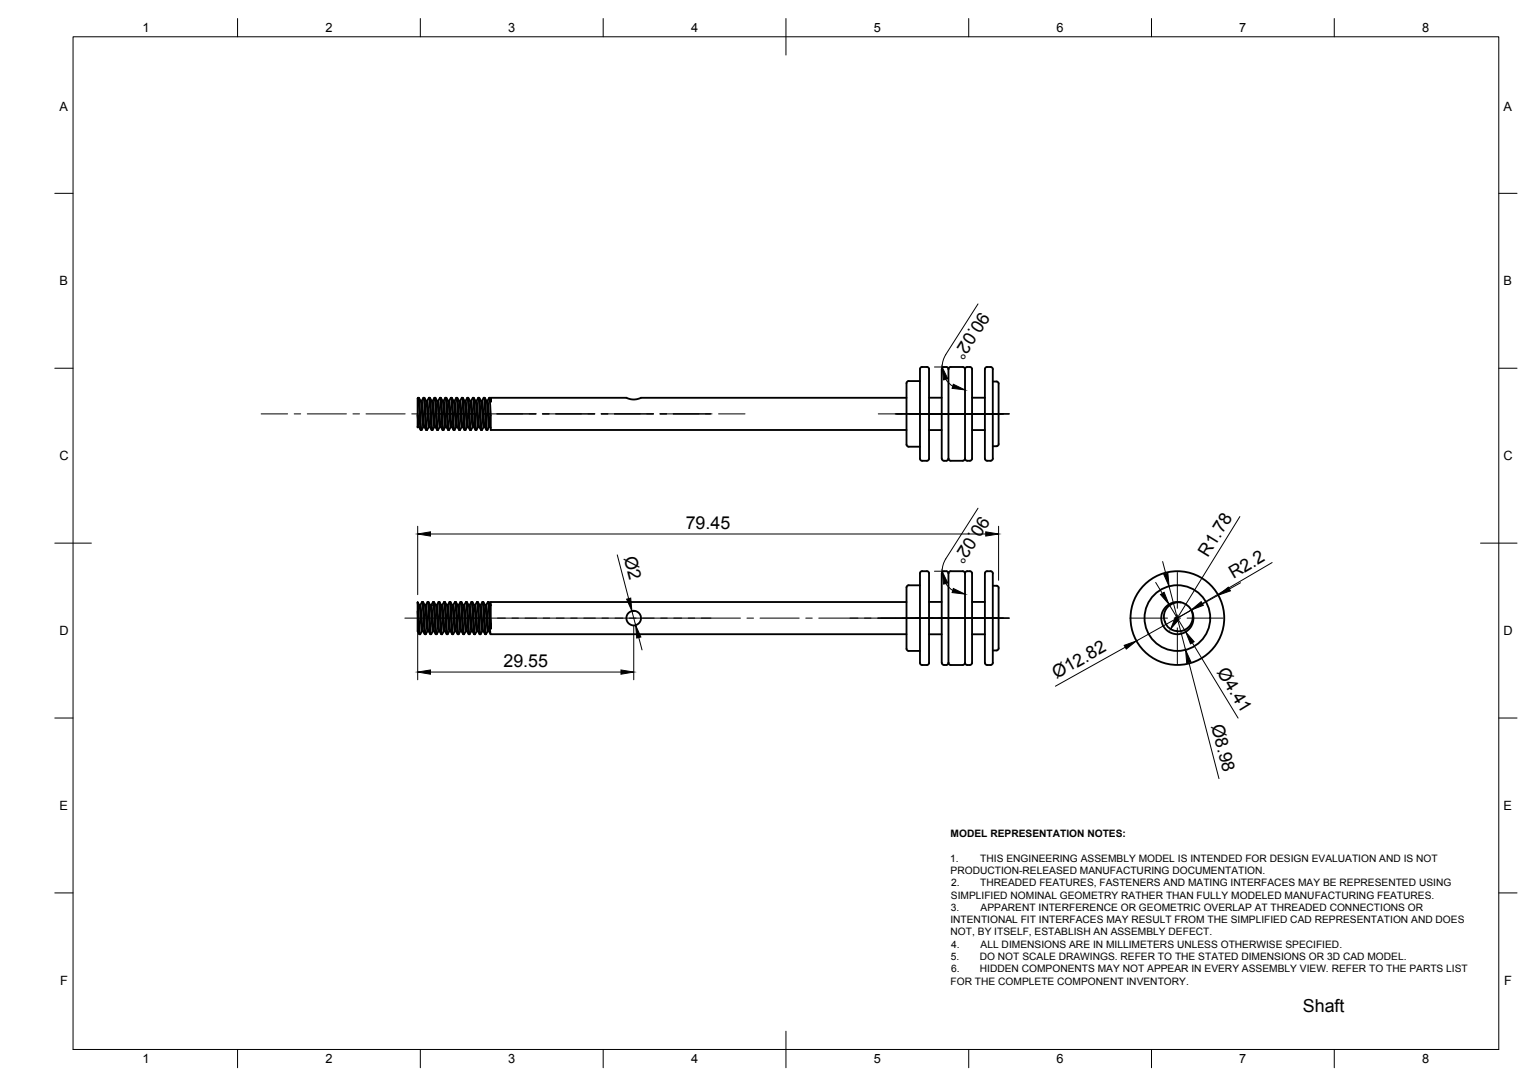
ISO-10303-21;
HEADER;
/* Generated by software containing ST-Developer
 * from STEP Tools, Inc. (www.steptools.com) 
 */

FILE_DESCRIPTION(
/* description */ (''),
/* implementation_level */ '2;1');

FILE_NAME(
/* name */ 'Shaft.step',
/* time_stamp */ '2026-10-06T13:15:55-07:00',
/* author */ (''),
/* organization */ (''),
/* preprocessor_version */ 'ST-DEVELOPER v20.2',
/* originating_system */ 'Autodesk Translation Framework v15.15.0.0',
/* authorisation */ '');

FILE_SCHEMA (('AUTOMOTIVE_DESIGN { 1 0 10303 214 3 1 1 }'));
ENDSEC;

DATA;
#10=MECHANICAL_DESIGN_GEOMETRIC_PRESENTATION_REPRESENTATION('',(#116),#27707);
#55=TOROIDAL_SURFACE('',#4197,6.10845002480549,0.3);
#56=TOROIDAL_SURFACE('',#4203,6.107959450045,0.3);
#57=TOROIDAL_SURFACE('',#4209,4.18902817623056,0.3);
#58=TOROIDAL_SURFACE('',#4216,6.1096023907077,0.3);
#59=TOROIDAL_SURFACE('',#4223,6.10941276264524,0.3);
#60=TOROIDAL_SURFACE('',#4228,6.1087216021292,0.3);
#61=TOROIDAL_SURFACE('',#4236,6.1086273903848,0.3);
#62=TOROIDAL_SURFACE('',#4238,6.10778208446569,0.3);
#63=TOROIDAL_SURFACE('',#4243,6.10767319978801,0.3);
#64=TOROIDAL_SURFACE('',#4248,6.1069775362949,0.3);
#65=TOROIDAL_SURFACE('',#4256,6.10683442041659,0.3);
#66=TOROIDAL_SURFACE('',#4261,4.12329516333974,0.3);
#83=CONICAL_SURFACE('',#4201,6.40820475053297,0.000295609290233083);
#84=CONICAL_SURFACE('',#4220,6.40950758978419,0.000295609290232241);
#85=CONICAL_SURFACE('',#4232,6.40867450936473,0.000295609290232273);
#86=CONICAL_SURFACE('',#4241,6.40772765523458,0.000295609290232245);
#87=CONICAL_SURFACE('',#4252,6.40690599146347,0.000295609290233429);
#96=SHAPE_REPRESENTATION_RELATIONSHIP('SRR','None',#27753,#106);
#106=ADVANCED_BREP_SHAPE_REPRESENTATION('',(#126),#27705);
#116=STYLED_ITEM('',(#27804),#126);
#126=MANIFOLD_SOLID_BREP('Body1',#3842);
#151=FACE_BOUND('',#835,.T.);
#152=FACE_BOUND('',#866,.T.);
#153=FACE_BOUND('',#871,.T.);
#154=FACE_BOUND('',#879,.T.);
#155=FACE_BOUND('',#883,.T.);
#156=FACE_BOUND('',#886,.T.);
#157=FACE_BOUND('',#890,.T.);
#158=FACE_BOUND('',#896,.T.);
#159=FACE_BOUND('',#900,.T.);
#160=FACE_BOUND('',#903,.T.);
#203=PLANE('',#4191);
#204=PLANE('',#4194);
#205=PLANE('',#4205);
#206=PLANE('',#4207);
#207=PLANE('',#4208);
#208=PLANE('',#4215);
#209=PLANE('',#4222);
#210=PLANE('',#4226);
#211=PLANE('',#4234);
#212=PLANE('',#4246);
#213=PLANE('',#4254);
#214=PLANE('',#4259);
#215=PLANE('',#4265);
#291=CIRCLE('',#4158,2.204);
#292=CIRCLE('',#4159,2.204);
#293=CIRCLE('',#4160,2.204);
#294=CIRCLE('',#4174,1.77625);
#295=CIRCLE('',#4188,1.77625);
#296=CIRCLE('',#4190,0.999999999999996);
#297=CIRCLE('',#4193,2.204);
#298=CIRCLE('',#4195,6.107959450045);
#299=CIRCLE('',#4196,6.10778208446569);
#300=CIRCLE('',#4198,6.10845002480549);
#301=CIRCLE('',#4199,0.3);
#302=CIRCLE('',#4200,6.40845001169777);
#303=CIRCLE('',#4202,6.40795943693727);
#304=CIRCLE('',#4204,0.3);
#305=CIRCLE('',#4206,6.1086273903848);
#306=CIRCLE('',#4210,4.18902817623056);
#307=CIRCLE('',#4211,0.3);
#308=CIRCLE('',#4212,4.48902817623056);
#309=CIRCLE('',#4214,4.48902817623056);
#310=CIRCLE('',#4217,6.1096023907077);
#311=CIRCLE('',#4218,0.3);
#312=CIRCLE('',#4219,6.40960237759997);
#313=CIRCLE('',#4221,6.40941274953751);
#314=CIRCLE('',#4224,0.3);
#315=CIRCLE('',#4225,6.10941276264524);
#316=CIRCLE('',#4227,2.21164758166987);
#317=CIRCLE('',#4229,6.1087216021292);
#318=CIRCLE('',#4230,0.3);
#319=CIRCLE('',#4231,6.40872158902147);
#320=CIRCLE('',#4233,6.40862737727707);
#321=CIRCLE('',#4235,2.21164758166987);
#322=CIRCLE('',#4237,0.3);
#323=CIRCLE('',#4239,0.3);
#324=CIRCLE('',#4240,6.40778207135796);
#325=CIRCLE('',#4242,6.40767318668028);
#326=CIRCLE('',#4244,0.3);
#327=CIRCLE('',#4245,6.10767319978801);
#328=CIRCLE('',#4247,2.21164758166987);
#329=CIRCLE('',#4249,6.1069775362949);
#330=CIRCLE('',#4250,0.3);
#331=CIRCLE('',#4251,6.40697752318717);
#332=CIRCLE('',#4253,6.40683440730886);
#333=CIRCLE('',#4255,2.21164758166987);
#334=CIRCLE('',#4257,0.3);
#335=CIRCLE('',#4258,6.10683442041659);
#336=CIRCLE('',#4260,4.42329516333974);
#337=CIRCLE('',#4262,4.42329516333974);
#338=CIRCLE('',#4263,0.3);
#339=CIRCLE('',#4264,4.12329516333974);
#403=CYLINDRICAL_SURFACE('',#4157,2.204);
#404=CYLINDRICAL_SURFACE('',#4161,2.204);
#405=CYLINDRICAL_SURFACE('',#4162,2.204);
#406=CYLINDRICAL_SURFACE('',#4163,2.204);
#407=CYLINDRICAL_SURFACE('',#4164,2.204);
#408=CYLINDRICAL_SURFACE('',#4165,2.204);
#409=CYLINDRICAL_SURFACE('',#4166,2.204);
#410=CYLINDRICAL_SURFACE('',#4167,2.204);
#411=CYLINDRICAL_SURFACE('',#4168,2.204);
#412=CYLINDRICAL_SURFACE('',#4169,2.204);
#413=CYLINDRICAL_SURFACE('',#4170,2.204);
#414=CYLINDRICAL_SURFACE('',#4171,2.204);
#415=CYLINDRICAL_SURFACE('',#4172,2.204);
#416=CYLINDRICAL_SURFACE('',#4173,1.77625);
#417=CYLINDRICAL_SURFACE('',#4175,1.77625);
#418=CYLINDRICAL_SURFACE('',#4176,1.77625);
#419=CYLINDRICAL_SURFACE('',#4177,1.77625);
#420=CYLINDRICAL_SURFACE('',#4178,1.77625);
#421=CYLINDRICAL_SURFACE('',#4179,1.77625);
#422=CYLINDRICAL_SURFACE('',#4180,1.77625);
#423=CYLINDRICAL_SURFACE('',#4181,1.77625);
#424=CYLINDRICAL_SURFACE('',#4182,1.77625);
#425=CYLINDRICAL_SURFACE('',#4183,1.77625);
#426=CYLINDRICAL_SURFACE('',#4184,1.77625);
#427=CYLINDRICAL_SURFACE('',#4185,1.77625);
#428=CYLINDRICAL_SURFACE('',#4186,1.77625);
#429=CYLINDRICAL_SURFACE('',#4187,1.77625);
#430=CYLINDRICAL_SURFACE('',#4189,0.999999999999996);
#431=CYLINDRICAL_SURFACE('',#4192,2.204);
#432=CYLINDRICAL_SURFACE('',#4213,4.48902817623056);
#433=CYLINDRICAL_SURFACE('',#4266,4.42329516333974);
#434=CYLINDRICAL_SURFACE('',#4267,2.21164758166987);
#435=CYLINDRICAL_SURFACE('',#4268,2.21164758166987);
#590=FACE_OUTER_BOUND('',#834,.T.);
#591=FACE_OUTER_BOUND('',#836,.T.);
#592=FACE_OUTER_BOUND('',#837,.T.);
#593=FACE_OUTER_BOUND('',#838,.T.);
#594=FACE_OUTER_BOUND('',#839,.T.);
#595=FACE_OUTER_BOUND('',#840,.T.);
#596=FACE_OUTER_BOUND('',#841,.T.);
#597=FACE_OUTER_BOUND('',#842,.T.);
#598=FACE_OUTER_BOUND('',#843,.T.);
#599=FACE_OUTER_BOUND('',#844,.T.);
#600=FACE_OUTER_BOUND('',#845,.T.);
#601=FACE_OUTER_BOUND('',#846,.T.);
#602=FACE_OUTER_BOUND('',#847,.T.);
#603=FACE_OUTER_BOUND('',#848,.T.);
#604=FACE_OUTER_BOUND('',#849,.T.);
#605=FACE_OUTER_BOUND('',#850,.T.);
#606=FACE_OUTER_BOUND('',#851,.T.);
#607=FACE_OUTER_BOUND('',#852,.T.);
#608=FACE_OUTER_BOUND('',#853,.T.);
#609=FACE_OUTER_BOUND('',#854,.T.);
#610=FACE_OUTER_BOUND('',#855,.T.);
#611=FACE_OUTER_BOUND('',#856,.T.);
#612=FACE_OUTER_BOUND('',#857,.T.);
#613=FACE_OUTER_BOUND('',#858,.T.);
#614=FACE_OUTER_BOUND('',#859,.T.);
#615=FACE_OUTER_BOUND('',#860,.T.);
#616=FACE_OUTER_BOUND('',#861,.T.);
#617=FACE_OUTER_BOUND('',#862,.T.);
#618=FACE_OUTER_BOUND('',#863,.T.);
#619=FACE_OUTER_BOUND('',#864,.T.);
#620=FACE_OUTER_BOUND('',#865,.T.);
#621=FACE_OUTER_BOUND('',#867,.T.);
#622=FACE_OUTER_BOUND('',#868,.T.);
#623=FACE_OUTER_BOUND('',#869,.T.);
#624=FACE_OUTER_BOUND('',#870,.T.);
#625=FACE_OUTER_BOUND('',#872,.T.);
#626=FACE_OUTER_BOUND('',#873,.T.);
#627=FACE_OUTER_BOUND('',#874,.T.);
#628=FACE_OUTER_BOUND('',#875,.T.);
#629=FACE_OUTER_BOUND('',#876,.T.);
#630=FACE_OUTER_BOUND('',#877,.T.);
#631=FACE_OUTER_BOUND('',#878,.T.);
#632=FACE_OUTER_BOUND('',#880,.T.);
#633=FACE_OUTER_BOUND('',#881,.T.);
#634=FACE_OUTER_BOUND('',#882,.T.);
#635=FACE_OUTER_BOUND('',#884,.T.);
#636=FACE_OUTER_BOUND('',#885,.T.);
#637=FACE_OUTER_BOUND('',#887,.T.);
#638=FACE_OUTER_BOUND('',#888,.T.);
#639=FACE_OUTER_BOUND('',#889,.T.);
#640=FACE_OUTER_BOUND('',#891,.T.);
#641=FACE_OUTER_BOUND('',#892,.T.);
#642=FACE_OUTER_BOUND('',#893,.T.);
#643=FACE_OUTER_BOUND('',#894,.T.);
#644=FACE_OUTER_BOUND('',#895,.T.);
#645=FACE_OUTER_BOUND('',#897,.T.);
#646=FACE_OUTER_BOUND('',#898,.T.);
#647=FACE_OUTER_BOUND('',#899,.T.);
#648=FACE_OUTER_BOUND('',#901,.T.);
#649=FACE_OUTER_BOUND('',#902,.T.);
#650=FACE_OUTER_BOUND('',#904,.T.);
#651=FACE_OUTER_BOUND('',#905,.T.);
#652=FACE_OUTER_BOUND('',#906,.T.);
#653=FACE_OUTER_BOUND('',#907,.T.);
#654=FACE_OUTER_BOUND('',#908,.T.);
#834=EDGE_LOOP('',(#3233,#3234,#3235,#3236,#3237,#3238,#3239,#3240,#3241,
#3242));
#835=EDGE_LOOP('',(#3243,#3244));
#836=EDGE_LOOP('',(#3245,#3246,#3247,#3248));
#837=EDGE_LOOP('',(#3249,#3250,#3251,#3252));
#838=EDGE_LOOP('',(#3253,#3254,#3255,#3256,#3257,#3258));
#839=EDGE_LOOP('',(#3259,#3260,#3261,#3262,#3263,#3264));
#840=EDGE_LOOP('',(#3265,#3266,#3267,#3268));
#841=EDGE_LOOP('',(#3269,#3270,#3271,#3272,#3273,#3274));
#842=EDGE_LOOP('',(#3275,#3276,#3277,#3278));
#843=EDGE_LOOP('',(#3279,#3280,#3281,#3282));
#844=EDGE_LOOP('',(#3283,#3284,#3285,#3286,#3287,#3288));
#845=EDGE_LOOP('',(#3289,#3290,#3291,#3292,#3293,#3294));
#846=EDGE_LOOP('',(#3295,#3296,#3297,#3298));
#847=EDGE_LOOP('',(#3299,#3300,#3301,#3302));
#848=EDGE_LOOP('',(#3303,#3304,#3305,#3306));
#849=EDGE_LOOP('',(#3307,#3308,#3309,#3310));
#850=EDGE_LOOP('',(#3311,#3312,#3313,#3314,#3315));
#851=EDGE_LOOP('',(#3316,#3317,#3318,#3319));
#852=EDGE_LOOP('',(#3320,#3321,#3322,#3323));
#853=EDGE_LOOP('',(#3324,#3325,#3326,#3327));
#854=EDGE_LOOP('',(#3328,#3329,#3330,#3331));
#855=EDGE_LOOP('',(#3332,#3333,#3334,#3335));
#856=EDGE_LOOP('',(#3336,#3337,#3338,#3339));
#857=EDGE_LOOP('',(#3340,#3341,#3342,#3343));
#858=EDGE_LOOP('',(#3344,#3345,#3346,#3347));
#859=EDGE_LOOP('',(#3348,#3349,#3350,#3351,#3352));
#860=EDGE_LOOP('',(#3353,#3354,#3355,#3356));
#861=EDGE_LOOP('',(#3357,#3358,#3359,#3360,#3361));
#862=EDGE_LOOP('',(#3362,#3363,#3364,#3365,#3366));
#863=EDGE_LOOP('',(#3367));
#864=EDGE_LOOP('',(#3368,#3369,#3370,#3371));
#865=EDGE_LOOP('',(#3372));
#866=EDGE_LOOP('',(#3373));
#867=EDGE_LOOP('',(#3374,#3375,#3376,#3377));
#868=EDGE_LOOP('',(#3378,#3379,#3380,#3381));
#869=EDGE_LOOP('',(#3382,#3383,#3384,#3385));
#870=EDGE_LOOP('',(#3386));
#871=EDGE_LOOP('',(#3387));
#872=EDGE_LOOP('',(#3388,#3389,#3390,#3391,#3392,#3393,#3394,#3395,#3396,
#3397,#3398,#3399,#3400,#3401,#3402,#3403,#3404,#3405,#3406,#3407,#3408,
#3409,#3410,#3411,#3412,#3413,#3414,#3415,#3416,#3417,#3418,#3419,#3420,
#3421,#3422,#3423,#3424,#3425));
#873=EDGE_LOOP('',(#3426,#3427,#3428,#3429,#3430,#3431));
#874=EDGE_LOOP('',(#3432,#3433,#3434,#3435,#3436,#3437,#3438,#3439,#3440,
#3441,#3442,#3443,#3444,#3445,#3446,#3447,#3448,#3449,#3450,#3451,#3452,
#3453,#3454,#3455,#3456,#3457,#3458,#3459,#3460,#3461,#3462,#3463,#3464,
#3465,#3466,#3467,#3468,#3469,#3470));
#875=EDGE_LOOP('',(#3471,#3472,#3473,#3474,#3475));
#876=EDGE_LOOP('',(#3476,#3477,#3478,#3479));
#877=EDGE_LOOP('',(#3480,#3481,#3482,#3483));
#878=EDGE_LOOP('',(#3484));
#879=EDGE_LOOP('',(#3485));
#880=EDGE_LOOP('',(#3486,#3487,#3488,#3489));
#881=EDGE_LOOP('',(#3490,#3491,#3492,#3493));
#882=EDGE_LOOP('',(#3494));
#883=EDGE_LOOP('',(#3495));
#884=EDGE_LOOP('',(#3496,#3497,#3498,#3499));
#885=EDGE_LOOP('',(#3500));
#886=EDGE_LOOP('',(#3501));
#887=EDGE_LOOP('',(#3502,#3503,#3504,#3505));
#888=EDGE_LOOP('',(#3506,#3507,#3508,#3509));
#889=EDGE_LOOP('',(#3510));
#890=EDGE_LOOP('',(#3511));
#891=EDGE_LOOP('',(#3512,#3513,#3514,#3515));
#892=EDGE_LOOP('',(#3516,#3517,#3518,#3519));
#893=EDGE_LOOP('',(#3520,#3521,#3522,#3523));
#894=EDGE_LOOP('',(#3524,#3525,#3526,#3527));
#895=EDGE_LOOP('',(#3528));
#896=EDGE_LOOP('',(#3529));
#897=EDGE_LOOP('',(#3530,#3531,#3532,#3533));
#898=EDGE_LOOP('',(#3534,#3535,#3536,#3537));
#899=EDGE_LOOP('',(#3538));
#900=EDGE_LOOP('',(#3539));
#901=EDGE_LOOP('',(#3540,#3541,#3542,#3543));
#902=EDGE_LOOP('',(#3544));
#903=EDGE_LOOP('',(#3545));
#904=EDGE_LOOP('',(#3546,#3547,#3548,#3549));
#905=EDGE_LOOP('',(#3550));
#906=EDGE_LOOP('',(#3551,#3552,#3553,#3554));
#907=EDGE_LOOP('',(#3555,#3556,#3557,#3558));
#908=EDGE_LOOP('',(#3559,#3560,#3561,#3562));
#1052=LINE('',#15722,#1228);
#1053=LINE('',#15863,#1229);
#1054=LINE('',#15978,#1230);
#1055=LINE('',#16402,#1231);
#1056=LINE('',#16802,#1232);
#1057=LINE('',#17236,#1233);
#1058=LINE('',#17648,#1234);
#1059=LINE('',#18052,#1235);
#1060=LINE('',#18470,#1236);
#1061=LINE('',#18872,#1237);
#1062=LINE('',#19296,#1238);
#1063=LINE('',#19720,#1239);
#1064=LINE('',#20146,#1240);
#1065=LINE('',#20554,#1241);
#1066=LINE('',#20960,#1242);
#1067=LINE('',#21259,#1243);
#1068=LINE('',#21635,#1244);
#1069=LINE('',#22036,#1245);
#1070=LINE('',#22418,#1246);
#1071=LINE('',#22804,#1247);
#1072=LINE('',#23196,#1248);
#1073=LINE('',#23578,#1249);
#1074=LINE('',#23968,#1250);
#1075=LINE('',#24346,#1251);
#1076=LINE('',#24732,#1252);
#1077=LINE('',#25116,#1253);
#1078=LINE('',#25507,#1254);
#1079=LINE('',#26142,#1255);
#1080=LINE('',#26496,#1256);
#1081=LINE('',#27575,#1257);
#1082=LINE('',#27586,#1258);
#1083=LINE('',#27604,#1259);
#1084=LINE('',#27617,#1260);
#1085=LINE('',#27634,#1261);
#1086=LINE('',#27654,#1262);
#1087=LINE('',#27656,#1263);
#1088=LINE('',#27658,#1264);
#1228=VECTOR('',#4831,2.204);
#1229=VECTOR('',#4834,2.204);
#1230=VECTOR('',#4841,2.204);
#1231=VECTOR('',#4844,2.204);
#1232=VECTOR('',#4847,2.204);
#1233=VECTOR('',#4850,2.204);
#1234=VECTOR('',#4853,2.204);
#1235=VECTOR('',#4856,2.204);
#1236=VECTOR('',#4859,2.204);
#1237=VECTOR('',#4862,2.204);
#1238=VECTOR('',#4865,2.204);
#1239=VECTOR('',#4868,2.204);
#1240=VECTOR('',#4871,2.204);
#1241=VECTOR('',#4874,2.204);
#1242=VECTOR('',#4877,1.77625);
#1243=VECTOR('',#4882,1.77625);
#1244=VECTOR('',#4885,1.77625);
#1245=VECTOR('',#4888,1.77625);
#1246=VECTOR('',#4891,1.77625);
#1247=VECTOR('',#4894,1.77625);
#1248=VECTOR('',#4897,1.77625);
#1249=VECTOR('',#4900,1.77625);
#1250=VECTOR('',#4903,1.77625);
#1251=VECTOR('',#4906,1.77625);
#1252=VECTOR('',#4909,1.77625);
#1253=VECTOR('',#4912,1.77625);
#1254=VECTOR('',#4915,1.77625);
#1255=VECTOR('',#4924,0.999999999999996);
#1256=VECTOR('',#4947,6.40820475053297);
#1257=VECTOR('',#4972,4.48902817623056);
#1258=VECTOR('',#4987,6.40950758978419);
#1259=VECTOR('',#5012,6.40867450936473);
#1260=VECTOR('',#5031,6.40772765523458);
#1261=VECTOR('',#5054,6.40690599146347);
#1262=VECTOR('',#5083,4.42329516333974);
#1263=VECTOR('',#5086,2.21164758166987);
#1264=VECTOR('',#5089,2.21164758166987);
#1442=B_SPLINE_CURVE_WITH_KNOTS('',3,(#15724,#15725,#15726,#15727),
 .UNSPECIFIED.,.F.,.F.,(4,4),(2.77524983164141,2.7754356884636),
 .UNSPECIFIED.);
#1443=B_SPLINE_CURVE_WITH_KNOTS('',3,(#15729,#15730,#15731,#15732,#15733,
#15734,#15735,#15736,#15737,#15738,#15739,#15740,#15741,#15742,#15743,#15744,
#15745,#15746,#15747,#15748,#15749,#15750,#15751,#15752,#15753,#15754,#15755,
#15756,#15757,#15758,#15759,#15760,#15761,#15762,#15763,#15764,#15765,#15766,
#15767,#15768,#15769,#15770,#15771,#15772,#15773,#15774,#15775,#15776,#15777,
#15778,#15779,#15780,#15781,#15782,#15783,#15784,#15785,#15786,#15787,#15788,
#15789,#15790,#15791,#15792,#15793,#15794,#15795,#15796,#15797,#15798,#15799,
#15800,#15801,#15802,#15803,#15804,#15805,#15806,#15807,#15808,#15809,#15810,
#15811,#15812,#15813,#15814,#15815,#15816,#15817,#15818,#15819,#15820,#15821,
#15822,#15823,#15824,#15825,#15826,#15827,#15828,#15829,#15830,#15831,#15832,
#15833,#15834,#15835,#15836,#15837,#15838,#15839,#15840,#15841,#15842,#15843,
#15844,#15845,#15846,#15847,#15848,#15849,#15850,#15851,#15852),
 .UNSPECIFIED.,.F.,.F.,(4,3,3,3,3,3,3,3,3,3,3,3,3,3,3,3,3,3,3,3,3,3,3,3,
3,3,3,3,3,3,3,3,3,3,3,3,3,3,3,3,3,4),(-5.2891562906822,-5.18360776201043,
-5.16592202403009,-5.06502794865638,-5.0409071101405,-4.991013367524,-4.99097352154249,
-4.89791297254004,-4.8887207823386,-4.78661873310371,-4.68463617498642,
-4.58271830049947,-4.48083193862712,-4.37894396049634,-4.27695022114797,
-4.17490252616154,-4.07267004030852,-3.9928178800891,-3.99277881723399,
-3.89952340746646,-3.89022667007414,-3.78782539108402,-3.68554527959923,
-3.58333102513057,-3.48114986928111,-3.37896909715953,-3.27668767666928,
-3.17435468887112,-3.0718440432757,-2.9946218545813,-2.99458411292549,-2.90179614365268,
-2.89325038855348,-2.79021171641803,-2.68914057287426,-2.58812832611143,
-2.48714069765389,-2.38259077610789,-2.28148996903811,-2.175215490254,-2.07915882623621,
-2.06894888197497),.UNSPECIFIED.);
#1444=B_SPLINE_CURVE_WITH_KNOTS('',3,(#15854,#15855,#15856,#15857,#15858,
#15859),.UNSPECIFIED.,.F.,.F.,(4,2,4),(0.000102523276221914,0.00211374109474727,
0.00412550342438516),.UNSPECIFIED.);
#1445=B_SPLINE_CURVE_WITH_KNOTS('',3,(#15867,#15868,#15869,#15870,#15871,
#15872,#15873,#15874,#15875,#15876,#15877,#15878,#15879,#15880,#15881,#15882,
#15883,#15884,#15885,#15886,#15887,#15888,#15889,#15890,#15891,#15892,#15893,
#15894,#15895,#15896,#15897,#15898,#15899,#15900,#15901,#15902,#15903,#15904,
#15905,#15906,#15907,#15908,#15909,#15910,#15911,#15912,#15913,#15914,#15915,
#15916,#15917,#15918,#15919,#15920,#15921,#15922,#15923,#15924,#15925,#15926,
#15927,#15928,#15929,#15930,#15931,#15932,#15933,#15934,#15935,#15936),
 .UNSPECIFIED.,.F.,.F.,(4,3,3,3,3,3,3,3,3,3,3,3,3,3,3,3,3,3,3,3,3,3,3,4),
(0.,0.104661171317195,0.209255039882458,0.313836025669164,0.418414672909222,
0.523017976486558,0.627672951902333,0.732486530385716,0.837386576506837,
0.942488701205836,0.998194704308485,1.09966450843524,1.20096987785232,1.30213869551464,
1.40323263958923,1.50428592829615,1.60533272568538,1.70647828415392,1.80767242300264,
1.9090522202859,1.99638940861699,2.12019797963207,2.24242280953419,2.31370279205594),
 .UNSPECIFIED.);
#1446=B_SPLINE_CURVE_WITH_KNOTS('',3,(#15939,#15940,#15941,#15942,#15943,
#15944,#15945,#15946,#15947,#15948),.UNSPECIFIED.,.F.,.F.,(4,2,2,2,4),(0.,
0.038320218022911,0.076640436045822,0.114893233564743,0.153146031083664),
 .UNSPECIFIED.);
#1447=B_SPLINE_CURVE_WITH_KNOTS('',3,(#15949,#15950,#15951,#15952,#15953,
#15954,#15955,#15956,#15957,#15958,#15959,#15960,#15961,#15962,#15963,#15964,
#15965,#15966,#15967,#15968,#15969,#15970,#15971,#15972,#15973,#15974),
 .UNSPECIFIED.,.F.,.F.,(4,2,2,2,2,2,2,2,2,2,2,2,4),(0.153146031083664,0.191398828602585,
0.229651626121507,0.267971844144418,0.306292062167329,0.344612280190239,
0.382932498213151,0.421185295732072,0.459438093250993,0.497690890769914,
0.535943688288835,0.574263906311746,0.612584124334657),.UNSPECIFIED.);
#1448=B_SPLINE_CURVE_WITH_KNOTS('',3,(#15979,#15980,#15981,#15982,#15983,
#15984,#15985,#15986,#15987,#15988,#15989,#15990,#15991,#15992,#15993,#15994,
#15995,#15996,#15997,#15998,#15999,#16000,#16001,#16002,#16003,#16004,#16005,
#16006,#16007,#16008,#16009,#16010,#16011,#16012,#16013,#16014,#16015,#16016,
#16017,#16018,#16019,#16020,#16021,#16022,#16023,#16024,#16025,#16026,#16027,
#16028,#16029,#16030,#16031,#16032,#16033,#16034,#16035,#16036,#16037,#16038,
#16039,#16040,#16041,#16042,#16043,#16044,#16045,#16046,#16047,#16048,#16049,
#16050,#16051,#16052,#16053,#16054,#16055,#16056,#16057,#16058,#16059,#16060,
#16061,#16062,#16063,#16064,#16065,#16066,#16067,#16068,#16069,#16070,#16071,
#16072,#16073,#16074,#16075,#16076,#16077,#16078,#16079,#16080,#16081,#16082,
#16083,#16084,#16085,#16086,#16087,#16088,#16089,#16090,#16091,#16092,#16093,
#16094,#16095,#16096,#16097,#16098,#16099,#16100,#16101,#16102,#16103,#16104,
#16105,#16106,#16107,#16108,#16109,#16110,#16111,#16112,#16113,#16114,#16115,
#16116,#16117,#16118,#16119,#16120,#16121,#16122,#16123,#16124,#16125,#16126,
#16127,#16128,#16129,#16130,#16131,#16132,#16133,#16134,#16135,#16136,#16137,
#16138,#16139,#16140,#16141,#16142,#16143,#16144,#16145,#16146,#16147,#16148,
#16149,#16150,#16151,#16152,#16153,#16154,#16155,#16156,#16157,#16158,#16159,
#16160,#16161,#16162,#16163,#16164,#16165,#16166,#16167,#16168,#16169,#16170,
#16171,#16172,#16173,#16174,#16175,#16176,#16177,#16178,#16179,#16180,#16181,
#16182,#16183,#16184,#16185,#16186,#16187,#16188),.UNSPECIFIED.,.F.,.F.,
(4,2,2,2,2,2,2,2,2,2,2,2,2,2,2,2,2,2,2,2,2,2,2,2,2,2,2,2,2,2,2,2,2,2,2,
2,2,2,2,2,2,2,2,2,2,2,2,2,2,2,2,2,2,2,2,2,2,2,2,2,2,2,2,2,2,2,2,2,2,2,2,
2,2,2,2,2,2,2,2,2,2,2,2,2,2,2,2,2,2,2,2,2,2,2,2,2,2,2,2,2,2,2,2,2,4),(1.38781753873472,
1.39967307302691,1.40445914459052,1.40800356043637,1.41188756410644,1.41730276084749,
1.43084058397849,1.45101472565709,1.49357630988404,1.51136965632633,1.51559250277158,
1.51800787610396,1.52016188469643,1.52312080974288,1.5301823492393,1.54050794057009,
1.57534931570515,1.61237651259864,1.62165050138927,1.62639272592381,1.63018049920159,
1.63449363382543,1.64197198759118,1.68827555501049,1.72888793290298,1.73432736841164,
1.73703730628583,1.73921644847553,1.74151957718618,1.74523007548616,1.75831706971953,
1.78424581384169,1.83324275090273,1.84148685272035,1.84640241907379,1.85021948989542,
1.85438844787025,1.86119275138631,1.88833036670492,1.91645593292796,1.92484579996025,
1.95163644192558,1.95615739428983,1.95866430015579,1.96080002902903,1.96360332353323,
1.96976113670856,1.9974795461816,2.04742308357646,2.06052975701291,2.06602236058527,
2.06988229338644,2.07387199386493,2.07982730521795,2.09743024198081,2.12751039769845,
2.16992979139149,2.17582030821991,2.17857371361266,2.18070399666525,2.18324296864977,
2.18805348663228,2.19427456685343,2.20908608355818,2.2374776975812,2.27704904795642,
2.2843724340021,2.28869178348119,2.29243957129668,2.29714655932481,2.30656346429877,
2.31888721665889,2.35133919106459,2.39005584916645,2.39615404619614,2.39891498336828,
2.40104980462189,2.40355070418799,2.40817287159305,2.44279419766279,2.49508899561064,
2.5030484745972,2.50793628306202,2.51174021856224,2.51596804476606,2.52304226080094,
2.55492153642243,2.59780879562011,2.6137871040324,2.61788971530304,2.62028035171697,
2.62244948790057,2.62547794183238,2.63293492193362,2.64405309222125,2.66962673554813,
2.70117621828321,2.71983292544932,2.72609634153291,2.73015451659309,2.73402583299897,
2.73784961158552,2.74298847368029,2.75426624309546,2.77524983164141),
 .UNSPECIFIED.);
#1449=B_SPLINE_CURVE_WITH_KNOTS('',3,(#16189,#16190,#16191,#16192,#16193,
#16194,#16195,#16196,#16197,#16198,#16199,#16200,#16201,#16202,#16203,#16204,
#16205,#16206,#16207,#16208,#16209,#16210,#16211,#16212,#16213,#16214,#16215,
#16216,#16217,#16218,#16219,#16220,#16221,#16222,#16223,#16224,#16225,#16226,
#16227,#16228,#16229,#16230,#16231,#16232,#16233,#16234,#16235,#16236,#16237,
#16238,#16239,#16240,#16241,#16242,#16243,#16244,#16245,#16246,#16247,#16248,
#16249,#16250,#16251,#16252,#16253,#16254,#16255,#16256,#16257,#16258,#16259,
#16260,#16261,#16262,#16263,#16264,#16265,#16266,#16267,#16268,#16269,#16270,
#16271,#16272,#16273,#16274,#16275,#16276,#16277,#16278,#16279,#16280,#16281,
#16282,#16283,#16284,#16285,#16286,#16287,#16288,#16289,#16290,#16291,#16292,
#16293,#16294,#16295,#16296,#16297,#16298,#16299,#16300,#16301,#16302,#16303,
#16304,#16305,#16306,#16307,#16308,#16309,#16310,#16311,#16312,#16313,#16314,
#16315,#16316,#16317,#16318,#16319,#16320,#16321,#16322,#16323,#16324,#16325,
#16326,#16327,#16328,#16329,#16330,#16331,#16332,#16333,#16334,#16335,#16336,
#16337,#16338,#16339,#16340,#16341,#16342,#16343,#16344,#16345,#16346,#16347,
#16348,#16349,#16350,#16351,#16352,#16353,#16354,#16355,#16356,#16357,#16358,
#16359,#16360,#16361,#16362,#16363,#16364,#16365,#16366,#16367,#16368,#16369,
#16370,#16371,#16372,#16373,#16374,#16375,#16376,#16377,#16378,#16379,#16380,
#16381,#16382,#16383,#16384,#16385,#16386,#16387,#16388,#16389,#16390,#16391,
#16392,#16393,#16394,#16395,#16396,#16397,#16398),.UNSPECIFIED.,.F.,.F.,
(4,2,2,2,2,2,2,2,2,2,2,2,2,2,2,2,2,2,2,2,2,2,2,2,2,2,2,2,2,2,2,2,2,2,2,
2,2,2,2,2,2,2,2,2,2,2,2,2,2,2,2,2,2,2,2,2,2,2,2,2,2,2,2,2,2,2,2,2,2,2,2,
2,2,2,2,2,2,2,2,2,2,2,2,2,2,2,2,2,2,2,2,2,2,2,2,2,2,2,2,2,2,2,2,2,4),(0.000677522696600237,
0.0305089258241106,0.0357217105988039,0.0396135137556909,0.0435607528904782,
0.0477204696182164,0.0541915833973012,0.0741059967373185,0.115440097777174,
0.134317184493834,0.145106172757179,0.14864706152995,0.150963559598939,
0.153001420155386,0.155815446427006,0.163035034986156,0.217821138578187,
0.238208395197482,0.251873813278667,0.257357570144765,0.26129934021213,
0.26538551201792,0.271602298038433,0.289353198948155,0.339589261144455,
0.361984375015146,0.367591576073439,0.370311762371205,0.372252757395784,
0.374772116565687,0.379314809039923,0.406404733718979,0.414432682325065,
0.443038327387056,0.460786979930571,0.473151978164989,0.478396583079974,
0.482262594137674,0.486356375416247,0.492760354432907,0.51259909284976,
0.556547787118553,0.582188012129803,0.588138338702213,0.590907459740892,
0.592847503273448,0.595324546479347,0.599646787124584,0.619687590510394,
0.660066375923141,0.680065489411854,0.693550325746206,0.698995403707921,
0.702919464612365,0.706513885714489,0.711389222317492,0.723711801320998,
0.774193276476291,0.802031745603604,0.808230933663737,0.81106284263699,
0.813204901215941,0.815740344409894,0.820315956534282,0.848389345799933,
0.876342856806042,0.909948384155844,0.917146197055969,0.921427871307066,
0.9252687321384,0.930189007400477,0.938172509254794,0.999164983852803,1.01692011627422,
1.02727200361296,1.03071451736817,1.03297461344143,1.03498700860256,1.03776741267351,
1.04344525041317,1.07678153395365,1.10750510753919,1.13160484949986,1.1382267514405,
1.14238168193455,1.14625250349466,1.15133390112501,1.16295108822414,1.2146743273094,
1.24296511256131,1.24920253029659,1.25203487369017,1.25419112323307,1.2567231961712,
1.26128999367794,1.28892807428539,1.29537580787022,1.32175712996296,1.34142706453204,
1.35474982493395,1.36016555562901,1.36408011350876,1.36767367219295,1.37350241506738,
1.38838504316647),.UNSPECIFIED.);
#1450=B_SPLINE_CURVE_WITH_KNOTS('',3,(#16403,#16404,#16405,#16406,#16407,
#16408,#16409,#16410,#16411,#16412,#16413,#16414,#16415,#16416,#16417,#16418,
#16419,#16420,#16421,#16422,#16423,#16424,#16425,#16426,#16427,#16428,#16429,
#16430,#16431,#16432,#16433,#16434,#16435,#16436,#16437,#16438,#16439,#16440,
#16441,#16442,#16443,#16444,#16445,#16446,#16447,#16448,#16449,#16450,#16451,
#16452,#16453,#16454,#16455,#16456,#16457,#16458,#16459,#16460,#16461,#16462,
#16463,#16464,#16465,#16466,#16467,#16468,#16469,#16470,#16471,#16472,#16473,
#16474,#16475,#16476,#16477,#16478,#16479,#16480,#16481,#16482,#16483,#16484,
#16485,#16486,#16487,#16488,#16489,#16490,#16491,#16492,#16493,#16494,#16495,
#16496,#16497,#16498,#16499,#16500,#16501,#16502,#16503,#16504,#16505,#16506,
#16507,#16508,#16509,#16510,#16511,#16512,#16513,#16514,#16515,#16516,#16517,
#16518,#16519,#16520,#16521,#16522,#16523,#16524,#16525,#16526,#16527,#16528,
#16529,#16530,#16531,#16532,#16533,#16534,#16535,#16536,#16537,#16538,#16539,
#16540,#16541,#16542,#16543,#16544,#16545,#16546,#16547,#16548,#16549,#16550,
#16551,#16552,#16553,#16554,#16555,#16556,#16557,#16558,#16559,#16560,#16561,
#16562,#16563,#16564,#16565,#16566,#16567,#16568,#16569,#16570,#16571,#16572,
#16573,#16574,#16575,#16576,#16577,#16578,#16579,#16580,#16581,#16582,#16583,
#16584,#16585,#16586,#16587,#16588,#16589,#16590,#16591,#16592,#16593,#16594,
#16595,#16596,#16597,#16598),.UNSPECIFIED.,.F.,.F.,(4,2,2,2,2,2,2,2,2,2,
2,2,2,2,2,2,2,2,2,2,2,2,2,2,2,2,2,2,2,2,2,2,2,2,2,2,2,2,2,2,2,2,2,2,2,2,
2,2,2,2,2,2,2,2,2,2,2,2,2,2,2,2,2,2,2,2,2,2,2,2,2,2,2,2,2,2,2,2,2,2,2,2,
2,2,2,2,2,2,2,2,2,2,2,2,2,2,2,4),(0.00029246168118835,0.0328585636678094,
0.0667058328462643,0.0778435259812811,0.0828696078886542,0.0866900014310973,
0.0908461587794147,0.097592177913589,0.121093785472563,0.162881838567066,
0.180219822071848,0.190388972658726,0.193788250972792,0.196023740153427,
0.198017167485471,0.200771856106451,0.206396616707088,0.238925364174105,
0.266963907016703,0.294244321785116,0.301057788663898,0.305228435652312,
0.309044486884806,0.313955159749232,0.32218284537282,0.37135389164148,0.408175613816101,
0.412996223661644,0.415538634251756,0.417669540176693,0.420421537274337,
0.426304777495165,0.468914542634666,0.513239590782438,0.520844568367973,
0.525184629927034,0.528969383857968,0.533672976813764,0.542760084971374,
0.590969748200195,0.628864181011441,0.63355354838131,0.636068557916207,
0.638202427997394,0.640945550577899,0.646939191710579,0.687873371930506,
0.733784327768257,0.741346096652906,0.745676995844228,0.749462733365603,
0.75417927556698,0.763328775599775,0.810387242799095,0.837579976993194,
0.851030621355834,0.85477432184903,0.857084664002877,0.859259266550924,
0.861951867948976,0.868744858537939,0.912920490817548,0.940791392600704,
0.957582742793873,0.963439773532905,0.967408607838282,0.971282412503524,
0.976854716010281,0.990459250029259,1.03990459175393,1.06745386194676,1.0735937358375,
1.07639297618157,1.07852766872987,1.08103585188433,1.08556365529159,1.11268366089787,
1.11969753011607,1.1461997886862,1.16583340621934,1.17911405711989,1.18449016762945,
1.18836697719528,1.1919190330671,1.19766366486624,1.21233214987857,1.26072984825734,
1.28791979545175,1.29402325910311,1.29681596339525,1.29895021111714,1.30146329140139,
1.30601243315762,1.33451743269651,1.34130110590104,1.37019173079264,1.38769992508917,
1.38781753873472),.UNSPECIFIED.);
#1451=B_SPLINE_CURVE_WITH_KNOTS('',3,(#16599,#16600,#16601,#16602,#16603,
#16604,#16605,#16606,#16607,#16608,#16609,#16610,#16611,#16612,#16613,#16614,
#16615,#16616,#16617,#16618,#16619,#16620,#16621,#16622,#16623,#16624,#16625,
#16626,#16627,#16628,#16629,#16630,#16631,#16632,#16633,#16634,#16635,#16636,
#16637,#16638,#16639,#16640,#16641,#16642,#16643,#16644,#16645,#16646,#16647,
#16648,#16649,#16650,#16651,#16652,#16653,#16654,#16655,#16656,#16657,#16658,
#16659,#16660,#16661,#16662,#16663,#16664,#16665,#16666,#16667,#16668,#16669,
#16670,#16671,#16672,#16673,#16674,#16675,#16676,#16677,#16678,#16679,#16680,
#16681,#16682,#16683,#16684,#16685,#16686,#16687,#16688,#16689,#16690,#16691,
#16692,#16693,#16694,#16695,#16696,#16697,#16698,#16699,#16700,#16701,#16702,
#16703,#16704,#16705,#16706,#16707,#16708,#16709,#16710,#16711,#16712,#16713,
#16714,#16715,#16716,#16717,#16718,#16719,#16720,#16721,#16722,#16723,#16724,
#16725,#16726,#16727,#16728,#16729,#16730,#16731,#16732,#16733,#16734,#16735,
#16736,#16737,#16738,#16739,#16740,#16741,#16742,#16743,#16744,#16745,#16746,
#16747,#16748,#16749,#16750,#16751,#16752,#16753,#16754,#16755,#16756,#16757,
#16758,#16759,#16760,#16761,#16762,#16763,#16764,#16765,#16766,#16767,#16768,
#16769,#16770,#16771,#16772,#16773,#16774,#16775,#16776,#16777,#16778,#16779,
#16780,#16781,#16782,#16783,#16784,#16785,#16786,#16787,#16788,#16789,#16790,
#16791,#16792,#16793,#16794,#16795,#16796,#16797,#16798),.UNSPECIFIED.,
 .F.,.F.,(4,2,2,2,2,2,2,2,2,2,2,2,2,2,2,2,2,2,2,2,2,2,2,2,2,2,2,2,2,2,2,
2,2,2,2,2,2,2,2,2,2,2,2,2,2,2,2,2,2,2,2,2,2,2,2,2,2,2,2,2,2,2,2,2,2,2,2,
2,2,2,2,2,2,2,2,2,2,2,2,2,2,2,2,2,2,2,2,2,2,2,2,2,2,2,2,2,2,2,2,4),(1.38838504316647,
1.38850331657018,1.41256316811428,1.44667306241606,1.44811102723475,1.46649225057238,
1.47078026121916,1.47322547472784,1.47540162643616,1.4783881126609,1.48550725028072,
1.49592014500493,1.53121036702826,1.57078963891295,1.57821322467278,1.58258414872904,
1.58637316595498,1.59112839135375,1.60063468496618,1.61307917518895,1.64597237337316,
1.68389210018361,1.69005705102998,1.69284763421741,1.69500521915381,1.69753462282851,
1.70222009150174,1.70821798458257,1.75324208371746,1.79131622025913,1.79870369069099,
1.80306600069939,1.80685518199548,1.8116205870635,1.82118240752868,1.83372301547411,
1.86708290252621,1.90429856815899,1.91048908900112,1.91328403539824,1.9154419261792,
1.91796812267015,1.92263817328133,1.95937186695389,2.00891986627212,2.0171489199126,
2.02208526843446,2.02593676625895,2.03016270781747,2.03710709121351,2.06580112389977,
2.10529365796466,2.11401940909033,2.12837645384582,2.13235851468054,2.13473615847624,
2.13693609000036,2.14007345763307,2.14815486371714,2.16055820080493,2.2141235386633,
2.23416610497521,2.24061215811045,2.24473120291012,2.2486205794772,2.25389698809855,
2.26634447371481,2.28422675209128,2.31266795024048,2.32187714503914,2.34769990694516,
2.35222491717066,2.35474724607128,2.35688492438732,2.3597205397784,2.36597037686206,
2.39437673715468,2.44646960400029,2.45758228102903,2.46265717510102,2.46652855117249,
2.47068950817631,2.47733309926365,2.5016848784883,2.56327049652331,2.57095989607791,
2.57412270183141,2.57630528481707,2.57866621813506,2.58257291008395,2.59766209358923,
2.6311708372892,2.66962264116428,2.67899573405107,2.68378599503464,2.68761203478231,
2.6919694937766,2.69952942370826,2.74493413473101,2.77590460384327),
 .UNSPECIFIED.);
#1452=B_SPLINE_CURVE_WITH_KNOTS('',3,(#16804,#16805,#16806,#16807,#16808,
#16809,#16810,#16811,#16812,#16813,#16814,#16815,#16816,#16817,#16818,#16819,
#16820,#16821,#16822,#16823,#16824,#16825,#16826,#16827,#16828,#16829,#16830,
#16831,#16832,#16833,#16834,#16835,#16836,#16837,#16838,#16839,#16840,#16841,
#16842,#16843,#16844,#16845,#16846,#16847,#16848,#16849,#16850,#16851,#16852,
#16853,#16854,#16855,#16856,#16857,#16858,#16859,#16860,#16861,#16862,#16863,
#16864,#16865,#16866,#16867,#16868,#16869,#16870,#16871,#16872,#16873,#16874,
#16875,#16876,#16877,#16878,#16879,#16880,#16881,#16882,#16883,#16884,#16885,
#16886,#16887,#16888,#16889,#16890,#16891,#16892,#16893,#16894,#16895,#16896,
#16897,#16898,#16899,#16900,#16901,#16902,#16903,#16904,#16905,#16906,#16907,
#16908,#16909,#16910,#16911,#16912,#16913,#16914,#16915,#16916,#16917,#16918,
#16919,#16920,#16921,#16922,#16923,#16924,#16925,#16926,#16927,#16928,#16929,
#16930,#16931,#16932,#16933,#16934,#16935,#16936,#16937,#16938,#16939,#16940,
#16941,#16942,#16943,#16944,#16945,#16946,#16947,#16948,#16949,#16950,#16951,
#16952,#16953,#16954,#16955,#16956,#16957,#16958,#16959,#16960,#16961,#16962,
#16963,#16964,#16965,#16966,#16967,#16968,#16969,#16970,#16971,#16972,#16973,
#16974,#16975,#16976,#16977,#16978,#16979,#16980,#16981,#16982,#16983,#16984,
#16985,#16986,#16987,#16988,#16989,#16990,#16991,#16992,#16993,#16994,#16995,
#16996,#16997,#16998,#16999,#17000,#17001,#17002,#17003,#17004,#17005,#17006,
#17007,#17008,#17009,#17010,#17011,#17012,#17013),.UNSPECIFIED.,.F.,.F.,
(4,2,2,2,2,2,2,2,2,2,2,2,2,2,2,2,2,2,2,2,2,2,2,2,2,2,2,2,2,2,2,2,2,2,2,
2,2,2,2,2,2,2,2,2,2,2,2,2,2,2,2,2,2,2,2,2,2,2,2,2,2,2,2,2,2,2,2,2,2,2,2,
2,2,2,2,2,2,2,2,2,2,2,2,2,2,2,2,2,2,2,2,2,2,2,2,2,2,2,2,2,2,2,2,2,4),(1.38779141840252,
1.38798343212597,1.4200941295574,1.42466448576076,1.42718230209203,1.42931603129355,
1.43210214524226,1.43816902372091,1.46500213398631,1.51236265784808,1.52815980873776,
1.53406817122051,1.53765005781987,1.5415046631132,1.54675077690377,1.5592001045892,
1.57712914177577,1.60555853268652,1.61499139357061,1.64064669411246,1.64513951963695,
1.64764000456184,1.64975559015009,1.65255458380868,1.65869248426688,1.68622096081466,
1.73559073884686,1.74929574692861,1.75488677376961,1.75876424492972,1.76272908870636,
1.76856564521242,1.78519015610595,1.81261995164556,1.85542285589028,1.86363411170759,
1.86686333515655,1.86904240979612,1.87134558153992,1.87505658828857,1.88815045431959,
1.91410459456548,1.96304628452908,1.97129215603698,1.9762079341366,1.98002469242059,
1.98419282788319,1.99099467819026,2.01810242544466,2.04625021389738,2.05453441032295,
2.08143703927933,2.08595981212383,2.08846682702327,2.09060158029649,2.09340231752925,
2.09955071511475,2.12718617020335,2.17687348148206,2.19026267631174,2.19579648531033,
2.19966298905697,2.20364062338925,2.20954167656866,2.22669765154792,2.25554508800187,
2.29997330757964,2.30571580027897,2.30844114838567,2.31057019135909,2.31313303396502,
2.31805329943977,2.35104625300089,2.40466448394902,2.41247912984335,2.41732338293813,
2.42112060459359,2.42536903005419,2.4325461822975,2.46680266583386,2.49190339785816,
2.52223747407632,2.526779556272,2.52929069691744,2.53142462113234,2.53421861453376,
2.54033101365449,2.56761568812904,2.61628134863707,2.63068602467803,2.63638986867485,
2.63993416031327,2.6438163270291,2.6492257648443,2.66273138047077,2.68283935717001,
2.71721413585072,2.73655448432416,2.74511875093851,2.74840297010072,2.75039495632641,
2.7523847624689,2.75460988807712,2.75772530041555,2.77503528434477),
 .UNSPECIFIED.);
#1453=B_SPLINE_CURVE_WITH_KNOTS('',3,(#17014,#17015,#17016,#17017),
 .UNSPECIFIED.,.F.,.F.,(4,4),(0.000163392739190231,0.00029246168118835),
 .UNSPECIFIED.);
#1454=B_SPLINE_CURVE_WITH_KNOTS('',3,(#17019,#17020,#17021,#17022),
 .UNSPECIFIED.,.F.,.F.,(4,4),(2.77590460384327,2.77603086588106),
 .UNSPECIFIED.);
#1455=B_SPLINE_CURVE_WITH_KNOTS('',3,(#17023,#17024,#17025,#17026,#17027,
#17028,#17029,#17030,#17031,#17032,#17033,#17034,#17035,#17036,#17037,#17038,
#17039,#17040,#17041,#17042,#17043,#17044,#17045,#17046,#17047,#17048,#17049,
#17050,#17051,#17052,#17053,#17054,#17055,#17056,#17057,#17058,#17059,#17060,
#17061,#17062,#17063,#17064,#17065,#17066,#17067,#17068,#17069,#17070,#17071,
#17072,#17073,#17074,#17075,#17076,#17077,#17078,#17079,#17080,#17081,#17082,
#17083,#17084,#17085,#17086,#17087,#17088,#17089,#17090,#17091,#17092,#17093,
#17094,#17095,#17096,#17097,#17098,#17099,#17100,#17101,#17102,#17103,#17104,
#17105,#17106,#17107,#17108,#17109,#17110,#17111,#17112,#17113,#17114,#17115,
#17116,#17117,#17118,#17119,#17120,#17121,#17122,#17123,#17124,#17125,#17126,
#17127,#17128,#17129,#17130,#17131,#17132,#17133,#17134,#17135,#17136,#17137,
#17138,#17139,#17140,#17141,#17142,#17143,#17144,#17145,#17146,#17147,#17148,
#17149,#17150,#17151,#17152,#17153,#17154,#17155,#17156,#17157,#17158,#17159,
#17160,#17161,#17162,#17163,#17164,#17165,#17166,#17167,#17168,#17169,#17170,
#17171,#17172,#17173,#17174,#17175,#17176,#17177,#17178,#17179,#17180,#17181,
#17182,#17183,#17184,#17185,#17186,#17187,#17188,#17189,#17190,#17191,#17192,
#17193,#17194,#17195,#17196,#17197,#17198,#17199,#17200,#17201,#17202,#17203,
#17204,#17205,#17206,#17207,#17208,#17209,#17210,#17211,#17212,#17213,#17214,
#17215,#17216,#17217,#17218,#17219,#17220,#17221,#17222,#17223,#17224,#17225,
#17226,#17227,#17228,#17229,#17230,#17231,#17232),.UNSPECIFIED.,.F.,.F.,
(4,2,2,2,2,2,2,2,2,2,2,2,2,2,2,2,2,2,2,2,2,2,2,2,2,2,2,2,2,2,2,2,2,2,2,
2,2,2,2,2,2,2,2,2,2,2,2,2,2,2,2,2,2,2,2,2,2,2,2,2,2,2,2,2,2,2,2,2,2,2,2,
2,2,2,2,2,2,2,2,2,2,2,2,2,2,2,2,2,2,2,2,2,2,2,2,2,2,2,2,2,2,2,2,2,4),(0.000172071519088946,
0.00936200954417677,0.0149223775669653,0.017518380188118,0.0195753565284088,
0.0217251271889363,0.0244533148062466,0.0301257522401557,0.0487031491202788,
0.087748218640803,0.108099861116081,0.117389901349606,0.124970602857942,
0.129332630613796,0.133158342387564,0.137942465676234,0.14728499204543,
0.188635720076349,0.219885270247217,0.229668850919287,0.236467946344584,
0.239400183754385,0.241568242815474,0.244039959790243,0.248339588159849,
0.267928681029711,0.308718799179166,0.338827978987326,0.34585363499404,
0.350096838926966,0.353943539351612,0.358845602562056,0.366954519589289,
0.427304038829286,0.4515911703217,0.457408038422838,0.460163814382358,0.462108952690433,
0.464609661593327,0.469037341311807,0.491042611409219,0.529382799201337,
0.55931651300674,0.566332851140435,0.570574234803393,0.574421707536867,
0.579328066736765,0.589925139912958,0.64272496269062,0.671352346670467,
0.677624571272478,0.680464485685907,0.682602896576526,0.685123046349645,
0.68963732192096,0.715028593170323,0.724605226486315,0.752313070181977,
0.780010399846461,0.786893472118669,0.791106364215926,0.794961701941705,
0.799924852932101,0.808248318412805,0.856320024947246,0.894277998141745,
0.898976172261373,0.901508370041676,0.903665666865336,0.906452631902904,
0.912597330505417,0.950939765596203,0.983575954144689,1.00207891918968,
1.00817265736936,1.01221816215179,1.01610563912662,1.02159336246354,1.03439879193411,
1.08459299089626,1.11237275414485,1.11856079446773,1.12138557945048,1.12352262189201,
1.12605322828349,1.13061388620592,1.15792169624715,1.16475417716054,1.19125155847081,
1.2108201760337,1.22409352633608,1.22950078073953,1.23341301179958,1.2374905503967,
1.24373747271586,1.26194357533374,1.30706248408529,1.33542781675256,1.33997212116376,
1.34247181728779,1.34463451315869,1.34747062849104,1.35364978204733,1.38741841882821,
1.38761224885475),.UNSPECIFIED.);
#1456=B_SPLINE_CURVE_WITH_KNOTS('',3,(#17238,#17239,#17240,#17241),
 .UNSPECIFIED.,.F.,.F.,(4,4),(2.77512483966813,2.77514188312021),
 .UNSPECIFIED.);
#1457=B_SPLINE_CURVE_WITH_KNOTS('',3,(#17242,#17243,#17244,#17245,#17246,
#17247,#17248,#17249,#17250,#17251,#17252,#17253,#17254,#17255,#17256,#17257,
#17258,#17259,#17260,#17261,#17262,#17263,#17264,#17265,#17266,#17267,#17268,
#17269,#17270,#17271,#17272,#17273,#17274,#17275,#17276,#17277,#17278,#17279,
#17280,#17281,#17282,#17283,#17284,#17285,#17286,#17287,#17288,#17289,#17290,
#17291,#17292,#17293,#17294,#17295,#17296,#17297,#17298,#17299,#17300,#17301,
#17302,#17303,#17304,#17305,#17306,#17307,#17308,#17309,#17310,#17311,#17312,
#17313,#17314,#17315,#17316,#17317,#17318,#17319,#17320,#17321,#17322,#17323,
#17324,#17325,#17326,#17327,#17328,#17329,#17330,#17331,#17332,#17333,#17334,
#17335,#17336,#17337,#17338,#17339,#17340,#17341,#17342,#17343,#17344,#17345,
#17346,#17347,#17348,#17349,#17350,#17351,#17352,#17353,#17354,#17355,#17356,
#17357,#17358,#17359,#17360,#17361,#17362,#17363,#17364,#17365,#17366,#17367,
#17368,#17369,#17370,#17371,#17372,#17373,#17374,#17375,#17376,#17377,#17378,
#17379,#17380,#17381,#17382,#17383,#17384,#17385,#17386,#17387,#17388,#17389,
#17390,#17391,#17392,#17393,#17394,#17395,#17396,#17397,#17398,#17399,#17400,
#17401,#17402,#17403,#17404,#17405,#17406,#17407,#17408,#17409,#17410,#17411,
#17412,#17413,#17414,#17415,#17416,#17417,#17418,#17419,#17420,#17421,#17422,
#17423,#17424,#17425,#17426,#17427,#17428,#17429,#17430,#17431,#17432,#17433,
#17434,#17435,#17436,#17437,#17438,#17439,#17440,#17441),.UNSPECIFIED.,
 .F.,.F.,(4,2,2,2,2,2,2,2,2,2,2,2,2,2,2,2,2,2,2,2,2,2,2,2,2,2,2,2,2,2,2,
2,2,2,2,2,2,2,2,2,2,2,2,2,2,2,2,2,2,2,2,2,2,2,2,2,2,2,2,2,2,2,2,2,2,2,2,
2,2,2,2,2,2,2,2,2,2,2,2,2,2,2,2,2,2,2,2,2,2,2,2,2,2,2,2,2,2,2,2,4),(0.000192294988332048,
0.00607774719199029,0.0159169377236619,0.07398278467463,0.0901646279759542,
0.0967572037642757,0.101789524963687,0.104375587497259,0.10650371489967,
0.109202356866135,0.114803382211837,0.16059142721058,0.196384128692415,
0.207600242466767,0.212640225162752,0.216462826940986,0.220613265208185,
0.227331659049338,0.250360447559232,0.292397197982038,0.316101434412589,
0.321829231388031,0.324552020232788,0.326477015027514,0.328953908172427,
0.33334143309214,0.355071843920419,0.395089530730404,0.414212590606075,
0.42724804380981,0.432586554350752,0.436456819337085,0.44001704407753,0.445806861315989,
0.460777886563664,0.508888319781673,0.535978950451558,0.542072291622704,
0.544863168881321,0.546997240027056,0.549511512862563,0.554066242389265,
0.583546817453881,0.587892618058118,0.614224450006721,0.634122871496563,
0.643256189518113,0.650722921113714,0.655033860901014,0.658822355223786,
0.663569000615594,0.672863167770376,0.71546994844784,0.745873505836473,
0.755495636212241,0.762198933713271,0.765097778384368,0.767243682066841,
0.769690728384777,0.773946038582735,0.793176491308406,0.833021861268238,
0.864454730694058,0.871506455998565,0.875728489632487,0.879531940886113,
0.884425708407359,0.892408932896183,0.94443693775125,0.979190556805713,
0.983813268960183,0.986314367903372,0.988450298902266,0.991213530673869,
0.997317477465039,1.03601623075896,1.06850824923919,1.08084337654213,1.09026779983028,
1.09497866262644,1.09872966362081,1.10305293478694,1.11038375425721,1.14919005723998,
1.1774142228651,1.19277177394523,1.20214101896883,1.20543966566109,1.20765446748141,
1.20994392277896,1.21359190852609,1.224891134927,1.2651457388595,1.30479198503359,
1.31214463190117,1.31643114138381,1.32022284661305,1.32500655037598,1.33261294246727,
1.38779141840252),.UNSPECIFIED.);
#1458=B_SPLINE_CURVE_WITH_KNOTS('',3,(#17443,#17444,#17445,#17446,#17447,
#17448,#17449,#17450,#17451,#17452,#17453,#17454,#17455,#17456,#17457,#17458,
#17459,#17460,#17461,#17462,#17463,#17464,#17465,#17466,#17467,#17468,#17469,
#17470,#17471,#17472,#17473,#17474,#17475,#17476,#17477,#17478,#17479,#17480,
#17481,#17482,#17483,#17484,#17485,#17486,#17487,#17488,#17489,#17490,#17491,
#17492,#17493,#17494,#17495,#17496,#17497,#17498,#17499,#17500,#17501,#17502,
#17503,#17504,#17505,#17506,#17507,#17508,#17509,#17510,#17511,#17512,#17513,
#17514,#17515,#17516,#17517,#17518,#17519,#17520,#17521,#17522,#17523,#17524,
#17525,#17526,#17527,#17528,#17529,#17530,#17531,#17532,#17533,#17534,#17535,
#17536,#17537,#17538,#17539,#17540,#17541,#17542,#17543,#17544,#17545,#17546,
#17547,#17548,#17549,#17550,#17551,#17552,#17553,#17554,#17555,#17556,#17557,
#17558,#17559,#17560,#17561,#17562,#17563,#17564,#17565,#17566,#17567,#17568,
#17569,#17570,#17571,#17572,#17573,#17574,#17575,#17576,#17577,#17578,#17579,
#17580,#17581,#17582,#17583,#17584,#17585,#17586,#17587,#17588,#17589,#17590,
#17591,#17592,#17593,#17594,#17595,#17596,#17597,#17598,#17599,#17600,#17601,
#17602,#17603,#17604,#17605,#17606,#17607,#17608,#17609,#17610,#17611,#17612,
#17613,#17614,#17615,#17616,#17617,#17618,#17619,#17620,#17621,#17622,#17623,
#17624,#17625,#17626,#17627,#17628,#17629,#17630,#17631,#17632,#17633,#17634,
#17635,#17636,#17637,#17638,#17639,#17640),.UNSPECIFIED.,.F.,.F.,(4,2,2,
2,2,2,2,2,2,2,2,2,2,2,2,2,2,2,2,2,2,2,2,2,2,2,2,2,2,2,2,2,2,2,2,2,2,2,2,
2,2,2,2,2,2,2,2,2,2,2,2,2,2,2,2,2,2,2,2,2,2,2,2,2,2,2,2,2,2,2,2,2,2,2,2,
2,2,2,2,2,2,2,2,2,2,2,2,2,2,2,2,2,2,2,2,2,2,2,4),(1.38761224885475,1.4375036834497,
1.44569227850445,1.45061742311542,1.45446772566586,1.45870005310481,1.46567288350149,
1.49483724008579,1.53528308292903,1.55609614703464,1.56047418521489,1.56296387561242,
1.56491109692638,1.56768378278985,1.57358957035062,1.59867955919373,1.64123407087175,
1.66244243379664,1.66901419641069,1.67316053539395,1.67703909251926,1.68224443940608,
1.69425472675965,1.7413424817255,1.75085880380665,1.77630312287379,1.78081890893236,
1.78333954448885,1.78547810079993,1.7883179040798,1.79458860908678,1.82319783612459,
1.87591877396272,1.88555676656238,1.89040085508792,1.89398340270088,1.89790512472803,
1.90336650767092,1.91699752311241,1.93731941143245,1.98024552865551,1.99740812312745,
2.00161523245294,2.00404217779395,2.00622305592542,2.00924428024446,2.01657765486436,
2.02742099020821,2.06581876662872,2.10174465708663,2.10915591987101,2.11348218716905,
2.11693013752729,2.12158335290285,2.13057192847698,2.16304397066469,2.21490148709462,
2.22092467880892,2.22368963628375,2.22584498402527,2.22839318537159,2.23316739266884,
2.27080250147295,2.31913182360865,2.32744321612165,2.33240298851514,2.33625790394365,
2.34047255901488,2.34736365037911,2.37518965446231,2.40276282874832,2.41235029489264,
2.43768200497963,2.44219440404535,2.44471415568999,2.44685263659423,2.44969322094216,
2.45596905321813,2.48463334787844,2.53752115695101,2.54805836137235,2.55300695126462,
2.55684944912774,2.56111202791627,2.56822714023535,2.60006810498364,2.63864476614718,
2.65848492538306,2.6627967589665,2.66527131939438,2.66743883486286,2.67036632329412,
2.67713710462138,2.68686653808941,2.71778445042413,2.76083141921413,2.76892977369379,
2.77242616593864,2.7752680731555),.UNSPECIFIED.);
#1459=B_SPLINE_CURVE_WITH_KNOTS('',3,(#17641,#17642,#17643,#17644),
 .UNSPECIFIED.,.F.,.F.,(4,4),(0.000193089214357908,0.000209030494615362),
 .UNSPECIFIED.);
#1460=B_SPLINE_CURVE_WITH_KNOTS('',3,(#17649,#17650,#17651,#17652,#17653,
#17654,#17655,#17656,#17657,#17658,#17659,#17660,#17661,#17662,#17663,#17664,
#17665,#17666,#17667,#17668,#17669,#17670,#17671,#17672,#17673,#17674,#17675,
#17676,#17677,#17678,#17679,#17680,#17681,#17682,#17683,#17684,#17685,#17686,
#17687,#17688,#17689,#17690,#17691,#17692,#17693,#17694,#17695,#17696,#17697,
#17698,#17699,#17700,#17701,#17702,#17703,#17704,#17705,#17706,#17707,#17708,
#17709,#17710,#17711,#17712,#17713,#17714,#17715,#17716,#17717,#17718,#17719,
#17720,#17721,#17722,#17723,#17724,#17725,#17726,#17727,#17728,#17729,#17730,
#17731,#17732,#17733,#17734,#17735,#17736,#17737,#17738,#17739,#17740,#17741,
#17742,#17743,#17744,#17745,#17746,#17747,#17748,#17749,#17750,#17751,#17752,
#17753,#17754,#17755,#17756,#17757,#17758,#17759,#17760,#17761,#17762,#17763,
#17764,#17765,#17766,#17767,#17768,#17769,#17770,#17771,#17772,#17773,#17774,
#17775,#17776,#17777,#17778,#17779,#17780,#17781,#17782,#17783,#17784,#17785,
#17786,#17787,#17788,#17789,#17790,#17791,#17792,#17793,#17794,#17795,#17796,
#17797,#17798,#17799,#17800,#17801,#17802,#17803,#17804,#17805,#17806,#17807,
#17808,#17809,#17810,#17811,#17812,#17813,#17814,#17815,#17816,#17817,#17818,
#17819,#17820,#17821,#17822,#17823,#17824,#17825,#17826,#17827,#17828,#17829,
#17830,#17831,#17832,#17833,#17834,#17835,#17836,#17837,#17838,#17839,#17840,
#17841,#17842,#17843,#17844,#17845,#17846,#17847,#17848,#17849,#17850),
 .UNSPECIFIED.,.F.,.F.,(4,2,2,2,2,2,2,2,2,2,2,2,2,2,2,2,2,2,2,2,2,2,2,2,
2,2,2,2,2,2,2,2,2,2,2,2,2,2,2,2,2,2,2,2,2,2,2,2,2,2,2,2,2,2,2,2,2,2,2,2,
2,2,2,2,2,2,2,2,2,2,2,2,2,2,2,2,2,2,2,2,2,2,2,2,2,2,2,2,2,2,2,2,2,2,2,2,
2,2,2,2,4),(1.38767510941596,1.43112339601124,1.44039605580476,1.44513822465615,
1.44892626641656,1.45324005326402,1.4607204652113,1.46987448009624,1.4898415576597,
1.52903693125285,1.55018848634903,1.55455167320753,1.55702308145833,1.55894891956946,
1.56167959070667,1.56744907664187,1.59152382227246,1.63398317565435,1.6562623897388,
1.66294678284684,1.667089862421,1.670914744851,1.67597115047239,1.68728264468901,
1.72447587287317,1.76838266036149,1.77360945357837,1.77626714490509,1.77843300468403,
1.78075910335023,1.78457427656286,1.79884019787084,1.82906442645773,1.8719474956498,
1.88123774140026,1.88598344359576,1.88977168520334,1.89408287462065,1.90155145899932,
1.94809725340194,1.98843599942715,1.99449305198681,1.99724772480496,1.99938273452405,
2.00188958904393,2.00653998509891,2.04160575405013,2.09322857418171,2.10125434864285,
2.1061077163419,2.10991600606091,2.11411582525755,2.12106500774562,2.15057975615587,
2.17704738011528,2.18456687635986,2.21123387371285,2.21575145986064,2.2182573269305,
2.22039224892657,2.22319470419431,2.22935251871928,2.25708114858392,2.30704362751151,
2.320151926046,2.32564359127026,2.32950235273933,2.33349037636555,2.33944222748397,
2.35702651517694,2.38705959140961,2.42953922260409,2.43542611973755,2.43817862954996,
2.44030938448975,2.44285093341491,2.44766816192961,2.48368691196931,2.53383013242079,
2.54198250244127,2.54687154157531,2.55068421411694,2.554864798135,2.56172602988879,
2.58976962046305,2.61718293651675,2.62711231982529,2.65212325591286,2.65659795418927,
2.65909406831023,2.66120976551139,2.66401387584751,2.67018195298076,2.69801670035432,
2.72985904665648,2.74368990936215,2.75988741174204,2.76571496966692,2.76972187890552,
2.77245863450725,2.77512483966813),.UNSPECIFIED.);
#1461=B_SPLINE_CURVE_WITH_KNOTS('',3,(#17851,#17852,#17853,#17854,#17855,
#17856,#17857,#17858,#17859,#17860,#17861,#17862,#17863,#17864,#17865,#17866,
#17867,#17868,#17869,#17870,#17871,#17872,#17873,#17874,#17875,#17876,#17877,
#17878,#17879,#17880,#17881,#17882,#17883,#17884,#17885,#17886,#17887,#17888,
#17889,#17890,#17891,#17892,#17893,#17894,#17895,#17896,#17897,#17898,#17899,
#17900,#17901,#17902,#17903,#17904,#17905,#17906,#17907,#17908,#17909,#17910,
#17911,#17912,#17913,#17914,#17915,#17916,#17917,#17918,#17919,#17920,#17921,
#17922,#17923,#17924,#17925,#17926,#17927,#17928,#17929,#17930,#17931,#17932,
#17933,#17934,#17935,#17936,#17937,#17938,#17939,#17940,#17941,#17942,#17943,
#17944,#17945,#17946,#17947,#17948,#17949,#17950,#17951,#17952,#17953,#17954,
#17955,#17956,#17957,#17958,#17959,#17960,#17961,#17962,#17963,#17964,#17965,
#17966,#17967,#17968,#17969,#17970,#17971,#17972,#17973,#17974,#17975,#17976,
#17977,#17978,#17979,#17980,#17981,#17982,#17983,#17984,#17985,#17986,#17987,
#17988,#17989,#17990,#17991,#17992,#17993,#17994,#17995,#17996,#17997,#17998,
#17999,#18000,#18001,#18002,#18003,#18004,#18005,#18006,#18007,#18008,#18009,
#18010,#18011,#18012,#18013,#18014,#18015,#18016,#18017,#18018,#18019,#18020,
#18021,#18022,#18023,#18024,#18025,#18026,#18027,#18028,#18029,#18030,#18031,
#18032,#18033,#18034,#18035,#18036,#18037,#18038,#18039,#18040,#18041,#18042,
#18043,#18044,#18045,#18046,#18047,#18048),.UNSPECIFIED.,.F.,.F.,(4,2,2,
2,2,2,2,2,2,2,2,2,2,2,2,2,2,2,2,2,2,2,2,2,2,2,2,2,2,2,2,2,2,2,2,2,2,2,2,
2,2,2,2,2,2,2,2,2,2,2,2,2,2,2,2,2,2,2,2,2,2,2,2,2,2,2,2,2,2,2,2,2,2,2,2,
2,2,2,2,2,2,2,2,2,2,2,2,2,2,2,2,2,2,2,2,2,2,2,4),(0.000209030494615362,
0.00359170171313374,0.00801319147981052,0.0168020728302088,0.0773841769243228,
0.0952639350494035,0.105662925707357,0.109110945700868,0.111372170731263,
0.113384935493905,0.116163707070484,0.121830924692454,0.154946762097185,
0.185063790401504,0.209892269349023,0.216574301011722,0.220744210447303,
0.224613714204544,0.229671442592147,0.24113488885533,0.29299636669776,0.321327317194173,
0.32757058501874,0.330405434572305,0.332562866576736,0.335095005299073,
0.339662368457123,0.367341553470571,0.373741392744492,0.400169432933991,
0.429737036675418,0.436733589690745,0.440971115406994,0.444820258480975,
0.449735833184954,0.460382030936677,0.513136618016726,0.541751483294464,
0.54802297013801,0.550862995213566,0.553001681614494,0.555522386873839,
0.56003817770707,0.585465026779176,0.594666611669455,0.622067891505925,
0.650352030154785,0.657272765501373,0.661494139070315,0.66534780527941,
0.670295699394434,0.67856378793407,0.727558021069206,0.76440175930056,0.769282192585346,
0.771852685231552,0.774005962863598,0.776788042303393,0.78274306530777,
0.824305005342297,0.869604671686738,0.877203700112034,0.88157022621598,
0.885396356731324,0.890176359323216,0.899495816355134,0.942479013417658,
0.972514384964752,0.982094422924452,0.988788646646961,0.991703277619357,
0.993869516415409,0.996352090173414,1.00069820616056,1.02123427420754,1.06109214394567,
1.09113136745582,1.09815440120173,1.10239766390826,1.10624546199257,1.11115035099432,
1.1217365090302,1.17455898542707,1.20319545612348,1.20946913297048,1.21230958461967,
1.21444834878919,1.2169688539126,1.22148362417786,1.24687030071953,1.25645414820602,
1.28415538801843,1.31187016647005,1.31875518533815,1.32296893908029,1.32682485082551,
1.3317884416477,1.34011196177077,1.38801450560634),.UNSPECIFIED.);
#1462=B_SPLINE_CURVE_WITH_KNOTS('',3,(#18054,#18055,#18056,#18057),
 .UNSPECIFIED.,.F.,.F.,(4,4),(2.7753563039814,2.77545271603152),
 .UNSPECIFIED.);
#1463=B_SPLINE_CURVE_WITH_KNOTS('',3,(#18058,#18059,#18060,#18061,#18062,
#18063,#18064,#18065,#18066,#18067,#18068,#18069,#18070,#18071,#18072,#18073,
#18074,#18075,#18076,#18077,#18078,#18079,#18080,#18081,#18082,#18083,#18084,
#18085,#18086,#18087,#18088,#18089,#18090,#18091,#18092,#18093,#18094,#18095,
#18096,#18097,#18098,#18099,#18100,#18101,#18102,#18103,#18104,#18105,#18106,
#18107,#18108,#18109,#18110,#18111,#18112,#18113,#18114,#18115,#18116,#18117,
#18118,#18119,#18120,#18121,#18122,#18123,#18124,#18125,#18126,#18127,#18128,
#18129,#18130,#18131,#18132,#18133,#18134,#18135,#18136,#18137,#18138,#18139,
#18140,#18141,#18142,#18143,#18144,#18145,#18146,#18147,#18148,#18149,#18150,
#18151,#18152,#18153,#18154,#18155,#18156,#18157,#18158,#18159,#18160,#18161,
#18162,#18163,#18164,#18165,#18166,#18167,#18168,#18169,#18170,#18171,#18172,
#18173,#18174,#18175,#18176,#18177,#18178,#18179,#18180,#18181,#18182,#18183,
#18184,#18185,#18186,#18187,#18188,#18189,#18190,#18191,#18192,#18193,#18194,
#18195,#18196,#18197,#18198,#18199,#18200,#18201,#18202,#18203,#18204,#18205,
#18206,#18207,#18208,#18209,#18210,#18211,#18212,#18213,#18214,#18215,#18216,
#18217,#18218,#18219,#18220,#18221,#18222,#18223,#18224,#18225,#18226,#18227,
#18228,#18229,#18230,#18231,#18232,#18233,#18234,#18235,#18236,#18237,#18238,
#18239,#18240,#18241,#18242,#18243,#18244,#18245,#18246,#18247,#18248,#18249,
#18250,#18251,#18252,#18253,#18254,#18255,#18256,#18257),.UNSPECIFIED.,
 .F.,.F.,(4,2,2,2,2,2,2,2,2,2,2,2,2,2,2,2,2,2,2,2,2,2,2,2,2,2,2,2,2,2,2,
2,2,2,2,2,2,2,2,2,2,2,2,2,2,2,2,2,2,2,2,2,2,2,2,2,2,2,2,2,2,2,2,2,2,2,2,
2,2,2,2,2,2,2,2,2,2,2,2,2,2,2,2,2,2,2,2,2,2,2,2,2,2,2,2,2,2,2,2,4),(0.000182437931283686,
0.00653692196294665,0.0108609769573606,0.0130104903736253,0.0150542688106974,
0.0174265179469178,0.0214524366139877,0.0365305767037021,0.0787787328981987,
0.112285268459346,0.119432154772533,0.123674304161217,0.127473076906101,
0.132329194520251,0.140183791302266,0.193418740748948,0.227209744564475,
0.231821371483504,0.234319960305755,0.236455980335452,0.239222140074427,
0.245343379061742,0.283777908787235,0.316431851796508,0.328800611429692,
0.338244415141556,0.342958716191094,0.346709629394816,0.351029672091661,
0.358347407511598,0.399293664646039,0.432218473687358,0.443319513919408,
0.450765804092565,0.453786996395798,0.455950525789809,0.458336648643501,
0.462425926225514,0.478257660101814,0.51518183976668,0.552858135690341,
0.560156493659421,0.564431148432792,0.568224274037932,0.573025854561165,
0.580693819723936,0.63554907648934,0.66809932039209,0.672694513102882,0.675189667523938,
0.677326268798803,0.680097618843394,0.686023781836444,0.726898002540094,
0.772857763492995,0.780420281881811,0.7847513199462,0.788537009749807,0.793253270518437,
0.802401512598282,0.849485432533971,0.888475380488218,0.893122875235794,
0.895629066872899,0.897764063953238,0.90051945331205,0.90658077126419,0.946906838339564,
0.978290226453303,0.99634421909439,1.00235065791773,1.0063501174987,1.01020134143816,
1.01565028997868,1.0284328994166,1.07868462375402,1.10650661952783,1.11267410875596,
1.11547842035182,1.11759449172151,1.12009127611521,1.12456776472346,1.14960733215508,
1.15925455897892,1.18662796642128,1.21498656698914,1.22186840447295,1.2260539053021,
1.22986613635138,1.23474780735677,1.24287251263121,1.29338128185761,1.32937531542901,
1.33400890093295,1.33651227482695,1.33864784944877,1.3414077292625,1.34749320595248,
1.38747360616315,1.38767510941596),.UNSPECIFIED.);
#1464=B_SPLINE_CURVE_WITH_KNOTS('',3,(#18259,#18260,#18261,#18262,#18263,
#18264,#18265,#18266,#18267,#18268,#18269,#18270,#18271,#18272,#18273,#18274,
#18275,#18276,#18277,#18278,#18279,#18280,#18281,#18282,#18283,#18284,#18285,
#18286,#18287,#18288,#18289,#18290,#18291,#18292,#18293,#18294,#18295,#18296,
#18297,#18298,#18299,#18300,#18301,#18302,#18303,#18304,#18305,#18306,#18307,
#18308,#18309,#18310,#18311,#18312,#18313,#18314,#18315,#18316,#18317,#18318,
#18319,#18320,#18321,#18322,#18323,#18324,#18325,#18326,#18327,#18328,#18329,
#18330,#18331,#18332,#18333,#18334,#18335,#18336,#18337,#18338,#18339,#18340,
#18341,#18342,#18343,#18344,#18345,#18346,#18347,#18348,#18349,#18350,#18351,
#18352,#18353,#18354,#18355,#18356,#18357,#18358,#18359,#18360,#18361,#18362,
#18363,#18364,#18365,#18366,#18367,#18368,#18369,#18370,#18371,#18372,#18373,
#18374,#18375,#18376,#18377,#18378,#18379,#18380,#18381,#18382,#18383,#18384,
#18385,#18386,#18387,#18388,#18389,#18390,#18391,#18392,#18393,#18394,#18395,
#18396,#18397,#18398,#18399,#18400,#18401,#18402,#18403,#18404,#18405,#18406,
#18407,#18408,#18409,#18410,#18411,#18412,#18413,#18414,#18415,#18416,#18417,
#18418,#18419,#18420,#18421,#18422,#18423,#18424,#18425,#18426,#18427,#18428,
#18429,#18430,#18431,#18432,#18433,#18434,#18435,#18436,#18437,#18438,#18439,
#18440,#18441,#18442,#18443,#18444,#18445,#18446,#18447,#18448,#18449,#18450,
#18451,#18452,#18453,#18454,#18455,#18456,#18457,#18458,#18459,#18460,#18461,
#18462),.UNSPECIFIED.,.F.,.F.,(4,2,2,2,2,2,2,2,2,2,2,2,2,2,2,2,2,2,2,2,
2,2,2,2,2,2,2,2,2,2,2,2,2,2,2,2,2,2,2,2,2,2,2,2,2,2,2,2,2,2,2,2,2,2,2,2,
2,2,2,2,2,2,2,2,2,2,2,2,2,2,2,2,2,2,2,2,2,2,2,2,2,2,2,2,2,2,2,2,2,2,2,2,
2,2,2,2,2,2,2,2,2,4),(1.38801450560634,1.38821456747388,1.42369817782745,
1.42987238324046,1.43270770026876,1.4348704745835,1.43737103384921,1.44191880317453,
1.47039613150064,1.51578708719391,1.53371666506104,1.53993350385607,1.54400493083112,
1.54792120899495,1.55335026593637,1.56676498054793,1.58662744885994,1.6245372297973,
1.64695043283158,1.65139870467833,1.65390430628611,1.65584906348525,1.65859891302686,
1.6643829672707,1.68837409257627,1.74936329691702,1.7573420296936,1.76225984412887,
1.7660990874891,1.77037923682112,1.77757505223168,1.81117244864818,1.83932650150939,
1.86722547611572,1.87179560628477,1.87432829162228,1.87648550929775,1.87931922885402,
1.88555670049086,1.91383161529013,1.96551092154086,1.9770161386787,1.98170015466075,
1.98559929567117,1.98962758954039,1.99563829100745,2.01341542365613,2.04391184079909,
2.08555536014992,2.09150136733144,2.0942814291946,2.09643418581836,2.09900527847287,
2.10389012439133,2.14162809669519,2.18962680149004,2.19795596139163,2.20292051357819,
2.20677582364425,2.21098756183324,2.21786618783751,2.24550421666454,2.27323503645635,
2.28273971127688,2.30819372340121,2.31270911565288,2.31522940366754,2.31736757956771,
2.32020676598859,2.32647567800876,2.35507271951081,2.40776159121395,2.41847558330981,
2.42340255888651,2.42725248056222,2.43148253927356,2.43844730970399,2.46749164939931,
2.50853866858637,2.52893119103873,2.5332724157782,2.53575350135751,2.53791934118645,
2.54083469188214,2.54753569624607,2.55713056954624,2.58725526451146,2.63013596140322,
2.63945693115457,2.64423649514728,2.64806167924772,2.65242647931279,2.66002084554227,
2.70519835219979,2.73064921276551,2.74894487887096,2.75350970097938,2.75604098286511,
2.75817777618934,2.76029487092824,2.76308355449852,2.77549281338982),
 .UNSPECIFIED.);
#1465=B_SPLINE_CURVE_WITH_KNOTS('',3,(#18463,#18464,#18465,#18466),
 .UNSPECIFIED.,.F.,.F.,(4,4),(0.000175379134418719,0.000274764919486373),
 .UNSPECIFIED.);
#1466=B_SPLINE_CURVE_WITH_KNOTS('',3,(#18471,#18472,#18473,#18474,#18475,
#18476,#18477,#18478,#18479,#18480,#18481,#18482,#18483,#18484,#18485,#18486,
#18487,#18488,#18489,#18490,#18491,#18492,#18493,#18494,#18495,#18496,#18497,
#18498,#18499,#18500,#18501,#18502,#18503,#18504,#18505,#18506,#18507,#18508,
#18509,#18510,#18511,#18512,#18513,#18514,#18515,#18516,#18517,#18518,#18519,
#18520,#18521,#18522,#18523,#18524,#18525,#18526,#18527,#18528,#18529,#18530,
#18531,#18532,#18533,#18534,#18535,#18536,#18537,#18538,#18539,#18540,#18541,
#18542,#18543,#18544,#18545,#18546,#18547,#18548,#18549,#18550,#18551,#18552,
#18553,#18554,#18555,#18556,#18557,#18558,#18559,#18560,#18561,#18562,#18563,
#18564,#18565,#18566,#18567,#18568,#18569,#18570,#18571,#18572,#18573,#18574,
#18575,#18576,#18577,#18578,#18579,#18580,#18581,#18582,#18583,#18584,#18585,
#18586,#18587,#18588,#18589,#18590,#18591,#18592,#18593,#18594,#18595,#18596,
#18597,#18598,#18599,#18600,#18601,#18602,#18603,#18604,#18605,#18606,#18607,
#18608,#18609,#18610,#18611,#18612,#18613,#18614,#18615,#18616,#18617,#18618,
#18619,#18620,#18621,#18622,#18623,#18624,#18625,#18626,#18627,#18628,#18629,
#18630,#18631,#18632,#18633,#18634,#18635,#18636,#18637,#18638,#18639,#18640,
#18641,#18642,#18643,#18644,#18645,#18646,#18647,#18648,#18649,#18650,#18651,
#18652,#18653,#18654,#18655,#18656,#18657,#18658,#18659,#18660,#18661,#18662,
#18663,#18664,#18665,#18666,#18667,#18668,#18669,#18670),.UNSPECIFIED.,
 .F.,.F.,(4,2,2,2,2,2,2,2,2,2,2,2,2,2,2,2,2,2,2,2,2,2,2,2,2,2,2,2,2,2,2,
2,2,2,2,2,2,2,2,2,2,2,2,2,2,2,2,2,2,2,2,2,2,2,2,2,2,2,2,2,2,2,2,2,2,2,2,
2,2,2,2,2,2,2,2,2,2,2,2,2,2,2,2,2,2,2,2,2,2,2,2,2,2,2,2,2,2,2,2,4),(1.38783032955465,
1.38797382247406,1.42164717525487,1.45687548489826,1.46249483302315,1.46524838667397,
1.46724168212058,1.46947786297659,1.47287966671787,1.48306736885704,1.50045347420167,
1.54234804406643,1.56573909297665,1.57247812833265,1.57663306124756,1.58045434953077,
1.5854845802705,1.5966444173606,1.63111992479794,1.67316555063445,1.68224445455045,
1.68560198432229,1.6876079490253,1.68982914228136,1.69315900789914,1.7027688470521,
1.71870904191044,1.76597962238645,1.78669875942825,1.79317890893748,1.79727833693069,
1.80111968176933,1.8062841723444,1.81823369476285,1.8649872473264,1.87017244894104,
1.90031845774389,1.90487452889868,1.9073891600646,1.90952326180928,1.91231385939691,
1.91840532083447,1.94547724524786,1.99352125702125,2.00859085316158,2.01439529014585,
2.01795822203195,2.02182651726854,2.02715332607901,2.04011314850359,2.05907796824362,
2.08624978775251,2.09576383231955,2.12087042173293,2.12534848166642,2.12784564971207,
2.1299616925156,2.13276554675666,2.13893033033105,2.16672552088088,2.21688296002443,
2.22979164382826,2.23525711926235,2.23911134411923,2.24310649636951,2.24909197912153,
2.26696342902514,2.29781391881057,2.33900777215224,2.34497063530561,2.34770808693128,
2.34984141131703,2.35236043309928,2.35706911434152,2.3631197473591,2.37731632436639,
2.4063006888814,2.44622670283569,2.45353628082957,2.45785452368577,2.46160569764634,
2.46632271232396,2.4757804549929,2.48817189177434,2.52093544841506,2.55917949482486,
2.56529664159717,2.56806204196975,2.57019797929527,2.57269703828066,2.5773109881588,
2.61125912562925,2.66433002274866,2.67220591481856,2.67706814950483,2.68086752354038,
2.68510602794984,2.69223625731738,2.72537166303582,2.7753563039814),
 .UNSPECIFIED.);
#1467=B_SPLINE_CURVE_WITH_KNOTS('',3,(#18671,#18672,#18673,#18674,#18675,
#18676,#18677,#18678,#18679,#18680,#18681,#18682,#18683,#18684,#18685,#18686,
#18687,#18688,#18689,#18690,#18691,#18692,#18693,#18694,#18695,#18696,#18697,
#18698,#18699,#18700,#18701,#18702,#18703,#18704,#18705,#18706,#18707,#18708,
#18709,#18710,#18711,#18712,#18713,#18714,#18715,#18716,#18717,#18718,#18719,
#18720,#18721,#18722,#18723,#18724,#18725,#18726,#18727,#18728,#18729,#18730,
#18731,#18732,#18733,#18734,#18735,#18736,#18737,#18738,#18739,#18740,#18741,
#18742,#18743,#18744,#18745,#18746,#18747,#18748,#18749,#18750,#18751,#18752,
#18753,#18754,#18755,#18756,#18757,#18758,#18759,#18760,#18761,#18762,#18763,
#18764,#18765,#18766,#18767,#18768,#18769,#18770,#18771,#18772,#18773,#18774,
#18775,#18776,#18777,#18778,#18779,#18780,#18781,#18782,#18783,#18784,#18785,
#18786,#18787,#18788,#18789,#18790,#18791,#18792,#18793,#18794,#18795,#18796,
#18797,#18798,#18799,#18800,#18801,#18802,#18803,#18804,#18805,#18806,#18807,
#18808,#18809,#18810,#18811,#18812,#18813,#18814,#18815,#18816,#18817,#18818,
#18819,#18820,#18821,#18822,#18823,#18824,#18825,#18826,#18827,#18828,#18829,
#18830,#18831,#18832,#18833,#18834,#18835,#18836,#18837,#18838,#18839,#18840,
#18841,#18842,#18843,#18844,#18845,#18846,#18847,#18848,#18849,#18850,#18851,
#18852,#18853,#18854,#18855,#18856,#18857,#18858,#18859,#18860,#18861,#18862,
#18863,#18864,#18865,#18866,#18867,#18868),.UNSPECIFIED.,.F.,.F.,(4,2,2,
2,2,2,2,2,2,2,2,2,2,2,2,2,2,2,2,2,2,2,2,2,2,2,2,2,2,2,2,2,2,2,2,2,2,2,2,
2,2,2,2,2,2,2,2,2,2,2,2,2,2,2,2,2,2,2,2,2,2,2,2,2,2,2,2,2,2,2,2,2,2,2,2,
2,2,2,2,2,2,2,2,2,2,2,2,2,2,2,2,2,2,2,2,2,2,2,4),(0.000274764919486373,
0.062895630461027,0.0813501395675178,0.0874374187852338,0.0914808653973023,
0.0953680021534591,0.100858040901126,0.113687483403507,0.163842339124501,
0.193602521989007,0.198516403059142,0.201093239299371,0.2032450839026,0.206016656515119,
0.211918773340013,0.254215798711661,0.267386429908165,0.288843042588712,
0.302995696994059,0.308533403799369,0.312468373296255,0.316035183053858,
0.320816070505866,0.332701264299013,0.383864897410737,0.411964006093194,
0.418183334875138,0.421013422479729,0.42315056372249,0.425676584954236,
0.430218191572825,0.456688328809736,0.464516978629412,0.465739291622078,
0.495293695956529,0.520819755702825,0.527553043852622,0.531733369714844,
0.535598121938227,0.540629010791724,0.551938814644686,0.603952953025513,
0.632329023987934,0.638576056771627,0.641411234767869,0.643568306936236,
0.646099303556593,0.650662943396744,0.678173056626024,0.684761543505955,
0.710982094544844,0.74070615673981,0.747710453462217,0.751949078120344,
0.755796928922688,0.760707714572317,0.768847256701182,0.819450935999529,
0.855260572573492,0.859923279949871,0.862447841705736,0.864605972203848,
0.867403266015435,0.873606362357614,0.910529596186081,0.944109446073919,
0.956695639037509,0.9662832342947,0.971053702999564,0.974843406677438,0.979202462142167,
0.986575095102644,1.02538752318016,1.0537871748655,1.0689472681226,1.07528063488783,
1.0801682480595,1.0827398339018,1.08489240967791,1.08767150247474,1.09361278042131,
1.13536556076732,1.18047633506502,1.18807044408786,1.19243522838387,1.19626046527789,
1.20104018437499,1.21036178088627,1.25312035944959,1.2833067121169,1.29758815417143,
1.30142838602475,1.30377475737461,1.30596503157037,1.30917005368632,1.31712542592157,
1.36014291061841,1.38762556260924,1.38776860835863),.UNSPECIFIED.);
#1468=B_SPLINE_CURVE_WITH_KNOTS('',3,(#18873,#18874,#18875,#18876,#18877,
#18878,#18879,#18880,#18881,#18882,#18883,#18884,#18885,#18886,#18887,#18888,
#18889,#18890,#18891,#18892,#18893,#18894,#18895,#18896,#18897,#18898,#18899,
#18900,#18901,#18902,#18903,#18904,#18905,#18906,#18907,#18908,#18909,#18910,
#18911,#18912,#18913,#18914,#18915,#18916,#18917,#18918,#18919,#18920,#18921,
#18922,#18923,#18924,#18925,#18926,#18927,#18928,#18929,#18930,#18931,#18932,
#18933,#18934,#18935,#18936,#18937,#18938,#18939,#18940,#18941,#18942,#18943,
#18944,#18945,#18946,#18947,#18948,#18949,#18950,#18951,#18952,#18953,#18954,
#18955,#18956,#18957,#18958,#18959,#18960,#18961,#18962,#18963,#18964,#18965,
#18966,#18967,#18968,#18969,#18970,#18971,#18972,#18973,#18974,#18975,#18976,
#18977,#18978,#18979,#18980,#18981,#18982,#18983,#18984,#18985,#18986,#18987,
#18988,#18989,#18990,#18991,#18992,#18993,#18994,#18995,#18996,#18997,#18998,
#18999,#19000,#19001,#19002,#19003,#19004,#19005,#19006,#19007,#19008,#19009,
#19010,#19011,#19012,#19013,#19014,#19015,#19016,#19017,#19018,#19019,#19020,
#19021,#19022,#19023,#19024,#19025,#19026,#19027,#19028,#19029,#19030,#19031,
#19032,#19033,#19034,#19035,#19036,#19037,#19038,#19039,#19040,#19041,#19042,
#19043,#19044,#19045,#19046,#19047,#19048,#19049,#19050,#19051,#19052,#19053,
#19054,#19055,#19056,#19057,#19058,#19059,#19060,#19061,#19062,#19063,#19064,
#19065,#19066,#19067,#19068,#19069,#19070,#19071,#19072,#19073,#19074,#19075,
#19076,#19077,#19078,#19079,#19080,#19081,#19082),.UNSPECIFIED.,.F.,.F.,
(4,2,2,2,2,2,2,2,2,2,2,2,2,2,2,2,2,2,2,2,2,2,2,2,2,2,2,2,2,2,2,2,2,2,2,
2,2,2,2,2,2,2,2,2,2,2,2,2,2,2,2,2,2,2,2,2,2,2,2,2,2,2,2,2,2,2,2,2,2,2,2,
2,2,2,2,2,2,2,2,2,2,2,2,2,2,2,2,2,2,2,2,2,2,2,2,2,2,2,2,2,2,2,2,2,4),(0.000324143214619982,
0.0158771094677429,0.0253256916034115,0.0295631149526927,0.0331209995144121,
0.0369092809154866,0.0416550921416168,0.0509457788737595,0.0784877923858483,
0.106581253516791,0.134349941563318,0.140511989900533,0.143315274440515,
0.145431199113102,0.147928564149414,0.152407811664709,0.17755282354848,
0.187425837957977,0.215085789515885,0.242886023539641,0.249733061851928,
0.253911016914234,0.257725176551781,0.262621503787905,0.270798138512466,
0.320633374637595,0.357196980464997,0.361834460025077,0.364338615408408,
0.366474015537369,0.369232612490268,0.375311223949213,0.41543612103427,
0.446945705212345,0.465043005415902,0.471054562112113,0.475055214859167,
0.478905955056057,0.484351423021017,0.497106441653766,0.54738762045425,
0.575220035847899,0.581388739115619,0.584193354432322,0.586328702210027,
0.588833595523762,0.593346086128498,0.6197635794788,0.628535276753099,0.656623833246853,
0.683846243736795,0.690656446574303,0.694826678539508,0.698643380678667,
0.70355632828705,0.711791100802504,0.760876544034798,0.786716483537455,
0.799777497874279,0.803485626225488,0.805788333016259,0.807968087090028,
0.810679787991711,0.816125831712701,0.856712147270895,0.903051367701181,
0.910541362758302,0.914857263670785,0.91864515240653,0.923384476776052,
0.932643004919074,0.976743445578183,1.00604596927801,1.0154782267772,1.02208292984193,
1.02496480091048,1.02710858112767,1.02956525578479,1.03386303786208,1.0533385937206,
1.09228763610114,1.11353353978246,1.12756660898495,1.133054960024,1.13695227586539,
1.1404826398124,1.14610351218811,1.15997305013599,1.20915166312345,1.23661077063823,
1.24274179985566,1.24553958605232,1.24767431703644,1.25018390355316,1.25471741155012,
1.28211555775354,1.28996158175801,1.31872987310898,1.3363563305562,1.34865284472729,
1.35387436658997,1.35772496048381,1.36180366957232,1.36818631869201,1.38783032955465),
 .UNSPECIFIED.);
#1469=B_SPLINE_CURVE_WITH_KNOTS('',3,(#19083,#19084,#19085,#19086,#19087,
#19088,#19089,#19090,#19091,#19092,#19093,#19094,#19095,#19096,#19097,#19098,
#19099,#19100,#19101,#19102,#19103,#19104,#19105,#19106,#19107,#19108,#19109,
#19110,#19111,#19112,#19113,#19114,#19115,#19116,#19117,#19118,#19119,#19120,
#19121,#19122,#19123,#19124,#19125,#19126,#19127,#19128,#19129,#19130,#19131,
#19132,#19133,#19134,#19135,#19136,#19137,#19138,#19139,#19140,#19141,#19142,
#19143,#19144,#19145,#19146,#19147,#19148,#19149,#19150,#19151,#19152,#19153,
#19154,#19155,#19156,#19157,#19158,#19159,#19160,#19161,#19162,#19163,#19164,
#19165,#19166,#19167,#19168,#19169,#19170,#19171,#19172,#19173,#19174,#19175,
#19176,#19177,#19178,#19179,#19180,#19181,#19182,#19183,#19184,#19185,#19186,
#19187,#19188,#19189,#19190,#19191,#19192,#19193,#19194,#19195,#19196,#19197,
#19198,#19199,#19200,#19201,#19202,#19203,#19204,#19205,#19206,#19207,#19208,
#19209,#19210,#19211,#19212,#19213,#19214,#19215,#19216,#19217,#19218,#19219,
#19220,#19221,#19222,#19223,#19224,#19225,#19226,#19227,#19228,#19229,#19230,
#19231,#19232,#19233,#19234,#19235,#19236,#19237,#19238,#19239,#19240,#19241,
#19242,#19243,#19244,#19245,#19246,#19247,#19248,#19249,#19250,#19251,#19252,
#19253,#19254,#19255,#19256,#19257,#19258,#19259,#19260,#19261,#19262,#19263,
#19264,#19265,#19266,#19267,#19268,#19269,#19270,#19271,#19272,#19273,#19274,
#19275,#19276,#19277,#19278,#19279,#19280,#19281,#19282,#19283,#19284,#19285,
#19286,#19287,#19288,#19289,#19290,#19291,#19292),.UNSPECIFIED.,.F.,.F.,
(4,2,2,2,2,2,2,2,2,2,2,2,2,2,2,2,2,2,2,2,2,2,2,2,2,2,2,2,2,2,2,2,2,2,2,
2,2,2,2,2,2,2,2,2,2,2,2,2,2,2,2,2,2,2,2,2,2,2,2,2,2,2,2,2,2,2,2,2,2,2,2,
2,2,2,2,2,2,2,2,2,2,2,2,2,2,2,2,2,2,2,2,2,2,2,2,2,2,2,2,2,2,2,2,2,4),(1.38776860835863,
1.40398233122755,1.41000183807035,1.41362896188388,1.41751622842159,1.42277942376607,
1.43514507724354,1.45286443649362,1.48147220501137,1.49001685060718,1.51658431760489,
1.52112803959449,1.52365458190256,1.52579170351979,1.52862120717566,1.53483702891505,
1.56290070147281,1.61394052191223,1.62593366204401,1.63074978837543,1.63432506904011,
1.63825192507432,1.6437451301814,1.65759438927064,1.67838678690219,1.71798829944731,
1.73743485000576,1.74172687122125,1.74419674243102,1.74636498010362,1.74929993172342,
1.75611578834237,1.7659331722403,1.79738558949043,1.83850355419817,1.84784905440877,
1.85263353141662,1.85645895418144,1.86082003317611,1.86839750174269,1.91347260255677,
1.95524989945497,1.96118744088172,1.96396570133679,1.96611807457362,1.96868992327123,
1.97357941726164,1.97991658792669,1.99509159111867,2.02349581203877,2.06231521828226,
2.06968847118898,2.07404744963738,2.0778368148891,2.08260649948585,2.09219132972863,
2.10477186058338,2.13832904620017,2.17523617074205,2.18143716845065,2.18423391208206,
2.18639181423807,2.18891630482129,2.19357942337749,2.22942487332542,2.28001356930114,
2.28815621832208,2.29306756991374,2.2969151245303,2.3011526657105,2.30815341316567,
2.33783121018183,2.36407119171349,2.37073182078227,2.3981507716049,2.40271189030694,
2.40524214474599,2.40739899658415,2.41023446382361,2.41648423979278,2.44489287544769,
2.49698879118486,2.50809140785172,2.51316420984523,2.51703500955063,2.52119634034231,
2.52784270954923,2.55223478687431,2.60654278757697,2.61989508290732,2.62378478291468,
2.62614182645868,2.62835137441456,2.63154348302303,2.63999967044271,2.65322071616338,
2.68708746236375,2.71557822445905,2.72780807222084,2.73266290825367,2.73624748959956,
2.74016571088565,2.74404832192756,2.7493056597695,2.77503853942652),
 .UNSPECIFIED.);
#1470=B_SPLINE_CURVE_WITH_KNOTS('',3,(#19298,#19299,#19300,#19301,#19302,
#19303,#19304,#19305,#19306,#19307,#19308,#19309,#19310,#19311,#19312,#19313,
#19314,#19315,#19316,#19317,#19318,#19319,#19320,#19321,#19322,#19323,#19324,
#19325,#19326,#19327,#19328,#19329,#19330,#19331,#19332,#19333,#19334,#19335,
#19336,#19337,#19338,#19339,#19340,#19341,#19342,#19343,#19344,#19345,#19346,
#19347,#19348,#19349,#19350,#19351,#19352,#19353,#19354,#19355,#19356,#19357,
#19358,#19359,#19360,#19361,#19362,#19363,#19364,#19365,#19366,#19367,#19368,
#19369,#19370,#19371,#19372,#19373,#19374,#19375,#19376,#19377,#19378,#19379,
#19380,#19381,#19382,#19383,#19384,#19385,#19386,#19387,#19388,#19389,#19390,
#19391,#19392,#19393,#19394,#19395,#19396,#19397,#19398,#19399,#19400,#19401,
#19402,#19403,#19404,#19405,#19406,#19407,#19408,#19409,#19410,#19411,#19412,
#19413,#19414,#19415,#19416,#19417,#19418,#19419,#19420,#19421,#19422,#19423,
#19424,#19425,#19426,#19427,#19428,#19429,#19430,#19431,#19432,#19433,#19434,
#19435,#19436,#19437,#19438,#19439,#19440,#19441,#19442,#19443,#19444,#19445,
#19446,#19447,#19448,#19449,#19450,#19451,#19452,#19453,#19454,#19455,#19456,
#19457,#19458,#19459,#19460,#19461,#19462,#19463,#19464,#19465,#19466,#19467,
#19468,#19469,#19470,#19471,#19472,#19473,#19474,#19475,#19476,#19477,#19478,
#19479,#19480,#19481,#19482,#19483,#19484,#19485,#19486,#19487,#19488,#19489,
#19490,#19491),.UNSPECIFIED.,.F.,.F.,(4,2,2,2,2,2,2,2,2,2,2,2,2,2,2,2,2,
2,2,2,2,2,2,2,2,2,2,2,2,2,2,2,2,2,2,2,2,2,2,2,2,2,2,2,2,2,2,2,2,2,2,2,2,
2,2,2,2,2,2,2,2,2,2,2,2,2,2,2,2,2,2,2,2,2,2,2,2,2,2,2,2,2,2,2,2,2,2,2,2,
2,2,2,2,2,2,2,4),(1.38751651967754,1.39697591777425,1.42674998314585,1.4702579200917,
1.47953589550948,1.48427962318721,1.48806835250533,1.49238232116074,1.49986148827734,
1.54615730070722,1.58679397815463,1.59223249451174,1.59494253514564,1.59712204235159,
1.59942583509039,1.60313813181305,1.61623976683816,1.64221612717862,1.6911439151196,
1.69939330148544,1.7043106590849,1.70812834945081,1.71229720636026,1.71909955459103,
1.74619760867662,1.77436384398711,1.78258875633297,1.80956214071788,1.81408731392465,
1.81659520388562,1.81873040026365,1.82153132476725,1.82767865010866,1.85529595906221,
1.90492261126032,1.91838594168092,1.92393318028493,1.9278028212278,1.931778455983,
1.93766657364923,1.95470800629132,1.9832413031419,2.02824017418,2.03392619157339,
2.03664117836699,2.03877012997708,2.04134256263214,2.04630781598199,2.08070180057313,
2.13251105184096,2.14052006760041,2.14542138815011,2.14922587314184,2.15344413127749,
2.16047776650624,2.19155381143962,2.23362429189789,2.25116751938539,2.25537199407536,
2.25778342871889,2.25993890114918,2.26290649436243,2.27001912405128,2.28044606894956,
2.31597917370023,2.35549686073998,2.36282374805078,2.36714617676002,2.37089733628049,
2.37560955867643,2.38504086394715,2.39738654447141,2.42993011092691,2.46850666193667,
2.47461557824794,2.47737968713199,2.47951570600553,2.48201615913376,2.48663588685027,
2.52105538985485,2.57357844702098,2.58149697303046,2.5863718984084,2.59017308388314,
2.59419656196975,2.60083417866563,2.6088647789538,2.62524974937419,2.6689731736202,
2.69156590513936,2.69599526701249,2.69848152159372,2.70040503240681,2.70311443853625,
2.70877221380305,2.73186702711985,2.77508623523689),.UNSPECIFIED.);
#1471=B_SPLINE_CURVE_WITH_KNOTS('',3,(#19492,#19493,#19494,#19495),
 .UNSPECIFIED.,.F.,.F.,(4,4),(0.00015374700249208,0.000324143214619982),
 .UNSPECIFIED.);
#1472=B_SPLINE_CURVE_WITH_KNOTS('',3,(#19497,#19498,#19499,#19500),
 .UNSPECIFIED.,.F.,.F.,(4,4),(2.77503853942652,2.77520897093981),
 .UNSPECIFIED.);
#1473=B_SPLINE_CURVE_WITH_KNOTS('',3,(#19501,#19502,#19503,#19504,#19505,
#19506,#19507,#19508,#19509,#19510,#19511,#19512,#19513,#19514,#19515,#19516,
#19517,#19518,#19519,#19520,#19521,#19522,#19523,#19524,#19525,#19526,#19527,
#19528,#19529,#19530,#19531,#19532,#19533,#19534,#19535,#19536,#19537,#19538,
#19539,#19540,#19541,#19542,#19543,#19544,#19545,#19546,#19547,#19548,#19549,
#19550,#19551,#19552,#19553,#19554,#19555,#19556,#19557,#19558,#19559,#19560,
#19561,#19562,#19563,#19564,#19565,#19566,#19567,#19568,#19569,#19570,#19571,
#19572,#19573,#19574,#19575,#19576,#19577,#19578,#19579,#19580,#19581,#19582,
#19583,#19584,#19585,#19586,#19587,#19588,#19589,#19590,#19591,#19592,#19593,
#19594,#19595,#19596,#19597,#19598,#19599,#19600,#19601,#19602,#19603,#19604,
#19605,#19606,#19607,#19608,#19609,#19610,#19611,#19612,#19613,#19614,#19615,
#19616,#19617,#19618,#19619,#19620,#19621,#19622,#19623,#19624,#19625,#19626,
#19627,#19628,#19629,#19630,#19631,#19632,#19633,#19634,#19635,#19636,#19637,
#19638,#19639,#19640,#19641,#19642,#19643,#19644,#19645,#19646,#19647,#19648,
#19649,#19650,#19651,#19652,#19653,#19654,#19655,#19656,#19657,#19658,#19659,
#19660,#19661,#19662,#19663,#19664,#19665,#19666,#19667,#19668,#19669,#19670,
#19671,#19672,#19673,#19674,#19675,#19676,#19677,#19678,#19679,#19680,#19681,
#19682,#19683,#19684,#19685,#19686,#19687,#19688,#19689,#19690,#19691,#19692,
#19693,#19694,#19695,#19696,#19697,#19698,#19699,#19700,#19701,#19702,#19703,
#19704,#19705,#19706,#19707,#19708,#19709,#19710,#19711,#19712,#19713,#19714,
#19715,#19716),.UNSPECIFIED.,.F.,.F.,(4,2,2,2,2,2,2,2,2,2,2,2,2,2,2,2,2,
2,2,2,2,2,2,2,2,2,2,2,2,2,2,2,2,2,2,2,2,2,2,2,2,2,2,2,2,2,2,2,2,2,2,2,2,
2,2,2,2,2,2,2,2,2,2,2,2,2,2,2,2,2,2,2,2,2,2,2,2,2,2,2,2,2,2,2,2,2,2,2,2,
2,2,2,2,2,2,2,2,2,2,2,2,2,2,2,2,2,2,4),(0.000144395392494094,0.0335360417482643,
0.061369564427443,0.0675626175607466,0.0703881121110802,0.0725444079601289,
0.0750822964663496,0.0796765049185713,0.111407318138572,0.146349092280614,
0.162357644088658,0.173765973228149,0.178382268974139,0.178526076332496,
0.178673879658054,0.178826415336729,0.178984514681895,0.179149125689295,
0.17932134022883,0.17938678786255,0.179473112109535,0.179588328256961,0.183377949240674,
0.187737567173298,0.195112746848084,0.23389246083911,0.262199201363727,
0.277437258647108,0.283791911916812,0.288692226521834,0.291266435908779,
0.293418773028459,0.296194430520708,0.302117353072285,0.344260863152019,
0.389019310541182,0.396607313634844,0.400970789500911,0.404796164070481,
0.409577747284325,0.418908453871539,0.461166385467933,0.491726531638866,
0.501394769547792,0.508134262805267,0.5110562327663,0.513222920003422,0.515700240096551,
0.520024840959891,0.540130580129801,0.578664439233278,0.610310550593883,
0.617415996861764,0.621676253185538,0.625518823943701,0.630470554248946,
0.641026657918823,0.693866049261419,0.722504761659807,0.72877777371306,
0.731617667780256,0.733755901598967,0.736275649268416,0.740788762352783,
0.766150521253197,0.77543890823226,0.802937309949103,0.831097905157373,
0.838009753561634,0.842228568539597,0.84608175125631,0.851031595886933,
0.861874126785413,0.914399762147479,0.942939951596952,0.949203423803074,
0.952041677818635,0.954179832078454,0.956700871283743,0.961219443267498,
0.986776090664185,0.995783710226313,1.02297369908458,1.04190942125654,1.05487675843095,
1.06023618084105,1.06413975890095,1.06823147447015,1.07454732996413,1.09340159334891,
1.13795234375634,1.16608935844108,1.17062746374711,1.17312565637463,1.17528832042572,
1.17812601031381,1.18431452134361,1.21904877008705,1.25299440546504,1.26649418136381,
1.27660561404815,1.28147572109749,1.28530962003881,1.28961705449172,1.29694102868511,
1.32920643338237,1.37072333147956,1.38737691891928),.UNSPECIFIED.);
#1474=B_SPLINE_CURVE_WITH_KNOTS('',3,(#19722,#19723,#19724,#19725),
 .UNSPECIFIED.,.F.,.F.,(4,4),(2.77561970906091,2.77582150461351),
 .UNSPECIFIED.);
#1475=B_SPLINE_CURVE_WITH_KNOTS('',3,(#19726,#19727,#19728,#19729,#19730,
#19731,#19732,#19733,#19734,#19735,#19736,#19737,#19738,#19739,#19740,#19741,
#19742,#19743,#19744,#19745,#19746,#19747,#19748,#19749,#19750,#19751,#19752,
#19753,#19754,#19755,#19756,#19757,#19758,#19759,#19760,#19761,#19762,#19763,
#19764,#19765,#19766,#19767,#19768,#19769,#19770,#19771,#19772,#19773,#19774,
#19775,#19776,#19777,#19778,#19779,#19780,#19781,#19782,#19783,#19784,#19785,
#19786,#19787,#19788,#19789,#19790,#19791,#19792,#19793,#19794,#19795,#19796,
#19797,#19798,#19799,#19800,#19801,#19802,#19803,#19804,#19805,#19806,#19807,
#19808,#19809,#19810,#19811,#19812,#19813,#19814,#19815,#19816,#19817,#19818,
#19819,#19820,#19821,#19822,#19823,#19824,#19825,#19826,#19827,#19828,#19829,
#19830,#19831,#19832,#19833,#19834,#19835,#19836,#19837,#19838,#19839,#19840,
#19841,#19842,#19843,#19844,#19845,#19846,#19847,#19848,#19849,#19850,#19851,
#19852,#19853,#19854,#19855,#19856,#19857,#19858,#19859,#19860,#19861,#19862,
#19863,#19864,#19865,#19866,#19867,#19868,#19869,#19870,#19871,#19872,#19873,
#19874,#19875,#19876,#19877,#19878,#19879,#19880,#19881,#19882,#19883,#19884,
#19885,#19886,#19887,#19888,#19889,#19890,#19891,#19892,#19893,#19894,#19895,
#19896,#19897,#19898,#19899,#19900,#19901,#19902,#19903,#19904,#19905,#19906,
#19907,#19908,#19909,#19910,#19911,#19912,#19913,#19914,#19915,#19916,#19917,
#19918,#19919,#19920,#19921,#19922,#19923,#19924,#19925,#19926,#19927,#19928,
#19929,#19930,#19931),.UNSPECIFIED.,.F.,.F.,(4,2,2,2,2,2,2,2,2,2,2,2,2,
2,2,2,2,2,2,2,2,2,2,2,2,2,2,2,2,2,2,2,2,2,2,2,2,2,2,2,2,2,2,2,2,2,2,2,2,
2,2,2,2,2,2,2,2,2,2,2,2,2,2,2,2,2,2,2,2,2,2,2,2,2,2,2,2,2,2,2,2,2,2,2,2,
2,2,2,2,2,2,2,2,2,2,2,2,2,2,2,2,2,4),(9.71563100416002E-5,0.0442115391377216,
0.0498403619130266,0.052544193992351,0.054467119812325,0.0569573303758112,
0.0614045012205749,0.0850904675135822,0.110413415476681,0.137546768762737,
0.154008548489618,0.159852348687565,0.1638186714502,0.167694952161709,0.173279579473492,
0.186949630735342,0.236491329206391,0.263879455827479,0.270003157766796,
0.272799553069537,0.274914888353178,0.277417100515319,0.281917736768463,
0.307862869991328,0.31706669719401,0.345020856809668,0.372414184984056,
0.379235408779519,0.383407942862652,0.387223860995817,0.39213177292575,
0.400348939950123,0.449683153424383,0.486573954653824,0.491273292128384,
0.493790525812396,0.495924322066288,0.498664899479556,0.504643861572882,
0.545721832064817,0.576672083524734,0.594578097553252,0.600567980979266,
0.604564279601765,0.608418276866243,0.613881145752979,0.626768175537875,
0.676926430237138,0.704718044645319,0.710882786761496,0.713686753829517,
0.715822118362307,0.718327633354895,0.722842634984869,0.749359018366637,
0.757095624674673,0.78356992048174,0.803167726698839,0.816431701565958,
0.821805647930899,0.825682406979315,0.829235449743582,0.834983993314114,
0.849675777432851,0.89805882811185,0.925244918677645,0.931348339078943,
0.934141206365647,0.936275621538627,0.938788905744417,0.943338584868203,
0.971860146414204,1.00005701663801,1.03317765885052,1.0403090465185,1.0445484662088,
1.04834879208563,1.05321242907214,1.06109091535175,1.11413457230855,1.14809163688687,
1.1527061547887,1.15520568838248,1.15734211800294,1.16010830675551,1.16622767810195,
1.20468354465209,1.2373388696191,1.24970912155006,1.25915428411731,1.26386948043372,
1.26762120400276,1.27194228850633,1.27926205245912,1.31936774856166,1.35344834228076,
1.36970336138195,1.37367363508361,1.37603406564585,1.37820866887168,1.3808124063889,
1.38746027865211,1.38751651967754),.UNSPECIFIED.);
#1476=B_SPLINE_CURVE_WITH_KNOTS('',3,(#19933,#19934,#19935,#19936,#19937,
#19938,#19939,#19940,#19941,#19942,#19943,#19944,#19945,#19946,#19947,#19948,
#19949,#19950,#19951,#19952,#19953,#19954,#19955,#19956,#19957,#19958,#19959,
#19960,#19961,#19962,#19963,#19964,#19965,#19966,#19967,#19968,#19969,#19970,
#19971,#19972,#19973,#19974,#19975,#19976,#19977,#19978,#19979,#19980,#19981,
#19982,#19983,#19984,#19985,#19986,#19987,#19988,#19989,#19990,#19991,#19992,
#19993,#19994,#19995,#19996,#19997,#19998,#19999,#20000,#20001,#20002,#20003,
#20004,#20005,#20006,#20007,#20008,#20009,#20010,#20011,#20012,#20013,#20014,
#20015,#20016,#20017,#20018,#20019,#20020,#20021,#20022,#20023,#20024,#20025,
#20026,#20027,#20028,#20029,#20030,#20031,#20032,#20033,#20034,#20035,#20036,
#20037,#20038,#20039,#20040,#20041,#20042,#20043,#20044,#20045,#20046,#20047,
#20048,#20049,#20050,#20051,#20052,#20053,#20054,#20055,#20056,#20057,#20058,
#20059,#20060,#20061,#20062,#20063,#20064,#20065,#20066,#20067,#20068,#20069,
#20070,#20071,#20072,#20073,#20074,#20075,#20076,#20077,#20078,#20079,#20080,
#20081,#20082,#20083,#20084,#20085,#20086,#20087,#20088,#20089,#20090,#20091,
#20092,#20093,#20094,#20095,#20096,#20097,#20098,#20099,#20100,#20101,#20102,
#20103,#20104,#20105,#20106,#20107,#20108,#20109,#20110,#20111,#20112,#20113,
#20114,#20115,#20116,#20117,#20118,#20119,#20120,#20121,#20122,#20123,#20124,
#20125,#20126,#20127,#20128,#20129,#20130,#20131,#20132,#20133,#20134,#20135,
#20136,#20137,#20138),.UNSPECIFIED.,.F.,.F.,(4,2,2,2,2,2,2,2,2,2,2,2,2,
2,2,2,2,2,2,2,2,2,2,2,2,2,2,2,2,2,2,2,2,2,2,2,2,2,2,2,2,2,2,2,2,2,2,2,2,
2,2,2,2,2,2,2,2,2,2,2,2,2,2,2,2,2,2,2,2,2,2,2,2,2,2,2,2,2,2,2,2,2,2,2,2,
2,2,2,2,2,2,2,2,2,2,2,2,2,2,2,2,2,4),(1.38737691891928,1.3874301155379,
1.3914573492088,1.39384492406497,1.39604053387784,1.39915262400335,1.40706582796174,
1.41911011093103,1.46839052997284,1.49253621173924,1.49936766779574,1.50356938820404,
1.50742787565361,1.51249962461698,1.52372725511669,1.55880702423526,1.60221336278169,
1.6097216025008,1.61285967553652,1.6150380628634,1.61740839948999,1.62135732076962,
1.63698676263006,1.67293551647641,1.71178010419775,1.71915389687138,1.72351324060164,
1.72730295139313,1.73207310766056,1.74165901626112,1.75424104973819,1.78780305275641,
1.82471080986153,1.83091250474988,1.83370952547598,1.83586762492197,1.83839232643769,
1.84305578568546,1.87889432823297,1.92949981962921,1.93764213707323,1.94255362866528,
1.94640149050478,1.9506395727265,1.95764169067504,1.98733528312913,2.01356105761642,
2.02023943300273,2.04764620826822,2.05220747199305,2.0547378953764,2.05689495014587,
2.05973076117126,2.06598158750037,2.09439769987869,2.1465210700625,2.15774952630424,
2.16276633134876,2.16662882562305,2.17081518356394,2.17757719804094,2.20350621930206,
2.23278606664219,2.23928866115746,2.26801129224337,2.27258950763136,2.2751236102448,
2.27728000500793,2.280109994405,2.28632924461263,2.31442994759481,2.36558496925798,
2.3774981745826,2.38228337249326,2.38585105711518,2.38978468179788,2.39531611658823,
2.40942752150695,2.43079179498945,2.46969900118903,2.48892417938543,2.49320480741984,
2.49567197196525,2.49784062859814,2.50077990656431,2.50762204299482,2.51749086542158,
2.54926025779796,2.58988411650958,2.59927833908641,2.60407258898838,2.6078985498712,
2.6122524023739,2.61801273761323,2.64168576507317,2.67698879724251,2.70873406769311,
2.71332734559176,2.71586473423071,2.71802059145565,2.72084553106778,2.72703735494925,
2.77453256021917),.UNSPECIFIED.);
#1477=B_SPLINE_CURVE_WITH_KNOTS('',3,(#20139,#20140,#20141,#20142),
 .UNSPECIFIED.,.F.,.F.,(4,4),(0.000109266196132223,0.0003121541379522),
 .UNSPECIFIED.);
#1478=B_SPLINE_CURVE_WITH_KNOTS('',3,(#20147,#20148,#20149,#20150,#20151,
#20152,#20153,#20154,#20155,#20156,#20157,#20158,#20159,#20160,#20161,#20162,
#20163,#20164,#20165,#20166,#20167,#20168,#20169,#20170,#20171,#20172,#20173,
#20174,#20175,#20176,#20177,#20178,#20179,#20180,#20181,#20182,#20183,#20184,
#20185,#20186,#20187,#20188,#20189,#20190,#20191,#20192,#20193,#20194,#20195,
#20196,#20197,#20198,#20199,#20200,#20201,#20202,#20203,#20204,#20205,#20206,
#20207,#20208,#20209,#20210,#20211,#20212,#20213,#20214,#20215,#20216,#20217,
#20218,#20219,#20220,#20221,#20222,#20223,#20224,#20225,#20226,#20227,#20228,
#20229,#20230,#20231,#20232,#20233,#20234,#20235,#20236,#20237,#20238,#20239,
#20240,#20241,#20242,#20243,#20244,#20245,#20246,#20247,#20248,#20249,#20250,
#20251,#20252,#20253,#20254,#20255,#20256,#20257,#20258,#20259,#20260,#20261,
#20262,#20263,#20264,#20265,#20266,#20267,#20268,#20269,#20270,#20271,#20272,
#20273,#20274,#20275,#20276,#20277,#20278,#20279,#20280,#20281,#20282,#20283,
#20284,#20285,#20286,#20287,#20288,#20289,#20290,#20291,#20292,#20293,#20294,
#20295,#20296,#20297,#20298,#20299,#20300,#20301,#20302,#20303,#20304,#20305,
#20306,#20307,#20308,#20309,#20310,#20311,#20312,#20313,#20314,#20315,#20316,
#20317,#20318,#20319,#20320,#20321,#20322,#20323,#20324,#20325,#20326,#20327,
#20328,#20329,#20330,#20331,#20332,#20333,#20334,#20335,#20336,#20337,#20338,
#20339,#20340,#20341,#20342,#20343,#20344,#20345,#20346,#20347,#20348),
 .UNSPECIFIED.,.F.,.F.,(4,2,2,2,2,2,2,2,2,2,2,2,2,2,2,2,2,2,2,2,2,2,2,2,
2,2,2,2,2,2,2,2,2,2,2,2,2,2,2,2,2,2,2,2,2,2,2,2,2,2,2,2,2,2,2,2,2,2,2,2,
2,2,2,2,2,2,2,2,2,2,2,2,2,2,2,2,2,2,2,2,2,2,2,2,2,2,2,2,2,2,2,2,2,2,2,2,
2,2,2,2,4),(1.38831186095198,1.39300679174099,1.39654302199116,1.40043426204388,
1.40589020757036,1.41970332207125,1.4404688199864,1.48145615898468,1.49978162807593,
1.50398918509946,1.50642536965992,1.50857376329047,1.51149230864179,1.51831186933442,
1.5281609251754,1.55992875436192,1.60077237109824,1.61008898947415,1.61484002974374,
1.61862863618847,1.62293605180366,1.63038726635909,1.67615638853852,1.71745784178709,
1.72341109212626,1.72614681219018,1.72828001189852,1.73080036662568,1.73551531377499,
1.77325566367512,1.82162740626428,1.82990849016319,1.83483412721202,1.83865220559887,
1.84281541571348,1.84959467519759,1.87636547945818,1.90494559773848,1.91371259005802,
1.94009986353888,1.94461079538658,1.94711513331963,1.94925020731962,1.95205475132837,
1.9582242477521,1.98606963200391,2.03637985295433,2.04912129632138,2.05456455030475,
2.05841449522715,2.06241497696242,2.06842757892544,2.08653980046283,2.11809508441971,
2.15809186918112,2.16417410500149,2.16693308586477,2.16906823511573,2.17157139552823,
2.17620537796885,2.21228932278736,2.26270968351192,2.2708424605116,2.27572586391455,
2.27953766902553,2.28372089205676,2.29059479451118,2.31884602377331,2.34627971190087,
2.35599762925622,2.38096676790436,2.38544021256849,2.38793599811848,2.39005166421448,
2.39285605519561,2.39902598003031,2.42688019803517,2.47721860213668,2.48992130061587,
2.49535876101637,2.49920726476822,2.50320853121849,2.50922679624455,2.52739391095364,
2.55911443388781,2.59886794325313,2.60494773483509,2.60770603859043,2.60984086209071,
2.6123438830557,2.6169781753519,2.63104405979159,2.66597052296919,2.70614065549259,
2.71350533986767,2.71783525593226,2.72158400700398,2.72628160818939,2.73133113198888,
2.74446638635469,2.77561970906091),.UNSPECIFIED.);
#1479=B_SPLINE_CURVE_WITH_KNOTS('',3,(#20349,#20350,#20351,#20352,#20353,
#20354,#20355,#20356,#20357,#20358,#20359,#20360,#20361,#20362,#20363,#20364,
#20365,#20366,#20367,#20368,#20369,#20370,#20371,#20372,#20373,#20374,#20375,
#20376,#20377,#20378,#20379,#20380,#20381,#20382,#20383,#20384,#20385,#20386,
#20387,#20388,#20389,#20390,#20391,#20392,#20393,#20394,#20395,#20396,#20397,
#20398,#20399,#20400,#20401,#20402,#20403,#20404,#20405,#20406,#20407,#20408,
#20409,#20410,#20411,#20412,#20413,#20414,#20415,#20416,#20417,#20418,#20419,
#20420,#20421,#20422,#20423,#20424,#20425,#20426,#20427,#20428,#20429,#20430,
#20431,#20432,#20433,#20434,#20435,#20436,#20437,#20438,#20439,#20440,#20441,
#20442,#20443,#20444,#20445,#20446,#20447,#20448,#20449,#20450,#20451,#20452,
#20453,#20454,#20455,#20456,#20457,#20458,#20459,#20460,#20461,#20462,#20463,
#20464,#20465,#20466,#20467,#20468,#20469,#20470,#20471,#20472,#20473,#20474,
#20475,#20476,#20477,#20478,#20479,#20480,#20481,#20482,#20483,#20484,#20485,
#20486,#20487,#20488,#20489,#20490,#20491,#20492,#20493,#20494,#20495,#20496,
#20497,#20498,#20499,#20500,#20501,#20502,#20503,#20504,#20505,#20506,#20507,
#20508,#20509,#20510,#20511,#20512,#20513,#20514,#20515,#20516,#20517,#20518,
#20519,#20520,#20521,#20522,#20523,#20524,#20525,#20526,#20527,#20528,#20529,
#20530,#20531,#20532,#20533,#20534,#20535,#20536,#20537,#20538,#20539,#20540,
#20541,#20542,#20543,#20544,#20545,#20546,#20547,#20548,#20549,#20550),
 .UNSPECIFIED.,.F.,.F.,(4,2,2,2,2,2,2,2,2,2,2,2,2,2,2,2,2,2,2,2,2,2,2,2,
2,2,2,2,2,2,2,2,2,2,2,2,2,2,2,2,2,2,2,2,2,2,2,2,2,2,2,2,2,2,2,2,2,2,2,2,
2,2,2,2,2,2,2,2,2,2,2,2,2,2,2,2,2,2,2,2,2,2,2,2,2,2,2,2,2,2,2,2,2,2,2,2,
2,2,2,2,4),(0.0003121541379522,0.0392060648077781,0.0446675046569061,0.0496673000307714,
0.0535160972622554,0.0577520518454449,0.0647432384458444,0.0911778289075277,
0.133032959052139,0.155101639846516,0.159541399983137,0.162018520179388,
0.164185453949274,0.167057699983818,0.173688012089452,0.235750831895649,
0.261197565219785,0.267924910902226,0.272103899441255,0.275968985478701,
0.281002551644563,0.292328410019673,0.344321573823604,0.372693315149619,
0.378939839155464,0.381774885497033,0.383931901223479,0.386462883074088,
0.391026615386072,0.418547368976696,0.425122557310079,0.451354895579256,
0.481068496777416,0.488072081891223,0.492310490273833,0.496158281403396,
0.501069178096886,0.509209322586512,0.559802772661404,0.595619079568649,
0.600281738946522,0.602806255127853,0.604964335404705,0.607761549496186,
0.613964409495356,0.650889101759488,0.684466565962733,0.697052137343631,
0.706639319739503,0.711409643299882,0.71519925888635,0.719558243126607,
0.726930828848786,0.765721436101874,0.79407866111338,0.809278784195776,
0.815623040489877,0.820517129394222,0.823090020178777,0.825242423845138,
0.828019670217397,0.833951279785584,0.875894075120533,0.920832535636686,
0.928423527251669,0.932787580920352,0.936612796362153,0.941393303603974,
0.950719072180697,0.993249719498709,1.02360446460572,1.03323781842868,1.03995921578549,
1.04287803864191,1.04504429410948,1.04752331289461,1.05185555840349,1.07212314259831,
1.11223388723409,1.13219936377714,1.14566068705711,1.15109583943171,1.15501230397639,
1.15908022177954,1.16528432023797,1.18311342917425,1.22854734098628,1.25703573554775,
1.26158218340804,1.26408198040801,1.26624405760627,1.26907845898553,1.27525055637446,
1.30916774530616,1.34370678335913,1.35733268068435,1.36751508693558,1.37239811094477,
1.37623299596259,1.38053196284411,1.38775902368221),.UNSPECIFIED.);
#1480=B_SPLINE_CURVE_WITH_KNOTS('',3,(#20555,#20556,#20557,#20558,#20559,
#20560,#20561,#20562,#20563,#20564,#20565,#20566,#20567,#20568,#20569,#20570,
#20571,#20572,#20573,#20574,#20575,#20576,#20577,#20578,#20579,#20580,#20581,
#20582,#20583,#20584,#20585,#20586,#20587,#20588,#20589,#20590,#20591,#20592,
#20593,#20594,#20595,#20596,#20597,#20598,#20599,#20600,#20601,#20602,#20603,
#20604,#20605,#20606,#20607,#20608,#20609,#20610,#20611,#20612,#20613,#20614,
#20615,#20616,#20617,#20618,#20619,#20620,#20621,#20622,#20623,#20624,#20625,
#20626,#20627,#20628,#20629,#20630,#20631,#20632,#20633,#20634,#20635,#20636,
#20637,#20638,#20639,#20640,#20641,#20642,#20643,#20644,#20645,#20646,#20647,
#20648,#20649,#20650,#20651,#20652,#20653,#20654,#20655,#20656,#20657,#20658,
#20659,#20660,#20661,#20662,#20663,#20664,#20665,#20666,#20667,#20668,#20669,
#20670,#20671,#20672,#20673,#20674,#20675,#20676,#20677,#20678,#20679,#20680,
#20681,#20682,#20683,#20684,#20685,#20686,#20687,#20688,#20689,#20690,#20691,
#20692,#20693,#20694,#20695,#20696,#20697,#20698,#20699,#20700,#20701,#20702,
#20703,#20704,#20705,#20706,#20707,#20708,#20709,#20710,#20711,#20712,#20713,
#20714,#20715,#20716,#20717,#20718,#20719,#20720,#20721,#20722,#20723,#20724,
#20725,#20726,#20727,#20728,#20729,#20730,#20731,#20732,#20733,#20734,#20735,
#20736,#20737,#20738,#20739,#20740,#20741,#20742,#20743,#20744,#20745,#20746,
#20747,#20748,#20749,#20750,#20751,#20752,#20753,#20754,#20755,#20756,#20757,
#20758),.UNSPECIFIED.,.F.,.F.,(4,2,2,2,2,2,2,2,2,2,2,2,2,2,2,2,2,2,2,2,
2,2,2,2,2,2,2,2,2,2,2,2,2,2,2,2,2,2,2,2,2,2,2,2,2,2,2,2,2,2,2,2,2,2,2,2,
2,2,2,2,2,2,2,2,2,2,2,2,2,2,2,2,2,2,2,2,2,2,2,2,2,2,2,2,2,2,2,2,2,2,2,2,
2,2,2,2,2,2,2,2,2,4),(0.000678815151983969,0.0135545168336831,0.0611711635650268,
0.068785317826121,0.0731324065597843,0.0769245232162855,0.0816391428814896,
0.0907550633644243,0.138107932867606,0.164894831513744,0.173869349804587,
0.180121182227087,0.182858732059293,0.182882308764285,0.182906020021552,
0.182929872685781,0.182953873785344,0.185107628733336,0.187548711308559,
0.191771062746313,0.210316627205456,0.249902635531842,0.275918125146367,
0.286838308381199,0.291827560649767,0.295644420915677,0.299820848739743,
0.306655115126896,0.331073289699422,0.372380459411266,0.395378045064019,
0.401024954084468,0.403732281417403,0.405655074684526,0.408140872750035,
0.412572955470426,0.435251989868403,0.474367051463985,0.503042478106631,
0.509939776856481,0.514126327195829,0.517934079849689,0.522802444066866,
0.5308876829993,0.581852597701758,0.616906110202894,0.621887898700021,0.624462163046354,
0.626589763799827,0.629298927888174,0.634955291839129,0.680245073914239,
0.716418150197959,0.72765365234876,0.732697470407692,0.73652112822304,0.740670945791758,
0.747384446099101,0.770356600533664,0.812406110647427,0.836112817095739,
0.841841354491834,0.844564796364056,0.846490187752058,0.848967402473689,
0.853356319456151,0.875118581695272,0.91509631169618,0.943880083691493,
0.950787015088377,0.954977691669364,0.958788172403765,0.963658710019169,
0.971744933331961,1.0226887538672,1.05796650011253,1.06280686867967,1.06535325266426,
1.06748353352322,1.07022964560481,1.07608263647188,1.11922003380121,1.14886726323934,
1.16631302846943,1.17224844112551,1.17623290450731,1.18009378298713,1.18559813203675,
1.19879761270301,1.24865043037431,1.27633816396436,1.28249174220238,1.28529327720863,
1.28740887351293,1.28990710584242,1.2943903513606,1.31968644789017,1.32944596727245,
1.35724538243593,1.3755962880985,1.38825411328145,1.38831186095198),
 .UNSPECIFIED.);
#1481=B_SPLINE_CURVE_WITH_KNOTS('',3,(#20759,#20760,#20761,#20762,#20763,
#20764,#20765,#20766,#20767,#20768,#20769,#20770,#20771,#20772,#20773,#20774,
#20775,#20776,#20777,#20778,#20779,#20780,#20781,#20782,#20783,#20784,#20785,
#20786,#20787,#20788,#20789,#20790,#20791,#20792,#20793,#20794,#20795,#20796,
#20797,#20798,#20799,#20800,#20801,#20802,#20803,#20804,#20805,#20806,#20807,
#20808,#20809,#20810,#20811,#20812,#20813,#20814,#20815,#20816,#20817,#20818,
#20819,#20820,#20821,#20822,#20823,#20824,#20825,#20826,#20827,#20828,#20829,
#20830,#20831,#20832,#20833,#20834,#20835,#20836,#20837,#20838,#20839,#20840,
#20841,#20842,#20843,#20844,#20845,#20846,#20847,#20848,#20849,#20850,#20851,
#20852,#20853,#20854,#20855,#20856,#20857,#20858,#20859,#20860,#20861,#20862,
#20863,#20864,#20865,#20866,#20867,#20868,#20869,#20870,#20871,#20872,#20873,
#20874,#20875,#20876,#20877,#20878,#20879,#20880,#20881,#20882,#20883,#20884,
#20885,#20886,#20887,#20888,#20889,#20890,#20891,#20892,#20893,#20894,#20895,
#20896,#20897,#20898,#20899,#20900,#20901,#20902,#20903,#20904,#20905,#20906,
#20907,#20908,#20909,#20910,#20911,#20912,#20913,#20914,#20915,#20916,#20917,
#20918,#20919,#20920,#20921,#20922,#20923,#20924,#20925,#20926,#20927,#20928,
#20929,#20930,#20931,#20932,#20933,#20934,#20935,#20936,#20937,#20938,#20939,
#20940,#20941,#20942,#20943,#20944,#20945,#20946,#20947,#20948,#20949,#20950,
#20951,#20952,#20953,#20954,#20955,#20956),.UNSPECIFIED.,.F.,.F.,(4,2,2,
2,2,2,2,2,2,2,2,2,2,2,2,2,2,2,2,2,2,2,2,2,2,2,2,2,2,2,2,2,2,2,2,2,2,2,2,
2,2,2,2,2,2,2,2,2,2,2,2,2,2,2,2,2,2,2,2,2,2,2,2,2,2,2,2,2,2,2,2,2,2,2,2,
2,2,2,2,2,2,2,2,2,2,2,2,2,2,2,2,2,2,2,2,2,2,2,4),(1.38775902368221,1.38781776182658,
1.42374712644421,1.44656466883186,1.47725592566392,1.48184182100099,1.48437775373741,
1.48653408692494,1.48936189250973,1.4955684715692,1.52354014058484,1.5743016397036,
1.58655876987782,1.59141817215752,1.59500391331784,1.59892126356546,1.60436186837484,
1.6178600672121,1.63790158758803,1.67939432613439,1.69823860898585,1.70249993736081,
1.70496283476324,1.70713275010269,1.71008047812879,1.71697163238382,1.72693585378422,
1.7592944092514,1.79921455801226,1.80858355382043,1.81337288105224,1.81719873071807,
1.82155657174777,1.82911871885237,1.87480171672228,1.91592657861927,1.92191200258405,
1.92469921463186,1.92685229858058,1.92941758616548,1.93427494944176,1.97198056740512,
2.02004914483874,2.02837280105711,2.03333556913017,2.03719035569486,2.04140239587713,
2.04828353353468,2.07596800873124,2.10365331108819,2.11318871315535,2.13859625795144,
2.14310994963642,2.14562968799694,2.14776750608049,2.15060643345803,2.15687600065352,
2.18548625751486,2.23821952923997,2.24875309821462,2.25371951467301,2.25757419174051,
2.26178313377423,2.26865234096921,2.29616551954454,2.3239479129378,2.33320957629621,
2.35896443119481,2.36348692724304,2.36600838321833,2.36814574978579,2.37098143808224,
2.37723304271062,2.40566134282915,2.45782418080421,2.46901476055243,2.47402475321731,
2.47788594508415,2.4820748041927,2.48884966745186,2.51496670806313,2.54395636565273,
2.57667707315928,2.58285036238085,2.58568481360637,2.5878469686997,2.59018570910623,
2.59419563317155,2.59933803021425,2.61043454439731,2.64995370249589,2.68430283169248,
2.69168464554774,2.69600421555137,2.69945254035975,2.70411374928957,2.713144566244,
2.74595194315684,2.77514791930297),.UNSPECIFIED.);
#1482=B_SPLINE_CURVE_WITH_KNOTS('',3,(#20962,#20963,#20964,#20965,#20966,
#20967,#20968,#20969,#20970,#20971,#20972,#20973,#20974,#20975,#20976,#20977,
#20978,#20979,#20980,#20981,#20982,#20983,#20984,#20985,#20986,#20987,#20988,
#20989,#20990,#20991,#20992,#20993,#20994,#20995,#20996,#20997,#20998,#20999,
#21000,#21001,#21002,#21003,#21004,#21005,#21006,#21007,#21008,#21009,#21010,
#21011,#21012,#21013,#21014,#21015,#21016,#21017,#21018,#21019,#21020,#21021,
#21022,#21023,#21024,#21025,#21026,#21027,#21028,#21029,#21030,#21031,#21032,
#21033,#21034,#21035,#21036,#21037,#21038,#21039,#21040,#21041,#21042,#21043,
#21044,#21045,#21046,#21047,#21048,#21049,#21050,#21051,#21052,#21053,#21054,
#21055,#21056,#21057,#21058,#21059,#21060,#21061,#21062,#21063,#21064,#21065,
#21066,#21067,#21068,#21069,#21070,#21071,#21072,#21073,#21074,#21075,#21076,
#21077,#21078,#21079,#21080,#21081,#21082,#21083,#21084,#21085,#21086,#21087,
#21088,#21089,#21090,#21091,#21092,#21093,#21094,#21095,#21096,#21097,#21098,
#21099,#21100,#21101,#21102,#21103,#21104,#21105,#21106,#21107,#21108,#21109,
#21110,#21111),.UNSPECIFIED.,.F.,.F.,(4,2,2,2,2,2,2,2,2,2,2,2,2,2,2,2,2,
2,2,2,2,2,2,2,2,2,2,2,2,2,2,2,2,2,2,2,2,2,2,2,2,2,2,2,2,2,2,2,2,2,2,2,2,
2,2,2,2,2,2,2,2,2,2,2,2,2,2,2,2,2,2,2,2,2,4),(-0.875860537968119,-0.875799606618078,
-0.873773553177765,-0.87149818754001,-0.867965548349446,-0.856448447729897,
-0.833732991281093,-0.799161880436857,-0.7917731182112,-0.787046992948174,
-0.783221389412492,-0.778784941286976,-0.770787706902226,-0.743813012619747,
-0.714534998448861,-0.702085142336867,-0.698351752718789,-0.696031594790346,
-0.69375930589405,-0.690263543538742,-0.679161910350972,-0.657871591932514,
-0.621533610623069,-0.614210117781182,-0.609499808353657,-0.605670060507595,
-0.601209419402849,-0.593111931121542,-0.565409806606647,-0.534782653391671,
-0.524105848956321,-0.520558385012711,-0.518505374981075,-0.51627358885697,
-0.512907823993746,-0.502797067005756,-0.48459875051324,-0.442538530977189,
-0.434986466049484,-0.430616436242226,-0.426812791679861,-0.422068984773143,
-0.412400073099503,-0.387174926820729,-0.356300434820293,-0.3459572784027,
-0.342459350338071,-0.340421463188156,-0.338162941301972,-0.334728984138968,
-0.324197280876602,-0.304782797605587,-0.265008585893149,-0.257163635100863,
-0.2526991700981,-0.248854362295849,-0.244110087804886,-0.234613342481773,
-0.20863912342285,-0.176848272932624,-0.167766002900717,-0.164404377275654,
-0.162165968466191,-0.159749783833764,-0.155725018712719,-0.138391996764361,
-0.116508694397701,-0.0871482397750525,-0.0803511701143885,-0.076130777917414,
-0.0722018029327749,-0.066922343944156,-0.0544148358211864,-0.0357514952089097,
-8.33018978494207E-5),.UNSPECIFIED.);
#1483=B_SPLINE_CURVE_WITH_KNOTS('',3,(#21114,#21115,#21116,#21117,#21118,
#21119,#21120,#21121,#21122,#21123,#21124,#21125,#21126,#21127,#21128,#21129,
#21130,#21131,#21132,#21133,#21134,#21135,#21136,#21137,#21138,#21139,#21140,
#21141,#21142,#21143,#21144,#21145,#21146,#21147,#21148,#21149,#21150,#21151,
#21152,#21153,#21154,#21155,#21156,#21157,#21158,#21159,#21160,#21161,#21162,
#21163,#21164,#21165,#21166,#21167,#21168,#21169,#21170,#21171,#21172,#21173,
#21174,#21175,#21176,#21177,#21178,#21179,#21180,#21181,#21182,#21183,#21184,
#21185,#21186,#21187,#21188,#21189,#21190,#21191,#21192,#21193,#21194,#21195,
#21196,#21197,#21198,#21199,#21200,#21201,#21202,#21203,#21204,#21205,#21206,
#21207,#21208,#21209,#21210,#21211,#21212,#21213,#21214,#21215,#21216,#21217,
#21218,#21219,#21220,#21221,#21222,#21223,#21224,#21225,#21226,#21227,#21228,
#21229,#21230,#21231,#21232,#21233,#21234,#21235,#21236,#21237,#21238,#21239,
#21240,#21241,#21242,#21243,#21244,#21245,#21246,#21247,#21248,#21249,#21250,
#21251,#21252,#21253,#21254,#21255),.UNSPECIFIED.,.F.,.F.,(4,3,3,3,3,3,
3,3,3,3,3,3,3,3,3,3,3,3,3,3,3,3,3,3,3,3,3,3,3,3,3,3,3,3,3,3,3,3,3,3,3,3,
3,3,3,3,3,4),(16.7019922841306,16.8021818348996,16.8124544772726,16.9234210411684,
17.033796869599,17.1441744311209,17.2545854631975,17.3659858445079,17.4766375907132,
17.5884122895762,17.6885982648488,17.7001869884391,17.7002311104944,17.7964751471802,
17.8072802155964,17.9128977895231,17.9186679002403,18.0254288144202,18.1321132984658,
18.2387615669814,18.3454137772225,18.4521802784855,18.5590147146697,18.6591545584869,
18.6660336585631,18.6983816927476,18.6984356183394,18.7948863424963,18.8065090728564,
18.9177674883813,19.025595407644,19.1333563054358,19.2410888397907,19.3488316227747,
19.4566913005886,19.5646218816293,19.6655852004633,19.6727314597256,19.6965763970561,
19.6966231841011,19.7936651766023,19.8047706499335,19.912813978709,20.0207451306855,
20.1286177204737,20.2364557658273,20.3443346961532,20.3930532338378),
 .UNSPECIFIED.);
#1484=B_SPLINE_CURVE_WITH_KNOTS('',3,(#21260,#21261,#21262,#21263,#21264,
#21265,#21266,#21267,#21268,#21269,#21270,#21271,#21272,#21273,#21274,#21275,
#21276,#21277,#21278,#21279,#21280,#21281,#21282,#21283,#21284,#21285,#21286,
#21287,#21288,#21289,#21290,#21291,#21292,#21293,#21294,#21295,#21296,#21297,
#21298,#21299,#21300,#21301,#21302,#21303,#21304,#21305,#21306,#21307,#21308,
#21309,#21310,#21311,#21312,#21313,#21314,#21315,#21316,#21317,#21318,#21319,
#21320,#21321,#21322,#21323,#21324,#21325,#21326,#21327,#21328,#21329,#21330,
#21331,#21332,#21333,#21334,#21335,#21336,#21337,#21338,#21339,#21340,#21341,
#21342,#21343,#21344,#21345,#21346,#21347,#21348,#21349,#21350,#21351,#21352,
#21353,#21354,#21355,#21356,#21357,#21358,#21359,#21360,#21361,#21362,#21363,
#21364,#21365,#21366,#21367,#21368,#21369,#21370,#21371,#21372,#21373,#21374,
#21375,#21376,#21377,#21378,#21379,#21380,#21381,#21382,#21383,#21384,#21385,
#21386,#21387,#21388,#21389,#21390,#21391,#21392,#21393,#21394,#21395,#21396,
#21397,#21398,#21399,#21400,#21401,#21402,#21403,#21404,#21405,#21406,#21407,
#21408,#21409,#21410,#21411,#21412,#21413,#21414,#21415,#21416,#21417,#21418,
#21419,#21420,#21421,#21422,#21423,#21424,#21425,#21426,#21427,#21428,#21429,
#21430,#21431,#21432,#21433,#21434,#21435,#21436,#21437,#21438,#21439,#21440,
#21441,#21442,#21443),.UNSPECIFIED.,.F.,.F.,(4,2,2,2,2,2,2,2,2,2,2,2,2,
2,2,2,2,2,2,2,2,2,2,2,2,2,2,2,2,2,2,2,2,2,2,2,2,2,2,2,2,2,2,2,2,2,2,2,2,
2,2,2,2,2,2,2,2,2,2,2,2,2,2,2,2,2,2,2,2,2,2,2,2,2,2,2,2,2,2,2,2,2,2,2,2,
2,2,2,2,2,2,4),(-1.99499716658925,-1.96752270825511,-1.94735063860436,-1.9432359106537,
-1.94083476043791,-1.93864780433138,-1.93596208580319,-1.92934417914976,
-1.8905985110623,-1.8722417129216,-1.85992088737411,-1.85471003307461,-1.8508313424147,
-1.84666657370522,-1.83997068590978,-1.81348594212233,-1.78232516918049,
-1.77318699572475,-1.76683405113085,-1.76399298440067,-1.76183078296909,
-1.75923191431716,-1.75432223774033,-1.71877759529623,-1.68657481614049,
-1.67927563000575,-1.67498453647151,-1.67114167156058,-1.66619958340817,
-1.65552021073062,-1.61175799810463,-1.59818907533202,-1.58980992138503,
-1.58665154432093,-1.58444856108206,-1.58202640779601,-1.57781376053967,
-1.55697423009811,-1.50949969125568,-1.50186736047801,-1.49746427033655,
-1.49363844392233,-1.48887447161339,-1.47918665538803,-1.4540281706685,
-1.42324846697106,-1.41279424097747,-1.40927380511322,-1.40722622457644,
-1.40497445531411,-1.40155505405732,-1.39109638873522,-1.37187045168249,
-1.33199521259349,-1.32420786483485,-1.31977091427651,-1.31594741940937,
-1.31122721591586,-1.30177611565075,-1.27091861601456,-1.2380028042242,
-1.23287399570558,-1.23022887746032,-1.2282859390128,-1.22561845713784,
-1.22021226502215,-1.19806621687394,-1.15657997283186,-1.14740409230815,
-1.14267694825044,-1.13885217487448,-1.13441853589904,-1.12643178956738,
-1.09953739031325,-1.07044095700247,-1.05772019663939,-1.05396507648837,
-1.05164182429368,-1.04938381387754,-1.04592827264721,-1.03512785458699,
-1.01482501961887,-0.976708412160299,-0.969463684150646,-0.964782683476268,
-0.960964021124115,-0.956502357916562,-0.948363876558926,-0.92025785255302,
-0.888782192695983,-0.879208177009835,-0.875860537968119),.UNSPECIFIED.);
#1485=B_SPLINE_CURVE_WITH_KNOTS('',3,(#21444,#21445,#21446,#21447,#21448,
#21449,#21450,#21451,#21452,#21453,#21454,#21455,#21456,#21457,#21458,#21459,
#21460,#21461,#21462,#21463,#21464,#21465,#21466,#21467,#21468,#21469,#21470,
#21471,#21472,#21473,#21474,#21475,#21476,#21477,#21478,#21479,#21480,#21481,
#21482,#21483,#21484,#21485,#21486,#21487,#21488,#21489,#21490,#21491,#21492,
#21493,#21494,#21495,#21496,#21497,#21498,#21499,#21500,#21501,#21502,#21503,
#21504,#21505,#21506,#21507,#21508,#21509,#21510,#21511,#21512,#21513,#21514,
#21515,#21516,#21517,#21518,#21519,#21520,#21521,#21522,#21523,#21524,#21525,
#21526,#21527,#21528,#21529,#21530,#21531,#21532,#21533,#21534,#21535,#21536,
#21537,#21538,#21539,#21540,#21541,#21542,#21543,#21544,#21545,#21546,#21547,
#21548,#21549,#21550,#21551,#21552,#21553,#21554,#21555,#21556,#21557,#21558,
#21559,#21560,#21561,#21562,#21563,#21564,#21565,#21566,#21567,#21568,#21569,
#21570,#21571,#21572,#21573,#21574,#21575,#21576,#21577,#21578,#21579,#21580,
#21581,#21582,#21583,#21584,#21585,#21586,#21587,#21588,#21589,#21590,#21591,
#21592,#21593,#21594,#21595,#21596,#21597,#21598,#21599,#21600,#21601,#21602,
#21603,#21604,#21605,#21606,#21607,#21608,#21609,#21610,#21611,#21612,#21613,
#21614,#21615,#21616,#21617,#21618,#21619,#21620,#21621,#21622,#21623,#21624,
#21625,#21626,#21627,#21628,#21629,#21630,#21631),.UNSPECIFIED.,.F.,.F.,
(4,2,2,2,2,2,2,2,2,2,2,2,2,2,2,2,2,2,2,2,2,2,2,2,2,2,2,2,2,2,2,2,2,2,2,
2,2,2,2,2,2,2,2,2,2,2,2,2,2,2,2,2,2,2,2,2,2,2,2,2,2,2,2,2,2,2,2,2,2,2,2,
2,2,2,2,2,2,2,2,2,2,2,2,2,2,2,2,2,2,2,2,2,2,4),(-5.59315610037617,-5.55336009091651,
-5.54468070666692,-5.54149575826921,-5.53930355215932,-5.53694214376124,
-5.53290593997252,-5.51564082705649,-5.48516821989026,-5.46958897838822,
-5.46199122264363,-5.45571624027886,-5.45183829629559,-5.44804344453449,
-5.44313686827759,-5.43206746069107,-5.39235075299744,-5.37067543905196,
-5.36535666667643,-5.36273451778536,-5.3608201428546,-5.35821291898656,
-5.35302769445264,-5.32043304297661,-5.28490221519477,-5.27799207685714,
-5.27380635635698,-5.26998139760904,-5.26503810849382,-5.25388108299712,
-5.21458055505209,-5.19314176132561,-5.18783107528596,-5.18519453495156,
-5.18326905299212,-5.18064249491269,-5.17536672417524,-5.13521978947001,
-5.10917482210811,-5.10133472572026,-5.09695938027789,-5.09317362824814,
-5.08848166764673,-5.08111969262822,-5.04668957869126,-5.02380202938147,
-5.01598141826372,-5.01032649433526,-5.00762902801662,-5.00549607300724,
-5.00283538453111,-4.99736863056442,-4.9711948142544,-4.94608375823654,
-4.92778764252021,-4.92186448637815,-4.91789012705217,-4.91401980341187,
-4.90931936558815,-4.8976438120184,-4.85898282298198,-4.83771786023274,
-4.83243255025401,-4.82980711646114,-4.82788687276963,-4.82526442917046,
-4.82000164325571,-4.77977013837314,-4.75374368839018,-4.74590586747846,
-4.74153148252857,-4.73774643581759,-4.73305518618399,-4.72569380318942,
-4.69152347916303,-4.66849914427294,-4.66065422490463,-4.65498618095219,
-4.65228564625593,-4.65015133546778,-4.64748991070208,-4.64202587343494,
-4.61469886284387,-4.57810890277073,-4.56907203287847,-4.56446021409638,
-4.56104690657797,-4.55674919128219,-4.5494722161337,-4.50572686508456,
-4.48854084273066,-4.47879510090985,-4.47547992283627,-4.4747574653027),
 .UNSPECIFIED.);
#1486=B_SPLINE_CURVE_WITH_KNOTS('',3,(#21637,#21638,#21639,#21640),
 .UNSPECIFIED.,.F.,.F.,(4,4),(-8.84127953393321E-6,-1.00000008615431E-6),
 .UNSPECIFIED.);
#1487=B_SPLINE_CURVE_WITH_KNOTS('',3,(#21641,#21642,#21643,#21644,#21645,
#21646,#21647,#21648,#21649,#21650,#21651,#21652,#21653,#21654,#21655,#21656,
#21657,#21658,#21659,#21660,#21661,#21662,#21663,#21664,#21665,#21666,#21667,
#21668,#21669,#21670,#21671,#21672,#21673,#21674,#21675,#21676,#21677,#21678,
#21679,#21680,#21681,#21682,#21683,#21684,#21685,#21686,#21687,#21688,#21689,
#21690,#21691,#21692,#21693,#21694,#21695,#21696,#21697,#21698,#21699,#21700,
#21701,#21702,#21703,#21704,#21705,#21706,#21707,#21708,#21709,#21710,#21711,
#21712,#21713,#21714,#21715,#21716,#21717,#21718,#21719,#21720,#21721,#21722,
#21723,#21724,#21725,#21726,#21727,#21728,#21729,#21730,#21731,#21732,#21733,
#21734,#21735,#21736,#21737,#21738,#21739,#21740,#21741,#21742,#21743,#21744,
#21745,#21746,#21747,#21748,#21749,#21750,#21751,#21752,#21753,#21754,#21755,
#21756,#21757,#21758,#21759,#21760,#21761,#21762,#21763,#21764,#21765,#21766,
#21767,#21768,#21769,#21770,#21771,#21772,#21773,#21774,#21775,#21776,#21777,
#21778,#21779,#21780,#21781,#21782,#21783,#21784,#21785,#21786,#21787,#21788,
#21789,#21790,#21791,#21792,#21793,#21794,#21795,#21796,#21797,#21798,#21799,
#21800,#21801,#21802,#21803,#21804,#21805,#21806,#21807,#21808,#21809,#21810,
#21811,#21812,#21813,#21814,#21815,#21816,#21817,#21818,#21819,#21820,#21821,
#21822,#21823,#21824,#21825,#21826,#21827,#21828,#21829,#21830,#21831,#21832,
#21833,#21834,#21835,#21836,#21837,#21838,#21839,#21840),.UNSPECIFIED.,
 .F.,.F.,(4,2,2,2,2,2,2,2,2,2,2,2,2,2,2,2,2,2,2,2,2,2,2,2,2,2,2,2,2,2,2,
2,2,2,2,2,2,2,2,2,2,2,2,2,2,2,2,2,2,2,2,2,2,2,2,2,2,2,2,2,2,2,2,2,2,2,2,
2,2,2,2,2,2,2,2,2,2,2,2,2,2,2,2,2,2,2,2,2,2,2,2,2,2,2,2,2,2,2,2,4),(-3.1139997766405,
-3.10786717358469,-3.10313095141403,-3.09929576443767,-3.09566140548508,
-3.09159150592066,-3.08535274331309,-3.06560943062476,-3.04529385652988,
-3.02394341873807,-3.01282322641162,-3.00933168828933,-3.00706504947068,
-3.00503078088594,-3.00158186315971,-2.99170530925925,-2.96049510615426,
-2.93252725611136,-2.92440373088149,-2.91994304339184,-2.91612119592423,
-2.91143107643737,-2.90416139239354,-2.86639798284569,-2.84586666879241,
-2.83499470172268,-2.83152959464521,-2.82926842461164,-2.82722936680897,
-2.82375482122616,-2.81367552186303,-2.78262519304721,-2.75473697020179,
-2.74662346945896,-2.742164791089,-2.73834279398468,-2.73365012307323,-2.7263717616517,
-2.68875306615179,-2.66812854152223,-2.65722786518841,-2.65375964940731,
-2.65149782745637,-2.64917701533559,-2.64543292634974,-2.63283416350648,
-2.60367433854199,-2.57675289645067,-2.56876351241746,-2.56433002413462,
-2.56050627987812,-2.55578162480459,-2.54839345627139,-2.51393502074948,
-2.4911397523198,-2.47960166400224,-2.47606703124804,-2.47379131745189,
-2.471764323461,-2.46835507398318,-2.4587849946654,-2.4273297117135,-2.39923979742529,
-2.39110080403027,-2.38663692546834,-2.38281517452671,-2.37812874833993,
-2.37087190275465,-2.33290063946706,-2.31250068666943,-2.30166922582491,
-2.29820844583645,-2.29594813130233,-2.29362531824098,-2.28987216823794,
-2.27717131240512,-2.27320829484086,-2.22345287285724,-2.21407461879421,
-2.20936838870713,-2.20554594345223,-2.20109867669856,-2.19326244784376,
-2.15385099969815,-2.13433545748308,-2.12378359464746,-2.12035372517665,
-2.11809986380834,-2.11605428501288,-2.11254461890502,-2.10217914219586,
-2.07135506493894,-2.06673609042256,-2.04283669872105,-2.03516634509768,
-2.03079850454282,-2.0269685232856,-2.02215328350044,-2.01218671374677,
-1.99499716658925),.UNSPECIFIED.);
#1488=B_SPLINE_CURVE_WITH_KNOTS('',3,(#21841,#21842,#21843,#21844,#21845,
#21846,#21847,#21848,#21849,#21850,#21851,#21852,#21853,#21854,#21855,#21856,
#21857,#21858,#21859,#21860,#21861,#21862,#21863,#21864,#21865,#21866,#21867,
#21868,#21869,#21870,#21871,#21872,#21873,#21874,#21875,#21876,#21877,#21878,
#21879,#21880,#21881,#21882,#21883,#21884,#21885,#21886,#21887,#21888,#21889,
#21890,#21891,#21892,#21893,#21894,#21895,#21896,#21897,#21898,#21899,#21900,
#21901,#21902,#21903,#21904,#21905,#21906,#21907,#21908,#21909,#21910,#21911,
#21912,#21913,#21914,#21915,#21916,#21917,#21918,#21919,#21920,#21921,#21922,
#21923,#21924,#21925,#21926,#21927,#21928,#21929,#21930,#21931,#21932,#21933,
#21934,#21935,#21936,#21937,#21938,#21939,#21940,#21941,#21942,#21943,#21944,
#21945,#21946,#21947,#21948,#21949,#21950,#21951,#21952,#21953,#21954,#21955,
#21956,#21957,#21958,#21959,#21960,#21961,#21962,#21963,#21964,#21965,#21966,
#21967,#21968,#21969,#21970,#21971,#21972,#21973,#21974,#21975,#21976,#21977,
#21978,#21979,#21980,#21981,#21982,#21983,#21984,#21985,#21986,#21987,#21988,
#21989,#21990,#21991,#21992,#21993,#21994,#21995,#21996,#21997,#21998,#21999,
#22000,#22001,#22002,#22003,#22004,#22005,#22006,#22007,#22008,#22009,#22010,
#22011,#22012,#22013,#22014,#22015,#22016,#22017,#22018,#22019,#22020,#22021,
#22022,#22023,#22024,#22025,#22026,#22027,#22028,#22029,#22030,#22031,#22032),
 .UNSPECIFIED.,.F.,.F.,(4,2,2,2,2,2,2,2,2,2,2,2,2,2,2,2,2,2,2,2,2,2,2,2,
2,2,2,2,2,2,2,2,2,2,2,2,2,2,2,2,2,2,2,2,2,2,2,2,2,2,2,2,2,2,2,2,2,2,2,2,
2,2,2,2,2,2,2,2,2,2,2,2,2,2,2,2,2,2,2,2,2,2,2,2,2,2,2,2,2,2,2,2,2,2,2,4),
(-4.4747574653027,-4.47326539155446,-4.47122679992775,-4.46767864801904,
-4.45680377328828,-4.41412104218659,-4.39490205505733,-4.38888742570857,
-4.38489290809498,-4.3810332425115,-4.37638271074941,-4.36492125697367,
-4.32601974773498,-4.30467944294444,-4.29938452696129,-4.2967560851514,
-4.2948350970118,-4.29221360519118,-4.28695518095048,-4.24670484063484,
-4.22069337965014,-4.21285851551769,-4.20848541952633,-4.20470132826991,
-4.20001110713729,-4.19265121097419,-4.15835777417686,-4.13540421342134,
-4.1275724521397,-4.12191176580497,-4.11921322559772,-4.1170795142747,-4.11441772629565,
-4.10895077624916,-4.08385939488568,-4.05503519514153,-4.04412763514328,
-4.03565801431279,-4.03115696044226,-4.02775233398908,-4.02336644618819,
-4.01568406543595,-3.97510161814073,-3.95622494312453,-3.94590171752278,
-3.94251912163939,-3.94029108632671,-3.93798411401097,-3.93423136146072,
-3.92126178096673,-3.89236486843817,-3.86555605105747,-3.85761566658606,
-3.85322103576581,-3.84943864518334,-3.84477658997144,-3.83751353172781,
-3.8001699924732,-3.77932563528012,-3.7683795602408,-3.76492862796063,-3.76268651608166,
-3.76039736082186,-3.7567269193915,-3.74468139024641,-3.71511917927646,
-3.68796447362976,-3.67997903474244,-3.67557515280169,-3.67179326185878,
-3.66714258339532,-3.65819841061653,-3.61641981939016,-3.59414338260762,
-3.58874711982154,-3.5860987480815,-3.58417668339503,-3.58157344791445,
-3.57640847159548,-3.54345083467954,-3.51260411806326,-3.50319337517041,
-3.49851044195156,-3.49472661487203,-3.49034758989789,-3.48269789941469,
-3.44182256874747,-3.42310799143732,-3.41283808599623,-3.40946136119019,
-3.40723438459369,-3.40492550709695,-3.40116458074908,-3.38810295257325,
-3.35926906550475,-3.35634983843352),.UNSPECIFIED.);
#1489=B_SPLINE_CURVE_WITH_KNOTS('',3,(#22037,#22038,#22039,#22040,#22041,
#22042,#22043,#22044,#22045,#22046,#22047,#22048,#22049,#22050,#22051,#22052,
#22053,#22054,#22055,#22056,#22057,#22058,#22059,#22060,#22061,#22062,#22063,
#22064,#22065,#22066,#22067,#22068,#22069,#22070,#22071,#22072,#22073,#22074,
#22075,#22076,#22077,#22078,#22079,#22080,#22081,#22082,#22083,#22084,#22085,
#22086,#22087,#22088,#22089,#22090,#22091,#22092,#22093,#22094,#22095,#22096,
#22097,#22098,#22099,#22100,#22101,#22102,#22103,#22104,#22105,#22106,#22107,
#22108,#22109,#22110,#22111,#22112,#22113,#22114,#22115,#22116,#22117,#22118,
#22119,#22120,#22121,#22122,#22123,#22124,#22125,#22126,#22127,#22128,#22129,
#22130,#22131,#22132,#22133,#22134,#22135,#22136,#22137,#22138,#22139,#22140,
#22141,#22142,#22143,#22144,#22145,#22146,#22147,#22148,#22149,#22150,#22151,
#22152,#22153,#22154,#22155,#22156,#22157,#22158,#22159,#22160,#22161,#22162,
#22163,#22164,#22165,#22166,#22167,#22168,#22169,#22170,#22171,#22172,#22173,
#22174,#22175,#22176,#22177,#22178,#22179,#22180,#22181,#22182,#22183,#22184,
#22185,#22186,#22187,#22188,#22189,#22190,#22191,#22192,#22193,#22194,#22195,
#22196,#22197,#22198,#22199,#22200,#22201,#22202,#22203,#22204,#22205,#22206,
#22207,#22208,#22209,#22210,#22211,#22212,#22213,#22214,#22215,#22216,#22217,
#22218,#22219,#22220,#22221,#22222),.UNSPECIFIED.,.F.,.F.,(4,2,2,2,2,2,
2,2,2,2,2,2,2,2,2,2,2,2,2,2,2,2,2,2,2,2,2,2,2,2,2,2,2,2,2,2,2,2,2,2,2,2,
2,2,2,2,2,2,2,2,2,2,2,2,2,2,2,2,2,2,2,2,2,2,2,2,2,2,2,2,2,2,2,2,2,2,2,2,
2,2,2,2,2,2,2,2,2,2,2,2,2,2,4),(-1.11918234038498,-1.1062908624538,-1.06420020199838,
-1.05627401622338,-1.05139521280838,-1.04755932581885,-1.04323193802121,
-1.03575732258743,-1.00271471962037,-0.968524114009293,-0.963473507625799,
-0.960844958582337,-0.958901819449467,-0.956218385220644,-0.950725822975816,
-0.927750625134705,-0.883950830818214,-0.87657163698206,-0.87226411565372,
-0.868424820339599,-0.86351270814788,-0.853003765437371,-0.803674626480437,
-0.788656202161589,-0.784710120192069,-0.782345369193335,-0.780113669352325,
-0.776797017681588,-0.767212956474858,-0.750534316864445,-0.708116258644078,
-0.700428817531146,-0.695617705790056,-0.691787629430989,-0.687416035342625,
-0.679729294925883,-0.670155629469278,-0.647579385029872,-0.612791185148299,
-0.607796077431028,-0.605179093552806,-0.603039120201972,-0.600233812846179,
-0.594083704099069,-0.585344457961139,-0.557023668584067,-0.527243108045143,
-0.520442165931277,-0.51625523206506,-0.512384276309439,-0.507226873978072,
-0.495249455226615,-0.477644726311858,-0.443805892544685,-0.432447097693965,
-0.428822092930933,-0.426754044593035,-0.424520151581741,-0.421192464504828,
-0.411519187864713,-0.39459337576055,-0.350426382462267,-0.343098662258047,
-0.338801493034557,-0.334959624219661,-0.330027807099145,-0.31940840349828,
-0.304598944901089,-0.282825937345396,-0.25790938238555,-0.252417953672966,
-0.249734617132589,-0.247577320518606,-0.244837547162199,-0.239047116623659,
-0.230994916129851,-0.206918960243676,-0.174327126996468,-0.166872391128234,
-0.162128208701056,-0.158302974491009,-0.153883642006941,-0.145964835264397,
-0.136010036494511,-0.11182885421081,-0.0797644168535668,-0.0745062912994022,
-0.0718682101913314,-0.0699253668840754,-0.0672516767516004,-0.0618106216543333,
-0.039332013226959,-8.84127953393321E-6),.UNSPECIFIED.);
#1490=B_SPLINE_CURVE_WITH_KNOTS('',3,(#22223,#22224,#22225,#22226,#22227,
#22228,#22229,#22230,#22231,#22232,#22233,#22234,#22235,#22236,#22237,#22238,
#22239,#22240,#22241,#22242,#22243,#22244,#22245,#22246,#22247,#22248,#22249,
#22250,#22251,#22252,#22253,#22254,#22255,#22256,#22257,#22258,#22259,#22260,
#22261,#22262,#22263,#22264,#22265,#22266,#22267,#22268,#22269,#22270,#22271,
#22272,#22273,#22274,#22275,#22276,#22277,#22278,#22279,#22280,#22281,#22282,
#22283,#22284,#22285,#22286,#22287,#22288,#22289,#22290,#22291,#22292,#22293,
#22294,#22295,#22296,#22297,#22298,#22299,#22300,#22301,#22302,#22303,#22304,
#22305,#22306,#22307,#22308,#22309,#22310,#22311,#22312,#22313,#22314,#22315,
#22316,#22317,#22318,#22319,#22320,#22321,#22322,#22323,#22324,#22325,#22326,
#22327,#22328,#22329,#22330,#22331,#22332,#22333,#22334,#22335,#22336,#22337,
#22338,#22339,#22340,#22341,#22342,#22343,#22344,#22345,#22346,#22347,#22348,
#22349,#22350,#22351,#22352,#22353,#22354,#22355,#22356,#22357,#22358,#22359,
#22360,#22361,#22362,#22363,#22364,#22365,#22366,#22367,#22368,#22369,#22370,
#22371,#22372,#22373,#22374,#22375,#22376,#22377,#22378,#22379,#22380,#22381,
#22382,#22383,#22384,#22385,#22386,#22387,#22388,#22389,#22390,#22391,#22392,
#22393,#22394,#22395,#22396,#22397,#22398,#22399,#22400,#22401,#22402,#22403,
#22404,#22405,#22406,#22407,#22408,#22409,#22410,#22411,#22412,#22413,#22414),
 .UNSPECIFIED.,.F.,.F.,(4,2,2,2,2,2,2,2,2,2,2,2,2,2,2,2,2,2,2,2,2,2,2,2,
2,2,2,2,2,2,2,2,2,2,2,2,2,2,2,2,2,2,2,2,2,2,2,2,2,2,2,2,2,2,2,2,2,2,2,2,
2,2,2,2,2,2,2,2,2,2,2,2,2,2,2,2,2,2,2,2,2,2,2,2,2,2,2,2,2,2,2,2,2,2,2,4),
(-3.35634983843352,-3.33249191080876,-3.32455529168109,-3.32016118668897,
-3.31637840165538,-3.31171477689914,-3.30444709018579,-3.2671791475581,
-3.24628183255185,-3.2353193185757,-3.23186644442745,-3.22962379602355,
-3.22733487510822,-3.2236660359991,-3.21163975151283,-3.18206062530389,
-3.15489621736199,-3.14690919416847,-3.14250478707676,-3.13872263380292,
-3.13407187330001,-3.12512831994961,-3.08334466617103,-3.0610658601259,
-3.05566912152535,-3.05302054362203,-3.05109833720453,-3.04849492273822,
-3.04332965330926,-3.00258951258646,-2.9768437089507,-2.96904407031554,
-2.96467787150807,-2.96089270125881,-2.95619201711199,-2.94879706414001,
-2.91718389978793,-2.89224067494513,-2.88405638900473,-2.87820788855236,
-2.8754743670322,-2.87333958130688,-2.87070933097621,-2.86540692544813,
-2.83384428254287,-2.8224081209352,-2.79672242669935,-2.79023351091857,
-2.78614060281697,-2.7822914187972,-2.77706359857726,-2.76442006374167,
-2.74528137378472,-2.70564058946459,-2.70026041146983,-2.69761497718234,
-2.69548054824832,-2.69276357168621,-2.68700532126765,-2.67899245898068,
-2.65503443361358,-2.62214256050429,-2.61475891585796,-2.61006131419861,
-2.60627610830684,-2.60190708367343,-2.59409467479844,-2.56825612461192,
-2.52763087623772,-2.52243623028852,-2.5198268483335,-2.51790470266971,
-2.51526191133981,-2.50989606232597,-2.4879102617746,-2.447037421138,-2.43720688756629,
-2.43244579988985,-2.42865572756464,-2.4243312998688,-2.41673605326765,
-2.3836629341208,-2.34976520886268,-2.34471029969662,-2.34209653468647,
-2.3401745632025,-2.33753633207052,-2.33219414470639,-2.31042880111988,
-2.27023699617197,-2.25978802510393,-2.25491632441335,-2.25111555742662,
-2.24685972821094,-2.23959477212428,-2.23775823947936),.UNSPECIFIED.);
#1491=B_SPLINE_CURVE_WITH_KNOTS('',3,(#22419,#22420,#22421,#22422,#22423,
#22424,#22425,#22426,#22427,#22428,#22429,#22430,#22431,#22432,#22433,#22434,
#22435,#22436,#22437,#22438,#22439,#22440,#22441,#22442,#22443,#22444,#22445,
#22446,#22447,#22448,#22449,#22450,#22451,#22452,#22453,#22454,#22455,#22456,
#22457,#22458,#22459,#22460,#22461,#22462,#22463,#22464,#22465,#22466,#22467,
#22468,#22469,#22470,#22471,#22472,#22473,#22474,#22475,#22476,#22477,#22478,
#22479,#22480,#22481,#22482,#22483,#22484,#22485,#22486,#22487,#22488,#22489,
#22490,#22491,#22492,#22493,#22494,#22495,#22496,#22497,#22498,#22499,#22500,
#22501,#22502,#22503,#22504,#22505,#22506,#22507,#22508,#22509,#22510,#22511,
#22512,#22513,#22514,#22515,#22516,#22517,#22518,#22519,#22520,#22521,#22522,
#22523,#22524,#22525,#22526,#22527,#22528,#22529,#22530,#22531,#22532,#22533,
#22534,#22535,#22536,#22537,#22538,#22539,#22540,#22541,#22542,#22543,#22544,
#22545,#22546,#22547,#22548,#22549,#22550,#22551,#22552,#22553,#22554,#22555,
#22556,#22557,#22558,#22559,#22560,#22561,#22562,#22563,#22564,#22565,#22566,
#22567,#22568,#22569,#22570,#22571,#22572,#22573,#22574,#22575,#22576,#22577,
#22578,#22579,#22580,#22581,#22582,#22583,#22584,#22585,#22586,#22587,#22588,
#22589,#22590,#22591,#22592,#22593,#22594,#22595,#22596,#22597,#22598,#22599,
#22600,#22601,#22602,#22603,#22604,#22605,#22606,#22607,#22608,#22609,#22610),
 .UNSPECIFIED.,.F.,.F.,(4,2,2,2,2,2,2,2,2,2,2,2,2,2,2,2,2,2,2,2,2,2,2,2,
2,2,2,2,2,2,2,2,2,2,2,2,2,2,2,2,2,2,2,2,2,2,2,2,2,2,2,2,2,2,2,2,2,2,2,2,
2,2,2,2,2,2,2,2,2,2,2,2,2,2,2,2,2,2,2,2,2,2,2,2,2,2,2,2,2,2,2,2,2,2,2,4),
(-2.23814687865753,-2.2135431078615,-2.20804974798867,-2.20536657571047,
-2.20321000138374,-2.20047189255,-2.19468748382366,-2.1866456685039,-2.16262154776817,
-2.12990913544601,-2.12249567916594,-2.11776430486937,-2.11394103106288,
-2.10951466569314,-2.10155691898455,-2.07486862763743,-2.04616187342406,
-2.03291166967119,-2.02911129195532,-2.0267786393877,-2.02452685343346,
-2.0211059684685,-2.01063017848018,-1.99134830012102,-1.95159310831359,
-1.94379698917397,-1.93935884234044,-1.93553647479024,-1.93082042781496,
-1.92138755723278,-1.89177308604314,-1.85744923063672,-1.85241202228884,
-1.84978662012121,-1.84784373937883,-1.84515802270196,-1.83965176070333,
-1.81653727947187,-1.77297414864555,-1.76556388724565,-1.76125047510115,
-1.75741319039678,-1.75251366649491,-1.74207275704226,-1.69288029668137,
-1.67766390183171,-1.67370623712585,-1.67133929058727,-1.669109649141,-1.66580200733089,
-1.65628719905207,-1.63979698948903,-1.59813526220858,-1.58909658117665,
-1.58439817327087,-1.5805763911687,-1.57612348144307,-1.56803660795203,
-1.54035334711031,-1.50971775893567,-1.4990832645134,-1.49554139263011,
-1.49348975882711,-1.49124221506284,-1.48784319704305,-1.47756225508325,
-1.45887454988745,-1.41806791807798,-1.41038578606383,-1.40597196746985,
-1.40214721171164,-1.39739805934924,-1.38778977758836,-1.33790151248559,
-1.32215719264125,-1.31816544950352,-1.31579094371483,-1.31356521581295,
-1.3102792001932,-1.30093901363295,-1.28492342671935,-1.2451205505612,-1.23536506023486,
-1.23052833364272,-1.22695015784882,-1.22301506120958,-1.21746655173353,
-1.20277306521964,-1.17853868090279,-1.14658116786608,-1.14131027314233,
-1.13866985603365,-1.13672734415375,-1.13405671890653,-1.12863065038081,
-1.11918234038498),.UNSPECIFIED.);
#1492=B_SPLINE_CURVE_WITH_KNOTS('',3,(#22611,#22612,#22613,#22614,#22615,
#22616,#22617,#22618,#22619,#22620,#22621,#22622,#22623,#22624,#22625,#22626,
#22627,#22628,#22629,#22630,#22631,#22632,#22633,#22634,#22635,#22636,#22637,
#22638,#22639,#22640,#22641,#22642,#22643,#22644,#22645,#22646,#22647,#22648,
#22649,#22650,#22651,#22652,#22653,#22654,#22655,#22656,#22657,#22658,#22659,
#22660,#22661,#22662,#22663,#22664,#22665,#22666,#22667,#22668,#22669,#22670,
#22671,#22672,#22673,#22674,#22675,#22676,#22677,#22678,#22679,#22680,#22681,
#22682,#22683,#22684,#22685,#22686,#22687,#22688,#22689,#22690,#22691,#22692,
#22693,#22694,#22695,#22696,#22697,#22698,#22699,#22700,#22701,#22702,#22703,
#22704,#22705,#22706,#22707,#22708,#22709,#22710,#22711,#22712,#22713,#22714,
#22715,#22716,#22717,#22718,#22719,#22720,#22721,#22722,#22723,#22724,#22725,
#22726,#22727,#22728,#22729,#22730,#22731,#22732,#22733,#22734,#22735,#22736,
#22737,#22738,#22739,#22740,#22741,#22742,#22743,#22744,#22745,#22746,#22747,
#22748,#22749,#22750,#22751,#22752,#22753,#22754,#22755,#22756,#22757,#22758,
#22759,#22760,#22761,#22762,#22763,#22764,#22765,#22766,#22767,#22768,#22769,
#22770,#22771,#22772,#22773,#22774,#22775,#22776,#22777,#22778,#22779,#22780,
#22781,#22782,#22783,#22784,#22785,#22786,#22787,#22788,#22789,#22790,#22791,
#22792,#22793,#22794,#22795,#22796,#22797,#22798,#22799,#22800),
 .UNSPECIFIED.,.F.,.F.,(4,2,2,2,2,2,2,2,2,2,2,2,2,2,2,2,2,2,2,2,2,2,2,2,
2,2,2,2,2,2,2,2,2,2,2,2,2,2,2,2,2,2,2,2,2,2,2,2,2,2,2,2,2,2,2,2,2,2,2,2,
2,2,2,2,2,2,2,2,2,2,2,2,2,2,2,2,2,2,2,2,2,2,2,2,2,2,2,2,2,2,2,2,2,2,4),
(-2.23775823947936,-2.2306787948275,-2.2105876527433,-2.18011911248231,
-2.16924918976833,-2.16570076042661,-2.16366166535568,-2.16144630879085,
-2.15812929492565,-2.14837256766464,-2.13115878676025,-2.08749980007724,
-2.08021312644081,-2.07591269632872,-2.07249887310717,-2.06788847036118,
-2.0588624911135,-2.04698567050094,-2.01247995750546,-1.9926756173253,-1.98852576555277,
-1.98613240962921,-1.98395183348138,-1.98082381188729,-1.97252310223593,
-1.95910552436682,-1.9165349388954,-1.90514840551939,-1.90049182036467,
-1.89662966389264,-1.89263516732375,-1.88662572169422,-1.86748055483274,
-1.82533821083558,-1.81390114510191,-1.81028946515461,-1.80801262562257,
-1.80575850450113,-1.80225267106759,-1.7907813747335,-1.76814683167503,
-1.73342280059525,-1.72607107304305,-1.72138244339194,-1.71759742518013,
-1.71322080996329,-1.70537284397219,-1.6792730193121,-1.63910470544662,
-1.63382059367302,-1.63119350726861,-1.62905801915656,-1.62631944488431,
-1.62044562902757,-1.61221500631695,-1.58699756023594,-1.55576771034777,
-1.54837114322118,-1.54366931039112,-1.53988316331238,-1.53551577810844,
-1.5277139365101,-1.50195977508585,-1.46116523836969,-1.45600131709839,
-1.45339769021933,-1.45147485976189,-1.44882485331593,-1.44342322560829,
-1.4211066069806,-1.37919425383731,-1.37113871850652,-1.36624892683847,
-1.36244561540714,-1.35819883426958,-1.35097941392647,-1.34213654353765,
-1.32231980853656,-1.29254539552005,-1.28073916766702,-1.27709020096959,
-1.27480512246437,-1.27255785141656,-1.26908529886751,-1.25794164288413,
-1.23644403402488,-1.20008984650402,-1.19278206877593,-1.18810591875068,
-1.18432126212414,-1.17993424150091,-1.17203691232783,-1.14556943797177,
-1.12769927842475,-1.11895968873475),.UNSPECIFIED.);
#1493=B_SPLINE_CURVE_WITH_KNOTS('',3,(#22805,#22806,#22807,#22808,#22809,
#22810,#22811,#22812,#22813,#22814,#22815,#22816,#22817,#22818,#22819,#22820,
#22821,#22822,#22823,#22824,#22825,#22826,#22827,#22828,#22829,#22830,#22831,
#22832,#22833,#22834,#22835,#22836,#22837,#22838,#22839,#22840,#22841,#22842,
#22843,#22844,#22845,#22846,#22847,#22848,#22849,#22850,#22851,#22852,#22853,
#22854,#22855,#22856,#22857,#22858,#22859,#22860,#22861,#22862,#22863,#22864,
#22865,#22866,#22867,#22868,#22869,#22870,#22871,#22872,#22873,#22874,#22875,
#22876,#22877,#22878,#22879,#22880,#22881,#22882,#22883,#22884,#22885,#22886,
#22887,#22888,#22889,#22890,#22891,#22892,#22893,#22894,#22895,#22896,#22897,
#22898,#22899,#22900,#22901,#22902,#22903,#22904,#22905,#22906,#22907,#22908,
#22909,#22910,#22911,#22912,#22913,#22914,#22915,#22916,#22917,#22918,#22919,
#22920,#22921,#22922,#22923,#22924,#22925,#22926,#22927,#22928,#22929,#22930,
#22931,#22932,#22933,#22934,#22935,#22936,#22937,#22938,#22939,#22940,#22941,
#22942,#22943,#22944,#22945,#22946,#22947,#22948,#22949,#22950,#22951,#22952,
#22953,#22954,#22955,#22956,#22957,#22958,#22959,#22960,#22961,#22962,#22963,
#22964,#22965,#22966,#22967,#22968,#22969,#22970,#22971,#22972,#22973,#22974,
#22975,#22976,#22977,#22978,#22979,#22980,#22981,#22982,#22983,#22984,#22985,
#22986,#22987,#22988,#22989,#22990,#22991,#22992,#22993,#22994),
 .UNSPECIFIED.,.F.,.F.,(4,2,2,2,2,2,2,2,2,2,2,2,2,2,2,2,2,2,2,2,2,2,2,2,
2,2,2,2,2,2,2,2,2,2,2,2,2,2,2,2,2,2,2,2,2,2,2,2,2,2,2,2,2,2,2,2,2,2,2,2,
2,2,2,2,2,2,2,2,2,2,2,2,2,2,2,2,2,2,2,2,2,2,2,2,2,2,2,2,2,2,2,2,2,2,4),
(-3.35683790262814,-3.35357765786577,-3.34585385121407,-3.30540077861235,
-3.28649997223239,-3.27614956588511,-3.27274304308916,-3.27049436269867,
-3.26815809506247,-3.26434029196816,-3.25091460056561,-3.22236500958243,
-3.19576253352604,-3.18781654161179,-3.18339289860963,-3.17956985962477,
-3.17483605044204,-3.16741316655585,-3.13591493929963,-3.1109545636412,
-3.10275006563831,-3.09688004221786,-3.09412626871319,-3.09196954141775,
-3.08930129384187,-3.08388457979645,-3.05546727072702,-3.01756402987333,
-3.00989126300549,-3.00552378902994,-3.00169511871894,-2.99688284316519,
-2.98692744605904,-2.94617547786139,-2.92425662202074,-2.9188764450497,
-2.91621523552983,-2.91427372240898,-2.91162602237495,-2.90631523604085,
-2.87469984863652,-2.85032156290244,-2.83557786716483,-2.83002403064476,
-2.82608886051902,-2.82203695599074,-2.81588172154763,-2.79710827897907,
-2.7558213741243,-2.74361411904854,-2.73990586470275,-2.73759322536519,
-2.73532576603829,-2.7318285505923,-2.72064779064818,-2.69908882023927,
-2.66293184755867,-2.6555916381664,-2.65088158260726,-2.64705959878097,
-2.6426168781004,-2.63457859630774,-2.60727072001866,-2.57736886295229,
-2.56577349884824,-2.56212375171917,-2.55982375040387,-2.55754508321889,
-2.55399474610088,-2.54229238651305,-2.51889807746939,-2.48532678589276,
-2.47792585839745,-2.47319812513326,-2.46937508068943,-2.4649459590731,
-2.45697466345485,-2.43018299542566,-2.40127561086429,-2.38830531401297,
-2.38452922840036,-2.38220185035745,-2.37994612356052,-2.37650585629217,
-2.36585589829144,-2.34603131104018,-2.30719074307194,-2.29930748410362,
-2.29485059465778,-2.29102945865006,-2.28633699380245,-2.27702906079664,
-2.26467859484985,-2.2396455148825,-2.23814687865753),.UNSPECIFIED.);
#1494=B_SPLINE_CURVE_WITH_KNOTS('',3,(#22995,#22996,#22997,#22998,#22999,
#23000,#23001,#23002,#23003,#23004,#23005,#23006,#23007,#23008,#23009,#23010,
#23011,#23012,#23013,#23014,#23015,#23016,#23017,#23018,#23019,#23020,#23021,
#23022,#23023,#23024,#23025,#23026,#23027,#23028,#23029,#23030,#23031,#23032,
#23033,#23034,#23035,#23036,#23037,#23038,#23039,#23040,#23041,#23042,#23043,
#23044,#23045,#23046,#23047,#23048,#23049,#23050,#23051,#23052,#23053,#23054,
#23055,#23056,#23057,#23058,#23059,#23060,#23061,#23062,#23063,#23064,#23065,
#23066,#23067,#23068,#23069,#23070,#23071,#23072,#23073,#23074,#23075,#23076,
#23077,#23078,#23079,#23080,#23081,#23082,#23083,#23084,#23085,#23086,#23087,
#23088,#23089,#23090,#23091,#23092,#23093,#23094,#23095,#23096,#23097,#23098,
#23099,#23100,#23101,#23102,#23103,#23104,#23105,#23106,#23107,#23108,#23109,
#23110,#23111,#23112,#23113,#23114,#23115,#23116,#23117,#23118,#23119,#23120,
#23121,#23122,#23123,#23124,#23125,#23126,#23127,#23128,#23129,#23130,#23131,
#23132,#23133,#23134,#23135,#23136,#23137,#23138,#23139,#23140,#23141,#23142,
#23143,#23144,#23145,#23146,#23147,#23148,#23149,#23150,#23151,#23152,#23153,
#23154,#23155,#23156,#23157,#23158,#23159,#23160,#23161,#23162,#23163,#23164,
#23165,#23166,#23167,#23168,#23169,#23170,#23171,#23172,#23173,#23174,#23175,
#23176,#23177,#23178,#23179,#23180,#23181,#23182,#23183,#23184,#23185,#23186,
#23187,#23188,#23189,#23190,#23191,#23192),.UNSPECIFIED.,.F.,.F.,(4,2,2,
2,2,2,2,2,2,2,2,2,2,2,2,2,2,2,2,2,2,2,2,2,2,2,2,2,2,2,2,2,2,2,2,2,2,2,2,
2,2,2,2,2,2,2,2,2,2,2,2,2,2,2,2,2,2,2,2,2,2,2,2,2,2,2,2,2,2,2,2,2,2,2,2,
2,2,2,2,2,2,2,2,2,2,2,2,2,2,2,2,2,2,2,2,2,2,2,4),(-1.11895968873475,-1.10411380111841,
-1.09987897483287,-1.09746713616499,-1.09529327166464,-1.09220743431856,
-1.08420511429452,-1.0714953711734,-1.04717908954595,-1.01976971294961,
-1.01309028604818,-1.00895664090545,-1.00512207966775,-0.999995394948391,
-0.9880161445331,-0.970362031004053,-0.936280333397552,-0.92513958812141,
-0.921560035703689,-0.919514596591889,-0.917303792701365,-0.914011914746847,
-0.904466028681687,-0.887843517248697,-0.845775033507896,-0.837836200575998,
-0.832979129487298,-0.82917924137921,-0.824913466164491,-0.817603579294294,
-0.808616297437559,-0.788259925821318,-0.757115212264873,-0.747107063254117,
-0.743661421783218,-0.741641684244542,-0.7394064691808,-0.735992283748977,
-0.725394661679828,-0.705677430006427,-0.666548097173002,-0.658715262066274,
-0.654295701276274,-0.650513021992327,-0.645877390033169,-0.63672301006463,
-0.598906937911911,-0.572919279484284,-0.567445527887247,-0.564781622198941,
-0.562646897977396,-0.559947963286475,-0.554289180390262,-0.546463185408821,
-0.523546856591881,-0.489203837333374,-0.481842564093089,-0.477150685114914,
-0.473364807398216,-0.468989154277872,-0.461148427261187,-0.435108798969085,
-0.394817519824743,-0.389554406945539,-0.386931120857671,-0.385008961842906,
-0.382379103688018,-0.377082322774433,-0.355741782665113,-0.316839225126266,
-0.305377376396611,-0.300724980334268,-0.2968630274758,-0.292865396152958,
-0.286844604131098,-0.267591960181098,-0.224762765940421,-0.213969068077737,
-0.210428582884749,-0.208390538184037,-0.206172796356866,-0.202846521691293,
-0.193018887126509,-0.175607474683788,-0.132306006357323,-0.124964642422751,
-0.120651266930897,-0.117237626708801,-0.112641038413573,-0.103692208073208,
-0.0822647593686294,-0.0506571534242049,-0.0367799085092122,-0.032937057104142,
-0.0306096245284612,-0.0283934190696086,-0.0261254434108124,-0.0228906791297862,
-9.99999999695689E-7),.UNSPECIFIED.);
#1495=B_SPLINE_CURVE_WITH_KNOTS('',3,(#23197,#23198,#23199,#23200,#23201,
#23202,#23203,#23204,#23205,#23206,#23207,#23208,#23209,#23210,#23211,#23212,
#23213,#23214,#23215,#23216,#23217,#23218,#23219,#23220,#23221,#23222,#23223,
#23224,#23225,#23226,#23227,#23228,#23229,#23230,#23231,#23232,#23233,#23234,
#23235,#23236,#23237,#23238,#23239,#23240,#23241,#23242,#23243,#23244,#23245,
#23246,#23247,#23248,#23249,#23250,#23251,#23252,#23253,#23254,#23255,#23256,
#23257,#23258,#23259,#23260,#23261,#23262,#23263,#23264,#23265,#23266,#23267,
#23268,#23269,#23270,#23271,#23272,#23273,#23274,#23275,#23276,#23277,#23278,
#23279,#23280,#23281,#23282,#23283,#23284,#23285,#23286,#23287,#23288,#23289,
#23290,#23291,#23292,#23293,#23294,#23295,#23296,#23297,#23298,#23299,#23300,
#23301,#23302,#23303,#23304,#23305,#23306,#23307,#23308,#23309,#23310,#23311,
#23312,#23313,#23314,#23315,#23316,#23317,#23318,#23319,#23320,#23321,#23322,
#23323,#23324,#23325,#23326,#23327,#23328,#23329,#23330,#23331,#23332,#23333,
#23334,#23335,#23336,#23337,#23338,#23339,#23340,#23341,#23342,#23343,#23344,
#23345,#23346,#23347,#23348,#23349,#23350,#23351,#23352,#23353,#23354,#23355,
#23356,#23357,#23358,#23359,#23360,#23361,#23362,#23363,#23364,#23365,#23366,
#23367,#23368,#23369,#23370,#23371,#23372,#23373,#23374,#23375,#23376,#23377,
#23378,#23379,#23380,#23381,#23382,#23383,#23384,#23385,#23386,#23387,#23388,
#23389,#23390,#23391,#23392),.UNSPECIFIED.,.F.,.F.,(4,2,2,2,2,2,2,2,2,2,
2,2,2,2,2,2,2,2,2,2,2,2,2,2,2,2,2,2,2,2,2,2,2,2,2,2,2,2,2,2,2,2,2,2,2,2,
2,2,2,2,2,2,2,2,2,2,2,2,2,2,2,2,2,2,2,2,2,2,2,2,2,2,2,2,2,2,2,2,2,2,2,2,
2,2,2,2,2,2,2,2,2,2,2,2,2,2,2,4),(-4.47528237196998,-4.47047723035589,-4.43862345421251,
-4.4312285888014,-4.42691966002181,-4.42308370713672,-4.41818221954144,
-4.41016934329169,-4.36820404056406,-4.34590397795295,-4.34048409174089,
-4.3378157277645,-4.33587452597949,-4.3332353725376,-4.32812921860268,-4.29484950989231,
-4.28497268168759,-4.26785736398973,-4.25610986305653,-4.25099165077918,
-4.24712864214056,-4.24292962605829,-4.23606122298278,-4.20572274378787,
-4.18298967547927,-4.16578720960486,-4.16181891012491,-4.15945043105863,
-4.15724954140713,-4.15397333850673,-4.14538372350735,-4.11315834756111,
-4.09242577625489,-4.08332116277573,-4.07592473331271,-4.07161520210312,
-4.06777889623146,-4.06287721053346,-4.05241771468118,-4.01223373781848,
-3.99050106477531,-3.98514170141821,-3.98248491664646,-3.98054400310775,
-3.97789324705692,-3.97256485030836,-3.94187253896268,-3.92933592293723,
-3.90919293646593,-3.89969165200108,-3.89496369824028,-3.89114171457042,
-3.886715201937,-3.87896920685487,-3.83202710892516,-3.81076579878064,-3.8066108135089,
-3.80420169204174,-3.80201968343461,-3.79885226936393,-3.79278801431145,
-3.75398211121775,-3.73562319673773,-3.72716513418025,-3.72017563747995,
-3.7159506928184,-3.71209442869865,-3.7071159046257,-3.69589560817632,-3.65651494500333,
-3.64060826556114,-3.63425811958733,-3.62941417039701,-3.62685997629127,
-3.62469330883092,-3.62184137798591,-3.61524293862453,-3.58112647403818,
-3.55421202871605,-3.5444187757795,-3.53963622105286,-3.5358449858793,-3.53147003892715,
-3.5239638531155,-3.48172499313599,-3.46380297773179,-3.45378220980638,
-3.45041386536529,-3.44817282362102,-3.4461153458794,-3.44254138099382,
-3.43162595691448,-3.39740648965698,-3.37609716138104,-3.36655839977513,
-3.36182292304886,-3.35799986058677,-3.35683790262814),.UNSPECIFIED.);
#1496=B_SPLINE_CURVE_WITH_KNOTS('',3,(#23393,#23394,#23395,#23396,#23397,
#23398,#23399,#23400,#23401,#23402,#23403,#23404,#23405,#23406,#23407,#23408,
#23409,#23410,#23411,#23412,#23413,#23414,#23415,#23416,#23417,#23418,#23419,
#23420,#23421,#23422,#23423,#23424,#23425,#23426,#23427,#23428,#23429,#23430,
#23431,#23432,#23433,#23434,#23435,#23436,#23437,#23438,#23439,#23440,#23441,
#23442,#23443,#23444,#23445,#23446,#23447,#23448,#23449,#23450,#23451,#23452,
#23453,#23454,#23455,#23456,#23457,#23458,#23459,#23460,#23461,#23462,#23463,
#23464,#23465,#23466,#23467,#23468,#23469,#23470,#23471,#23472,#23473,#23474,
#23475,#23476,#23477,#23478,#23479,#23480,#23481,#23482,#23483,#23484,#23485,
#23486,#23487,#23488,#23489,#23490,#23491,#23492,#23493,#23494,#23495,#23496,
#23497,#23498,#23499,#23500,#23501,#23502,#23503,#23504,#23505,#23506,#23507,
#23508,#23509,#23510,#23511,#23512,#23513,#23514,#23515,#23516,#23517,#23518,
#23519,#23520,#23521,#23522,#23523,#23524,#23525,#23526,#23527,#23528,#23529,
#23530,#23531,#23532,#23533,#23534,#23535,#23536,#23537,#23538,#23539,#23540,
#23541,#23542,#23543,#23544,#23545,#23546,#23547,#23548,#23549,#23550,#23551,
#23552,#23553,#23554,#23555,#23556,#23557,#23558,#23559,#23560,#23561,#23562,
#23563,#23564,#23565,#23566,#23567,#23568,#23569,#23570,#23571,#23572,#23573,
#23574),.UNSPECIFIED.,.F.,.F.,(4,2,2,2,2,2,2,2,2,2,2,2,2,2,2,2,2,2,2,2,
2,2,2,2,2,2,2,2,2,2,2,2,2,2,2,2,2,2,2,2,2,2,2,2,2,2,2,2,2,2,2,2,2,2,2,2,
2,2,2,2,2,2,2,2,2,2,2,2,2,2,2,2,2,2,2,2,2,2,2,2,2,2,2,2,2,2,2,2,2,2,4),
(-5.87804291519136,-5.83428954882498,-5.82829041028316,-5.82294371139109,
-5.81907490801547,-5.81550538548975,-5.80963855698751,-5.79334671522187,
-5.75865981592281,-5.74436672223993,-5.73578386261734,-5.73280426955157,
-5.73057178090971,-5.72827007924657,-5.72454245732517,-5.71186594800043,
-5.68276522388351,-5.65583554927645,-5.64787886969071,-5.64348057715903,
-5.6396979335013,-5.63503926031245,-5.62605695335963,-5.58431836518343,
-5.5620534799279,-5.55665815010132,-5.55400980969516,-5.55208757616313,
-5.54948383284988,-5.5443170746154,-5.50358300320923,-5.47783277690756,
-5.47003244416382,-5.46566604134631,-5.46188079631145,-5.45718015171272,
-5.4476761320721,-5.40641244311933,-5.38429743054231,-5.37891796515281,
-5.37627265464834,-5.37435053032704,-5.3717438696003,-5.36656247948738,
-5.32590154556352,-5.30010996779205,-5.29230396448624,-5.28793634411328,
-5.28415112530444,-5.27945191620595,-5.27206242725214,-5.23952580457398,
-5.21527610276786,-5.20721117918484,-5.20142578494464,-5.19870381434753,
-5.19656930218491,-5.19392852014822,-5.1885722263864,-5.15862408070966,
-5.12462702874218,-5.11549139675546,-5.11086024345266,-5.10707884573524,
-5.10265808316319,-5.09481585154511,-5.05578815584266,-5.0359972321654,
-5.0253775937572,-5.0219615698462,-5.01972644842878,-5.01742789985704,-5.01371512856654,
-5.00120823539113,-4.97197344022922,-4.94498753853897,-4.93702333926827,
-4.93262338654208,-4.92884066508907,-4.92418361562163,-4.91520998264583,
-4.87345860958561,-4.85118928593465,-4.84579334459361,-4.84314481144704,
-4.84122248507763,-4.83861868496744,-4.83345201237418,-4.79271438968909,
-4.76696387829719,-4.7594056615118),.UNSPECIFIED.);
#1497=B_SPLINE_CURVE_WITH_KNOTS('',3,(#23579,#23580,#23581,#23582,#23583,
#23584,#23585,#23586,#23587,#23588,#23589,#23590,#23591,#23592,#23593,#23594,
#23595,#23596,#23597,#23598,#23599,#23600,#23601,#23602,#23603,#23604,#23605,
#23606,#23607,#23608,#23609,#23610,#23611,#23612,#23613,#23614,#23615,#23616,
#23617,#23618,#23619,#23620,#23621,#23622,#23623,#23624,#23625,#23626,#23627,
#23628,#23629,#23630,#23631,#23632,#23633,#23634,#23635,#23636,#23637,#23638,
#23639,#23640,#23641,#23642,#23643,#23644,#23645,#23646,#23647,#23648,#23649,
#23650,#23651,#23652,#23653,#23654,#23655,#23656,#23657,#23658,#23659,#23660,
#23661,#23662,#23663,#23664,#23665,#23666,#23667,#23668,#23669,#23670,#23671,
#23672,#23673,#23674,#23675,#23676,#23677,#23678,#23679,#23680,#23681,#23682,
#23683,#23684,#23685,#23686,#23687,#23688,#23689,#23690,#23691,#23692,#23693,
#23694,#23695,#23696,#23697,#23698,#23699,#23700,#23701,#23702,#23703,#23704,
#23705,#23706,#23707,#23708,#23709,#23710,#23711,#23712,#23713,#23714,#23715,
#23716,#23717,#23718,#23719,#23720,#23721,#23722,#23723,#23724,#23725,#23726,
#23727,#23728,#23729,#23730,#23731,#23732,#23733,#23734,#23735,#23736,#23737,
#23738,#23739,#23740,#23741,#23742,#23743,#23744,#23745,#23746,#23747,#23748,
#23749,#23750,#23751,#23752,#23753,#23754,#23755,#23756,#23757,#23758,#23759,
#23760,#23761,#23762,#23763,#23764,#23765,#23766,#23767,#23768,#23769,#23770,
#23771,#23772),.UNSPECIFIED.,.F.,.F.,(4,2,2,2,2,2,2,2,2,2,2,2,2,2,2,2,2,
2,2,2,2,2,2,2,2,2,2,2,2,2,2,2,2,2,2,2,2,2,2,2,2,2,2,2,2,2,2,2,2,2,2,2,2,
2,2,2,2,2,2,2,2,2,2,2,2,2,2,2,2,2,2,2,2,2,2,2,2,2,2,2,2,2,2,2,2,2,2,2,2,
2,2,2,2,2,2,2,4),(-5.59347479354677,-5.58807672447325,-5.58435005752554,
-5.58212670041714,-5.58008295740095,-5.57771331531301,-5.57373863595134,
-5.55820622565288,-5.53272755108873,-5.50561552972491,-5.49760493978463,
-5.49316936137948,-5.48934906854456,-5.48463540563768,-5.4772780294438,
-5.44177303429365,-5.41975774612149,-5.40844599917441,-5.40493631486158,
-5.40266706912718,-5.40035913339524,-5.39666901672206,-5.38464048325009,
-5.35509884269625,-5.32798821861477,-5.31997777097135,-5.31554219737878,
-5.31172186855447,-5.30700810989418,-5.29965048052116,-5.26415229808797,
-5.24213182981134,-5.23081854038086,-5.22730867691153,-5.22503938040182,
-5.22301030220606,-5.21958369115782,-5.20986766975057,-5.17855977522271,
-5.1505528619324,-5.14242792885165,-5.13796910805751,-5.13415027008705,
-5.12946562572585,-5.12220797647264,-5.08436854797338,-5.06391983137564,
-5.05307682654478,-5.04961659819174,-5.04735761613324,-5.04503721383123,
-5.04128965961214,-5.02862871070675,-4.99954302071318,-4.97538888975385,
-4.96575233058842,-4.96099979415817,-4.95717698050517,-4.95277054711678,
-4.9451147238471,-4.90171911749374,-4.87898361711773,-4.87351808336627,
-4.87084099033883,-4.86889946118434,-4.86626868776896,-4.86120223923617,
-4.82730798027529,-4.79342366251387,-4.78631404860024,-4.78206472161939,
-4.77821628183218,-4.77328954451502,-4.76237520202226,-4.7226860216023,
-4.70111672781088,-4.69577545993641,-4.69312237978978,-4.69096580656558,
-4.68819678079606,-4.6822404680028,-4.64253983138402,-4.62406030050576,
-4.61168744557028,-4.60647096795489,-4.60259365871226,-4.59843558921065,
-4.59176214847682,-4.56585748649067,-4.53423326734789,-4.52503823731938,
-4.51865789027738,-4.51581332248875,-4.51365233107255,-4.51105966357998,
-4.5061733925627,-4.47528237196998),.UNSPECIFIED.);
#1498=B_SPLINE_CURVE_WITH_KNOTS('',3,(#23773,#23774,#23775,#23776,#23777,
#23778,#23779,#23780,#23781,#23782,#23783,#23784,#23785,#23786,#23787,#23788,
#23789,#23790,#23791,#23792,#23793,#23794,#23795,#23796,#23797,#23798,#23799,
#23800,#23801,#23802,#23803,#23804,#23805,#23806,#23807,#23808,#23809,#23810,
#23811,#23812,#23813,#23814,#23815,#23816,#23817,#23818,#23819,#23820,#23821,
#23822,#23823,#23824,#23825,#23826,#23827,#23828,#23829,#23830,#23831,#23832,
#23833,#23834,#23835,#23836,#23837,#23838,#23839,#23840,#23841,#23842,#23843,
#23844,#23845,#23846,#23847,#23848,#23849,#23850,#23851,#23852,#23853,#23854,
#23855,#23856,#23857,#23858,#23859,#23860,#23861,#23862,#23863,#23864,#23865,
#23866,#23867,#23868,#23869,#23870,#23871,#23872,#23873,#23874,#23875,#23876,
#23877,#23878,#23879,#23880,#23881,#23882,#23883,#23884,#23885,#23886,#23887,
#23888,#23889,#23890,#23891,#23892,#23893,#23894,#23895,#23896,#23897,#23898,
#23899,#23900,#23901,#23902,#23903,#23904,#23905,#23906,#23907,#23908,#23909,
#23910,#23911,#23912,#23913,#23914,#23915,#23916,#23917,#23918,#23919,#23920,
#23921,#23922,#23923,#23924,#23925,#23926,#23927,#23928,#23929,#23930,#23931,
#23932,#23933,#23934,#23935,#23936,#23937,#23938,#23939,#23940,#23941,#23942,
#23943,#23944,#23945,#23946,#23947,#23948,#23949,#23950,#23951,#23952,#23953,
#23954,#23955,#23956,#23957,#23958,#23959,#23960,#23961,#23962,#23963,#23964),
 .UNSPECIFIED.,.F.,.F.,(4,2,2,2,2,2,2,2,2,2,2,2,2,2,2,2,2,2,2,2,2,2,2,2,
2,2,2,2,2,2,2,2,2,2,2,2,2,2,2,2,2,2,2,2,2,2,2,2,2,2,2,2,2,2,2,2,2,2,2,2,
2,2,2,2,2,2,2,2,2,2,2,2,2,2,2,2,2,2,2,2,2,2,2,2,2,2,2,2,2,2,2,2,2,2,2,4),
(-4.7594056615118,-4.75916330577551,-4.75479672118297,-4.75101129435165,
-4.74631039257129,-4.73891530401789,-4.70719446169042,-4.68232964832486,
-4.67415843637189,-4.66831673066041,-4.66558434060177,-4.66344945119886,
-4.66081785017293,-4.65550907898097,-4.61551129383112,-4.58934791442217,
-4.58149202619319,-4.57711419077999,-4.57332984680469,-4.56864428510768,
-4.55952917681014,-4.5179460685827,-4.49572971738074,-4.49033941106809,
-4.48769197418721,-4.48576971140616,-4.48316492434027,-4.47799320373326,
-4.4372816241478,-4.41151702480388,-4.40371457412652,-4.3993476243877,-4.39556225843814,
-4.3908619219216,-4.38346872551801,-4.35136889676871,-4.32679103395646,
-4.31866905695481,-4.31285339061202,-4.31012580084012,-4.30799108118059,
-4.30535524801632,-4.30002464936691,-4.26014378983,-4.23391405862721,-4.22604935253471,
-4.22166972820171,-4.21788555135072,-4.21320240403191,-4.20586823551696,
-4.17037682459832,-4.14826396719347,-4.13694184716023,-4.13345136577009,
-4.1312007176295,-4.12892069615413,-4.12529343302871,-4.11370198611476,
-4.07175374732255,-4.05264402967884,-4.04663861118359,-4.04264522344916,
-4.03878297021516,-4.03412481326402,-4.02272719228344,-3.98378700268498,
-3.96243294563211,-3.95713583172976,-3.95450653780041,-3.95258512661787,
-3.94996333437502,-3.94470465884547,-3.90444441227508,-3.87843060752874,
-3.87059482566671,-3.86622117402689,-3.86243658461173,-3.85774573179725,
-3.85038484489403,-3.81606518686078,-3.79311963822545,-3.78528875550116,
-3.77962833525715,-3.77692965610979,-3.77479566282334,-3.77213332398795,
-3.76666483697129,-3.74041889739658,-3.7152018259883,-3.69704299919251,
-3.69113025998066,-3.68715534970216,-3.68327872888863,-3.67856335764708,
-3.66680938922734,-3.6407755406643),.UNSPECIFIED.);
#1499=B_SPLINE_CURVE_WITH_KNOTS('',3,(#23969,#23970,#23971,#23972,#23973,
#23974,#23975,#23976,#23977,#23978,#23979,#23980,#23981,#23982,#23983,#23984,
#23985,#23986,#23987,#23988,#23989,#23990,#23991,#23992,#23993,#23994,#23995,
#23996,#23997,#23998,#23999,#24000,#24001,#24002,#24003,#24004,#24005,#24006,
#24007,#24008,#24009,#24010,#24011,#24012,#24013,#24014,#24015,#24016,#24017,
#24018,#24019,#24020,#24021,#24022,#24023,#24024,#24025,#24026,#24027,#24028,
#24029,#24030,#24031,#24032,#24033,#24034,#24035,#24036,#24037,#24038,#24039,
#24040,#24041,#24042,#24043,#24044,#24045,#24046,#24047,#24048,#24049,#24050,
#24051,#24052,#24053,#24054,#24055,#24056,#24057,#24058,#24059,#24060,#24061,
#24062,#24063,#24064,#24065,#24066,#24067,#24068,#24069,#24070,#24071,#24072,
#24073,#24074,#24075,#24076,#24077,#24078,#24079,#24080,#24081,#24082,#24083,
#24084,#24085,#24086,#24087,#24088,#24089,#24090,#24091,#24092,#24093,#24094,
#24095,#24096,#24097,#24098,#24099,#24100,#24101,#24102,#24103,#24104,#24105,
#24106,#24107,#24108,#24109,#24110,#24111,#24112,#24113,#24114,#24115,#24116,
#24117,#24118,#24119,#24120,#24121,#24122,#24123,#24124,#24125,#24126,#24127,
#24128,#24129,#24130,#24131,#24132,#24133,#24134,#24135,#24136,#24137,#24138,
#24139,#24140,#24141,#24142,#24143,#24144,#24145,#24146,#24147,#24148),
 .UNSPECIFIED.,.F.,.F.,(4,2,2,2,2,2,2,2,2,2,2,2,2,2,2,2,2,2,2,2,2,2,2,2,
2,2,2,2,2,2,2,2,2,2,2,2,2,2,2,2,2,2,2,2,2,2,2,2,2,2,2,2,2,2,2,2,2,2,2,2,
2,2,2,2,2,2,2,2,2,2,2,2,2,2,2,2,2,2,2,2,2,2,2,2,2,2,2,2,2,4),(-1.11906078687382,
-1.10181719756328,-1.07310984421461,-1.05985843780124,-1.05605785257306,
-1.05372509720322,-1.05147323486519,-1.04805226761362,-1.03757651050938,
-1.01829523112983,-0.978536216269192,-0.970740034232509,-0.966301768190049,
-0.962479250577419,-0.957762957824193,-0.9483293794914,-0.918682663292412,
-0.884394640018681,-0.879353917502312,-0.876727716162809,-0.874784802186414,
-0.872099751645558,-0.866597293280621,-0.843520949547377,-0.799894699950944,
-0.792492933571567,-0.788181185011461,-0.784343434533903,-0.779440633115032,
-0.768981750228283,-0.719754271889976,-0.704590573714031,-0.700636004371981,
-0.698269671638376,-0.696039532100416,-0.692729599962305,-0.683196969960408,
-0.666658254259388,-0.624802868658829,-0.616701865773417,-0.611773993293723,
-0.607933222527686,-0.603635240958969,-0.596301011987247,-0.561970404022273,
-0.528936071610351,-0.523812934010734,-0.521169299097288,-0.519227056119098,
-0.516560149568661,-0.511152813789114,-0.488987640439833,-0.447454108425651,
-0.438305665834496,-0.433584979099549,-0.429761832363847,-0.42532611326299,
-0.417324444703676,-0.390305014645148,-0.360961861247237,-0.348590528670158,
-0.344866857353913,-0.342550622966136,-0.340285453920716,-0.336800480941869,
-0.325739876617737,-0.304587218315611,-0.267819782241878,-0.260501620447879,
-0.255797549618092,-0.251975284101376,-0.247526455782177,-0.239460438723052,
-0.211942495746812,-0.18163303708696,-0.170569331621413,-0.166977681682724,
-0.164916385687827,-0.162677538410238,-0.159322775234664,-0.149421481335123,
-0.131848696431952,-0.0889657923829509,-0.0815460130446182,-0.0771890969075821,
-0.0737410664450437,-0.0690969878737329,-0.0600445857718003,-0.0481504936189692,
-9.99999999695689E-7),.UNSPECIFIED.);
#1500=B_SPLINE_CURVE_WITH_KNOTS('',3,(#24149,#24150,#24151,#24152,#24153,
#24154,#24155,#24156,#24157,#24158,#24159,#24160,#24161,#24162,#24163,#24164,
#24165,#24166,#24167,#24168,#24169,#24170,#24171,#24172,#24173,#24174,#24175,
#24176,#24177,#24178,#24179,#24180,#24181,#24182,#24183,#24184,#24185,#24186,
#24187,#24188,#24189,#24190,#24191,#24192,#24193,#24194,#24195,#24196,#24197,
#24198,#24199,#24200,#24201,#24202,#24203,#24204,#24205,#24206,#24207,#24208,
#24209,#24210,#24211,#24212,#24213,#24214,#24215,#24216,#24217,#24218,#24219,
#24220,#24221,#24222,#24223,#24224,#24225,#24226,#24227,#24228,#24229,#24230,
#24231,#24232,#24233,#24234,#24235,#24236,#24237,#24238,#24239,#24240,#24241,
#24242,#24243,#24244,#24245,#24246,#24247,#24248,#24249,#24250,#24251,#24252,
#24253,#24254,#24255,#24256,#24257,#24258,#24259,#24260,#24261,#24262,#24263,
#24264,#24265,#24266,#24267,#24268,#24269,#24270,#24271,#24272,#24273,#24274,
#24275,#24276,#24277,#24278,#24279,#24280,#24281,#24282,#24283,#24284,#24285,
#24286,#24287,#24288,#24289,#24290,#24291,#24292,#24293,#24294,#24295,#24296,
#24297,#24298,#24299,#24300,#24301,#24302,#24303,#24304,#24305,#24306,#24307,
#24308,#24309,#24310,#24311,#24312,#24313,#24314,#24315,#24316,#24317,#24318,
#24319,#24320,#24321,#24322,#24323,#24324,#24325,#24326,#24327,#24328,#24329,
#24330,#24331,#24332,#24333,#24334,#24335,#24336,#24337,#24338,#24339,#24340,
#24341,#24342),.UNSPECIFIED.,.F.,.F.,(4,2,2,2,2,2,2,2,2,2,2,2,2,2,2,2,2,
2,2,2,2,2,2,2,2,2,2,2,2,2,2,2,2,2,2,2,2,2,2,2,2,2,2,2,2,2,2,2,2,2,2,2,2,
2,2,2,2,2,2,2,2,2,2,2,2,2,2,2,2,2,2,2,2,2,2,2,2,2,2,2,2,2,2,2,2,2,2,2,2,
2,2,2,2,2,2,2,4),(-3.6407755406643,-3.62823903672922,-3.60700928379253,
-3.60172573997997,-3.59909903792633,-3.59717765690908,-3.59455315925463,
-3.58928091310584,-3.54908947617732,-3.52303528128578,-3.51519394260481,
-3.51081905962426,-3.50703443352383,-3.50234486406071,-3.4929005906048,
-3.45156694260271,-3.42942943882715,-3.42404749039955,-3.42140165389513,
-3.41947945289459,-3.41687313615243,-3.41169372364897,-3.37102076726245,
-3.35234718742111,-3.34381987960854,-3.33679933930009,-3.3325947975643,
-3.32878302319415,-3.32389942684178,-3.31307527719816,-3.27326274865875,
-3.25161763985724,-3.24628853709875,-3.24365289391343,-3.24173109409809,
-3.23911501905084,-3.23388618372287,-3.19346535835553,-3.16753769189963,
-3.15971312550493,-3.15534155112109,-3.15155645389728,-3.14686198986802,
-3.13948935050053,-3.1057489287751,-3.08238121793475,-3.07070644041987,
-3.06718040000695,-3.06492211178239,-3.06292211275666,-3.05958180117751,
-3.05037771374336,-3.01440216970852,-2.99645323504766,-2.98433891606545,
-2.97919187937283,-2.97535497670775,-2.97123095057607,-2.96459447602382,
-2.93872912865183,-2.93340985404414,-2.90132098855327,-2.89249856975364,
-2.88921095074664,-2.88702328263193,-2.88469439189205,-2.88084226481917,
-2.8651484840993,-2.81840307593977,-2.80672333963632,-2.80204735075143,
-2.79818063723277,-2.79419315902494,-2.78821736028043,-2.76942161240239,
-2.7294038732124,-2.71583954369029,-2.7120227562128,-2.70970158445304,-2.70748275509494,
-2.70414770152325,-2.69423857097695,-2.67658905883789,-2.63377780420986,
-2.62637505797203,-2.62204939522561,-2.61829579818965,-2.6135555260694,
-2.60383795248285,-2.57737223856036,-2.54430079730469,-2.53664274838501,
-2.53352848575528,-2.53135035542992,-2.52895156704685,-2.52477599256707,
-2.52207415166318),.UNSPECIFIED.);
#1501=B_SPLINE_CURVE_WITH_KNOTS('',3,(#24347,#24348,#24349,#24350,#24351,
#24352,#24353,#24354,#24355,#24356,#24357,#24358,#24359,#24360,#24361,#24362,
#24363,#24364,#24365,#24366,#24367,#24368,#24369,#24370,#24371,#24372,#24373,
#24374,#24375,#24376,#24377,#24378,#24379,#24380,#24381,#24382,#24383,#24384,
#24385,#24386,#24387,#24388,#24389,#24390,#24391,#24392,#24393,#24394,#24395,
#24396,#24397,#24398,#24399,#24400,#24401,#24402,#24403,#24404,#24405,#24406,
#24407,#24408,#24409,#24410,#24411,#24412,#24413,#24414,#24415,#24416,#24417,
#24418,#24419,#24420,#24421,#24422,#24423,#24424,#24425,#24426,#24427,#24428,
#24429,#24430,#24431,#24432,#24433,#24434,#24435,#24436,#24437,#24438,#24439,
#24440,#24441,#24442,#24443,#24444,#24445,#24446,#24447,#24448,#24449,#24450,
#24451,#24452,#24453,#24454,#24455,#24456,#24457,#24458,#24459,#24460,#24461,
#24462,#24463,#24464,#24465,#24466,#24467,#24468,#24469,#24470,#24471,#24472,
#24473,#24474,#24475,#24476,#24477,#24478,#24479,#24480,#24481,#24482,#24483,
#24484,#24485,#24486,#24487,#24488,#24489,#24490,#24491,#24492,#24493,#24494,
#24495,#24496,#24497,#24498,#24499,#24500,#24501,#24502,#24503,#24504,#24505,
#24506,#24507,#24508,#24509,#24510,#24511,#24512,#24513,#24514,#24515,#24516,
#24517,#24518,#24519,#24520,#24521,#24522,#24523,#24524,#24525,#24526,#24527,
#24528,#24529,#24530,#24531,#24532,#24533,#24534,#24535,#24536,#24537,#24538,
#24539,#24540,#24541,#24542,#24543,#24544,#24545,#24546),.UNSPECIFIED.,
 .F.,.F.,(4,2,2,2,2,2,2,2,2,2,2,2,2,2,2,2,2,2,2,2,2,2,2,2,2,2,2,2,2,2,2,
2,2,2,2,2,2,2,2,2,2,2,2,2,2,2,2,2,2,2,2,2,2,2,2,2,2,2,2,2,2,2,2,2,2,2,2,
2,2,2,2,2,2,2,2,2,2,2,2,2,2,2,2,2,2,2,2,2,2,2,2,2,2,2,2,2,2,2,2,4),(-2.23776655190534,
-2.22778578623218,-2.21664579712278,-2.21168012354498,-2.20782513931058,
-2.20359282740332,-2.19657021046483,-2.1880595607134,-2.16951684413861,
-2.12944471222924,-2.12375041193938,-2.1210291076989,-2.11887273919109,
-2.11617347515858,-2.11059588467045,-2.10293885699918,-2.08100606667912,
-2.04538751067939,-2.03803063366754,-2.03331568678251,-2.02949337242211,
-2.02505434611152,-2.01703446455939,-1.98986969167966,-1.96024391688906,
-1.94827036633159,-1.94458385716107,-1.94227588363341,-1.94000430311049,
-1.9364876183063,-1.92511940665894,-1.90291729705943,-1.86768145878101,
-1.86031451822166,-1.85559661619329,-1.85177409368628,-1.84733727421533,
-1.83932839729022,-1.81224894927909,-1.78278746473526,-1.77058686454044,
-1.76687912336045,-1.76456653678717,-1.76229886971181,-1.75880094410284,
-1.74761424893408,-1.7260357946128,-1.68990457598868,-1.68256316367106,
-1.67785265847939,-1.67403051214529,-1.66958782970314,-1.66155027080362,
-1.63424936346443,-1.60436186620528,-1.59274498114508,-1.58909299526128,
-1.58679245191756,-1.58451411436486,-1.58096560717457,-1.56928261965791,
-1.54595979798705,-1.51228753497942,-1.5048880403939,-1.50016062331006,
-1.4963374611204,-1.49190778691123,-1.48393431199371,-1.45712731518792,
-1.42819116049543,-1.41525896850161,-1.41148607262065,-1.40915932826513,
-1.40690296117056,-1.40345985565169,-1.39278493394391,-1.37288208127055,
-1.33416753650424,-1.32627293824911,-1.32181350710689,-1.31799236189653,
-1.3133026310134,-1.30400972084381,-1.29168642256704,-1.26662142927137,
-1.24049651601774,-1.23500310922807,-1.23231986406611,-1.23016320455181,
-1.22742495387376,-1.22164013264208,-1.21359765320601,-1.18957061295041,
-1.15685959066571,-1.14944581247,-1.14471424361301,-1.14089081936404,-1.13646428735957,
-1.12850626248216,-1.11906078687382),.UNSPECIFIED.);
#1502=B_SPLINE_CURVE_WITH_KNOTS('',3,(#24547,#24548,#24549,#24550,#24551,
#24552,#24553,#24554,#24555,#24556,#24557,#24558,#24559,#24560,#24561,#24562,
#24563,#24564,#24565,#24566,#24567,#24568,#24569,#24570,#24571,#24572,#24573,
#24574,#24575,#24576,#24577,#24578,#24579,#24580,#24581,#24582,#24583,#24584,
#24585,#24586,#24587,#24588,#24589,#24590,#24591,#24592,#24593,#24594,#24595,
#24596,#24597,#24598,#24599,#24600,#24601,#24602,#24603,#24604,#24605,#24606,
#24607,#24608,#24609,#24610,#24611,#24612,#24613,#24614,#24615,#24616,#24617,
#24618,#24619,#24620,#24621,#24622,#24623,#24624,#24625,#24626,#24627,#24628,
#24629,#24630,#24631,#24632,#24633,#24634,#24635,#24636,#24637,#24638,#24639,
#24640,#24641,#24642,#24643,#24644,#24645,#24646,#24647,#24648,#24649,#24650,
#24651,#24652,#24653,#24654,#24655,#24656,#24657,#24658,#24659,#24660,#24661,
#24662,#24663,#24664,#24665,#24666,#24667,#24668,#24669,#24670,#24671,#24672,
#24673,#24674,#24675,#24676,#24677,#24678,#24679,#24680,#24681,#24682,#24683,
#24684,#24685,#24686,#24687,#24688,#24689,#24690,#24691,#24692,#24693,#24694,
#24695,#24696,#24697,#24698,#24699,#24700,#24701,#24702,#24703,#24704,#24705,
#24706,#24707,#24708,#24709,#24710,#24711,#24712,#24713,#24714,#24715,#24716,
#24717,#24718,#24719,#24720,#24721,#24722,#24723,#24724,#24725,#24726,#24727,
#24728),.UNSPECIFIED.,.F.,.F.,(4,2,2,2,2,2,2,2,2,2,2,2,2,2,2,2,2,2,2,2,
2,2,2,2,2,2,2,2,2,2,2,2,2,2,2,2,2,2,2,2,2,2,2,2,2,2,2,2,2,2,2,2,2,2,2,2,
2,2,2,2,2,2,2,2,2,2,2,2,2,2,2,2,2,2,2,2,2,2,2,2,2,2,2,2,2,2,2,2,2,2,4),
(-2.52207415166318,-2.50206841203732,-2.46446175317106,-2.45172959676644,
-2.44635922366383,-2.44252463193816,-2.43848787273917,-2.43227004783753,
-2.41069345718137,-2.3885425896863,-2.36325986778271,-2.35778913772044,
-2.35512636640086,-2.35299237400426,-2.35029414092764,-2.34463609308825,
-2.33681053428452,-2.31388984004935,-2.27957568644593,-2.27221660022988,
-2.26752623532568,-2.26374165393042,-2.2593675818048,-2.25152992085083,
-2.22550200042049,-2.18521970032241,-2.17995933267413,-2.17733713184624,
-2.17541562739576,-2.17278648651977,-2.16749056544787,-2.14614859757975,
-2.10723329517739,-2.0958338754606,-2.09117530941448,-2.08731277540526,
-2.08331918032209,-2.07731364598697,-2.05820821299268,-2.0163187509785,
-2.00463549312324,-2.0009988307737,-1.99871665196085,-1.99646751707909,
-1.99298496162698,-1.9817412005249,-1.95989985959076,-1.92405458162906,
-1.9167314612759,-1.91205125203168,-1.90826690519131,-1.90388424971708,
-1.89600615329143,-1.86967868930399,-1.82991359984729,-1.82455454730925,
-1.82191297490756,-1.81977812844573,-1.81705613250725,-1.81127200173337,
-1.80321084471109,-1.77898103129641,-1.74644665056317,-1.73905782061798,
-1.7343583600182,-1.73057254762485,-1.72620380801291,-1.71839467068711,
-1.6925848514777,-1.65189557172077,-1.64671162497265,-1.6441041290424,-1.64218160476008,
-1.63953604339504,-1.63415702417674,-1.61205188560703,-1.57080945029454,
-1.56129886500964,-1.55659637503463,-1.55281023028015,-1.54844343437122,
-1.54064428709557,-1.51490962759984,-1.47408083978773,-1.46892385649621,
-1.46632162108433,-1.4643987424934,-1.46174729928031,-1.45633810353154,
-1.43394943723756,-1.40333270505807),.UNSPECIFIED.);
#1503=B_SPLINE_CURVE_WITH_KNOTS('',3,(#24733,#24734,#24735,#24736,#24737,
#24738,#24739,#24740,#24741,#24742,#24743,#24744,#24745,#24746,#24747,#24748,
#24749,#24750,#24751,#24752,#24753,#24754,#24755,#24756,#24757,#24758,#24759,
#24760,#24761,#24762,#24763,#24764,#24765,#24766,#24767,#24768,#24769,#24770,
#24771,#24772,#24773,#24774,#24775,#24776,#24777,#24778,#24779,#24780,#24781,
#24782,#24783,#24784,#24785,#24786,#24787,#24788,#24789,#24790,#24791,#24792,
#24793,#24794,#24795,#24796,#24797,#24798,#24799,#24800,#24801,#24802,#24803,
#24804,#24805,#24806,#24807,#24808,#24809,#24810,#24811,#24812,#24813,#24814,
#24815,#24816,#24817,#24818,#24819,#24820,#24821,#24822,#24823,#24824,#24825,
#24826,#24827,#24828,#24829,#24830,#24831,#24832,#24833,#24834,#24835,#24836,
#24837,#24838,#24839,#24840,#24841,#24842,#24843,#24844,#24845,#24846,#24847,
#24848,#24849,#24850,#24851,#24852,#24853,#24854,#24855,#24856,#24857,#24858,
#24859,#24860,#24861,#24862,#24863,#24864,#24865,#24866,#24867,#24868,#24869,
#24870,#24871,#24872,#24873,#24874,#24875,#24876,#24877,#24878,#24879,#24880,
#24881,#24882,#24883,#24884,#24885,#24886,#24887,#24888,#24889,#24890,#24891,
#24892,#24893,#24894,#24895,#24896,#24897,#24898,#24899,#24900,#24901,#24902,
#24903,#24904,#24905,#24906,#24907,#24908,#24909,#24910,#24911,#24912,#24913,
#24914,#24915,#24916),.UNSPECIFIED.,.F.,.F.,(4,2,2,2,2,2,2,2,2,2,2,2,2,
2,2,2,2,2,2,2,2,2,2,2,2,2,2,2,2,2,2,2,2,2,2,2,2,2,2,2,2,2,2,2,2,2,2,2,2,
2,2,2,2,2,2,2,2,2,2,2,2,2,2,2,2,2,2,2,2,2,2,2,2,2,2,2,2,2,2,2,2,2,2,2,2,
2,2,2,2,2,2,4),(-3.35656936323946,-3.35555127465481,-3.32125403551656,-3.28820983530958,
-3.28081612012118,-3.27650623210897,-3.27266845797338,-3.26776330812124,
-3.25974149257815,-3.21776520366904,-3.19545770585155,-3.1900357074741,
-3.18736623355975,-3.18542419206659,-3.18278384966788,-3.17767527426617,
-3.14438515086975,-3.11390942837666,-3.10446815054549,-3.09975052997067,
-3.09592804175039,-3.09149104512586,-3.0837004338175,-3.04385229748872,
-3.024599256753,-3.0141329395229,-3.01071300288342,-3.00846140166676,-3.00612842555101,
-3.0023267254962,-2.98906039023524,-2.96038806981269,-2.93372108698596,
-2.92576600805621,-2.92134013310743,-2.91751671201493,-2.91278442265208,
-2.90536798090327,-2.87272536694968,-2.84861875839361,-2.84056139604117,
-2.83476916045929,-2.83202954047909,-2.8298728733851,-2.82719094453908,
-2.82170433253122,-2.79694262892508,-2.75551924072584,-2.74791231423617,
-2.74351509727161,-2.73968923629371,-2.73491848454737,-2.72519181982528,
-2.69923303146447,-2.66701656038511,-2.65836964724076,-2.65508520061442,
-2.65288217854081,-2.65051509482237,-2.64655600455908,-2.62952967427972,
-2.606724886456,-2.5761167337456,-2.56932854922896,-2.56514525967573,-2.56127491228829,
-2.55611414860776,-2.54410822702096,-2.52643877688118,-2.49218433746845,
-2.48127201763248,-2.47769798563009,-2.47564030585883,-2.47339885108536,
-2.47002962529166,-2.4600033876834,-2.44206790014104,-2.39988659582721,
-2.3923755358656,-2.38799913327179,-2.38420743676287,-2.37942535194345,
-2.36963725670147,-2.34279343300518,-2.30884761957336,-2.30220229640161,
-2.29951233806927,-2.29732480005187,-2.29492679668286,-2.29082494000496,
-2.27093300085587,-2.23776655190534),.UNSPECIFIED.);
#1504=B_SPLINE_CURVE_WITH_KNOTS('',3,(#24917,#24918,#24919,#24920,#24921,
#24922,#24923,#24924,#24925,#24926,#24927,#24928,#24929,#24930,#24931,#24932,
#24933,#24934,#24935,#24936,#24937,#24938,#24939,#24940,#24941,#24942,#24943,
#24944,#24945,#24946,#24947,#24948,#24949,#24950,#24951,#24952,#24953,#24954,
#24955,#24956,#24957,#24958,#24959,#24960,#24961,#24962,#24963,#24964,#24965,
#24966,#24967,#24968,#24969,#24970,#24971,#24972,#24973,#24974,#24975,#24976,
#24977,#24978,#24979,#24980,#24981,#24982,#24983,#24984,#24985,#24986,#24987,
#24988,#24989,#24990,#24991,#24992,#24993,#24994,#24995,#24996,#24997,#24998,
#24999,#25000,#25001,#25002,#25003,#25004,#25005,#25006,#25007,#25008,#25009,
#25010,#25011,#25012,#25013,#25014,#25015,#25016,#25017,#25018,#25019,#25020,
#25021,#25022,#25023,#25024,#25025,#25026,#25027,#25028,#25029,#25030,#25031,
#25032,#25033,#25034,#25035,#25036,#25037,#25038,#25039,#25040,#25041,#25042,
#25043,#25044,#25045,#25046,#25047,#25048,#25049,#25050,#25051,#25052,#25053,
#25054,#25055,#25056,#25057,#25058,#25059,#25060,#25061,#25062,#25063,#25064,
#25065,#25066,#25067,#25068,#25069,#25070,#25071,#25072,#25073,#25074,#25075,
#25076,#25077,#25078,#25079,#25080,#25081,#25082,#25083,#25084,#25085,#25086,
#25087,#25088,#25089,#25090,#25091,#25092,#25093,#25094,#25095,#25096,#25097,
#25098,#25099,#25100,#25101,#25102,#25103,#25104,#25105,#25106,#25107,#25108,
#25109,#25110,#25111,#25112),.UNSPECIFIED.,.F.,.F.,(4,2,2,2,2,2,2,2,2,2,
2,2,2,2,2,2,2,2,2,2,2,2,2,2,2,2,2,2,2,2,2,2,2,2,2,2,2,2,2,2,2,2,2,2,2,2,
2,2,2,2,2,2,2,2,2,2,2,2,2,2,2,2,2,2,2,2,2,2,2,2,2,2,2,2,2,2,2,2,2,2,2,2,
2,2,2,2,2,2,2,2,2,2,2,2,2,2,2,4),(-1.40333270505807,-1.39180496678422,-1.38392532244935,
-1.37908510902709,-1.37528713446274,-1.37101173818054,-1.36365501010383,
-1.35459247470321,-1.33394975120503,-1.30206072713359,-1.2929855579044,
-1.28966239596659,-1.2876652123249,-1.28540198829625,-1.28185430165187,
-1.26996114954773,-1.24578375012125,-1.21317340681559,-1.20578470752908,
-1.20108506819908,-1.19729894975835,-1.19292967789213,-1.18511908715568,
-1.1593012102664,-1.11861909634247,-1.11343263107251,-1.1108245046547,-1.10890183810593,
-1.10625649130622,-1.10087928630155,-1.07879355873006,-1.03761450685677,
-1.02804453512103,-1.02333075030235,-1.0195435390437,-1.01518434310488,
-1.00742336881242,-0.981972349650676,-0.942889925412528,-0.936347579360866,
-0.933521154772953,-0.931375470272141,-0.928851084358466,-0.924080862653826,
-0.917843806981941,-0.902339974435919,-0.864568329010454,-0.852002180895898,
-0.846648034177631,-0.842815239216356,-0.838771758290313,-0.83252560572496,
-0.810600085930862,-0.777169269684361,-0.761045995716779,-0.757048841356857,
-0.754688083131964,-0.752491564931561,-0.749275647617909,-0.740329476473356,
-0.725306406312121,-0.689299238443309,-0.674905702836174,-0.669275744450861,
-0.665746532577764,-0.661838468612679,-0.656277745601053,-0.641234339962453,
-0.615943597650611,-0.585574514865633,-0.58023773391861,-0.577600153769365,
-0.575464728532464,-0.572737155145714,-0.566924620767498,-0.558810478590108,
-0.534280246766163,-0.502134147682818,-0.494740521236823,-0.490039151188441,
-0.486252506650955,-0.481883586689752,-0.474076312195854,-0.448286801894074,
-0.407543046084399,-0.402367119870654,-0.39976088305286,-0.397837877267002,
-0.3951898587088,-0.389799803486504,-0.367596725965957,-0.326050794354874,
-0.316907653683928,-0.312215329333407,-0.308429144525465,-0.304053194457995,
-0.296212098783039,-0.284404947939953),.UNSPECIFIED.);
#1505=B_SPLINE_CURVE_WITH_KNOTS('',3,(#25117,#25118,#25119,#25120,#25121,
#25122,#25123,#25124,#25125,#25126,#25127,#25128,#25129,#25130,#25131,#25132,
#25133,#25134,#25135,#25136,#25137,#25138,#25139,#25140,#25141,#25142,#25143,
#25144,#25145,#25146,#25147,#25148,#25149,#25150,#25151,#25152,#25153,#25154,
#25155,#25156,#25157,#25158,#25159,#25160,#25161,#25162,#25163,#25164,#25165,
#25166,#25167,#25168,#25169,#25170,#25171,#25172,#25173,#25174,#25175,#25176,
#25177,#25178,#25179,#25180,#25181,#25182,#25183,#25184,#25185,#25186,#25187,
#25188,#25189,#25190,#25191,#25192,#25193,#25194,#25195,#25196,#25197,#25198,
#25199,#25200,#25201,#25202,#25203,#25204,#25205,#25206,#25207,#25208,#25209,
#25210,#25211,#25212,#25213,#25214,#25215,#25216,#25217,#25218,#25219,#25220,
#25221,#25222,#25223,#25224,#25225,#25226,#25227,#25228,#25229,#25230,#25231,
#25232,#25233,#25234,#25235,#25236,#25237,#25238,#25239,#25240,#25241,#25242,
#25243,#25244,#25245,#25246,#25247,#25248,#25249,#25250,#25251,#25252,#25253,
#25254,#25255,#25256,#25257,#25258,#25259,#25260,#25261,#25262,#25263,#25264,
#25265,#25266,#25267,#25268,#25269,#25270,#25271,#25272,#25273,#25274,#25275,
#25276,#25277,#25278,#25279,#25280,#25281,#25282,#25283,#25284,#25285,#25286,
#25287,#25288,#25289,#25290,#25291,#25292,#25293,#25294,#25295,#25296,#25297,
#25298,#25299,#25300,#25301,#25302,#25303,#25304,#25305,#25306,#25307,#25308),
 .UNSPECIFIED.,.F.,.F.,(4,2,2,2,2,2,2,2,2,2,2,2,2,2,2,2,2,2,2,2,2,2,2,2,
2,2,2,2,2,2,2,2,2,2,2,2,2,2,2,2,2,2,2,2,2,2,2,2,2,2,2,2,2,2,2,2,2,2,2,2,
2,2,2,2,2,2,2,2,2,2,2,2,2,2,2,2,2,2,2,2,2,2,2,2,2,2,2,2,2,2,2,2,2,2,2,4),
(-4.47541535506956,-4.46168686137262,-4.44533441280584,-4.43587076265126,
-4.43256971887689,-4.43034159877718,-4.42797315272518,-4.42400722012639,
-4.40863814634345,-4.35957448054162,-4.34919030325548,-4.3443013728649,
-4.3404657866815,-4.33614740160655,-4.32871089717986,-4.28530688791141,
-4.26206648242813,-4.25654768593994,-4.25385985597878,-4.25191710041922,
-4.24929425656539,-4.24426872711686,-4.20985718613612,-4.18035113457065,
-4.17092206770026,-4.16620681143604,-4.16238453193918,-4.15794585879716,
-4.15014716487225,-4.11038765894985,-4.09108798791207,-4.08060676665653,
-4.07718518013403,-4.07493325664548,-4.0726008339112,-4.06880135011771,
-4.05555828463033,-4.02687172384334,-4.00019836087532,-3.9922427238327,
-3.98781690381526,-3.98399372975824,-3.97926200361188,-3.97184697266457,
-3.9391156034799,-3.91507687253339,-3.90703168782298,-3.90124602681201,
-3.89850774136233,-3.89635124901468,-3.89366845105915,-3.88817669969464,
-3.86208059548485,-3.83705228453644,-3.82471930302464,-3.81542028956979,
-3.81072961079175,-3.80690864128574,-3.80245048847723,-3.79456111958678,
-3.75575123577177,-3.73588263896161,-3.72521886941121,-3.72177702776948,
-3.71952101947594,-3.71747823061421,-3.71398209636885,-3.70372433307347,
-3.67282322957182,-3.64501249227021,-3.63690987293162,-3.63245405580393,
-3.62863283941965,-3.62393900825083,-3.61492168625518,-3.5732146648061,
-3.5567089770894,-3.54718924110773,-3.54388110561216,-3.54165151987289,
-3.53928502288142,-3.53532886607847,-3.520127671446,-3.47095822590636,-3.46051875941119,
-3.45561973619867,-3.45178272220362,-3.44746948386088,-3.44005925236906,
-3.39646855509076,-3.37334785738748,-3.36784106763373,-3.36515533871445,
-3.36321256861206,-3.36058746060944,-3.35656936323946),.UNSPECIFIED.);
#1506=B_SPLINE_CURVE_WITH_KNOTS('',3,(#25310,#25311,#25312,#25313,#25314,
#25315,#25316,#25317,#25318,#25319,#25320,#25321,#25322,#25323,#25324,#25325,
#25326,#25327,#25328,#25329,#25330,#25331,#25332,#25333,#25334,#25335,#25336,
#25337,#25338,#25339,#25340,#25341,#25342,#25343,#25344,#25345,#25346,#25347,
#25348,#25349,#25350,#25351,#25352,#25353,#25354,#25355,#25356,#25357,#25358,
#25359,#25360,#25361,#25362,#25363),.UNSPECIFIED.,.F.,.F.,(4,2,2,2,2,2,
2,2,2,2,2,2,2,2,2,2,2,2,2,2,2,2,2,2,2,2,4),(-0.284404947939953,-0.270172367198298,
-0.229874565476045,-0.224611707048033,-0.22198834889193,-0.220066038374403,
-0.217435847933057,-0.212137987545278,-0.190789670724902,-0.151863692286156,
-0.140453460071792,-0.135791956829375,-0.131927557084387,-0.12793261428107,
-0.127722266749346,-0.127515952580895,-0.127311165663978,-0.120991416525271,
-0.0984562989763039,-0.068449773798942,-0.0501364229208393,-0.0460294130521238,
-0.0436447259434375,-0.0414592423917343,-0.0383062002011589,-0.0346567302149804,
-1.00000007596801E-6),.UNSPECIFIED.);
#1507=B_SPLINE_CURVE_WITH_KNOTS('',3,(#25364,#25365,#25366,#25367,#25368,
#25369,#25370,#25371,#25372,#25373,#25374,#25375,#25376,#25377,#25378,#25379,
#25380,#25381,#25382,#25383,#25384,#25385,#25386,#25387,#25388,#25389,#25390,
#25391,#25392,#25393,#25394,#25395,#25396,#25397,#25398,#25399,#25400,#25401,
#25402,#25403,#25404,#25405,#25406,#25407,#25408,#25409,#25410,#25411,#25412,
#25413,#25414,#25415,#25416,#25417,#25418,#25419,#25420,#25421,#25422,#25423,
#25424,#25425,#25426,#25427,#25428,#25429,#25430,#25431,#25432,#25433,#25434,
#25435,#25436,#25437,#25438,#25439,#25440,#25441,#25442,#25443,#25444,#25445,
#25446,#25447,#25448,#25449,#25450,#25451,#25452,#25453,#25454,#25455,#25456,
#25457,#25458,#25459,#25460,#25461,#25462,#25463,#25464,#25465,#25466,#25467,
#25468,#25469,#25470,#25471,#25472,#25473,#25474,#25475,#25476,#25477,#25478,
#25479,#25480,#25481,#25482,#25483,#25484,#25485,#25486,#25487,#25488,#25489,
#25490,#25491,#25492,#25493,#25494,#25495,#25496,#25497,#25498,#25499,#25500,
#25501,#25502,#25503),.UNSPECIFIED.,.F.,.F.,(4,2,2,2,2,2,2,2,2,2,2,2,2,
2,2,2,2,2,2,2,2,2,2,2,2,2,2,2,2,2,2,2,2,2,2,2,2,2,2,2,2,2,2,2,2,2,2,2,2,
2,2,2,2,2,2,2,2,2,2,2,2,2,2,2,2,2,2,2,2,4),(-2.78528382917142,-2.75364564113469,
-2.7479236220945,-2.74389220912167,-2.73990123562933,-2.73603756310898,
-2.730500203602,-2.71674562910167,-2.68539492617632,-2.66658365863005,-2.65633953007895,
-2.65293211477355,-2.6506989187282,-2.64839843243281,-2.64467601346079,
-2.63205701367805,-2.60292403279826,-2.57596910413347,-2.5680093946514,
-2.56361064585203,-2.55982826922107,-2.55517076527411,-2.54619342395583,
-2.50445187477274,-2.4821865743147,-2.47679137541237,-2.47414315349886,
-2.47222103006302,-2.4696174720036,-2.46445118591793,-2.42371839248954,
-2.39797007301252,-2.39017024092275,-2.38580409826865,-2.38201906787512,
-2.37731867580989,-2.3699244246843,-2.33819048119904,-2.3133407563055,-2.30517252526879,
-2.29933255121657,-2.29660064970405,-2.29446597990667,-2.29183444493081,
-2.28652522000183,-2.25581462821527,-2.23078124691386,-2.21582959706935,
-2.2102821720436,-2.20637775030518,-2.2028480572464,-2.19810938354337,-2.18620812017513,
-2.14779364809033,-2.12661720906565,-2.12133974114435,-2.11871432878208,
-2.11679312333415,-2.11416773570442,-2.10889029317753,-2.07714911463725,
-2.04501048191141,-2.03575757397118,-2.03110424504657,-2.02732192769614,
-2.02291949771949,-2.01516199718309,-1.97526101342384,-1.95598866852601,
-1.95100679492342),.UNSPECIFIED.);
#1508=B_SPLINE_CURVE_WITH_KNOTS('',3,(#25508,#25509,#25510,#25511,#25512,
#25513,#25514,#25515,#25516,#25517,#25518,#25519,#25520,#25521,#25522,#25523,
#25524,#25525,#25526,#25527,#25528,#25529,#25530,#25531,#25532,#25533,#25534,
#25535,#25536,#25537,#25538,#25539,#25540,#25541,#25542,#25543,#25544,#25545,
#25546,#25547,#25548,#25549,#25550,#25551,#25552,#25553,#25554,#25555,#25556,
#25557,#25558,#25559,#25560,#25561,#25562,#25563,#25564,#25565,#25566,#25567,
#25568,#25569,#25570,#25571,#25572,#25573,#25574,#25575,#25576,#25577,#25578,
#25579,#25580,#25581,#25582,#25583,#25584,#25585,#25586,#25587,#25588,#25589,
#25590,#25591,#25592,#25593,#25594,#25595,#25596,#25597,#25598,#25599,#25600,
#25601,#25602,#25603,#25604,#25605,#25606,#25607,#25608,#25609,#25610,#25611,
#25612,#25613,#25614,#25615,#25616,#25617,#25618,#25619,#25620,#25621,#25622,
#25623,#25624,#25625,#25626,#25627,#25628,#25629,#25630,#25631,#25632,#25633,
#25634,#25635,#25636,#25637,#25638,#25639,#25640,#25641,#25642,#25643,#25644,
#25645,#25646,#25647,#25648,#25649,#25650,#25651,#25652,#25653,#25654,#25655,
#25656,#25657,#25658,#25659,#25660,#25661,#25662,#25663,#25664,#25665,#25666,
#25667,#25668,#25669,#25670,#25671,#25672,#25673,#25674,#25675,#25676,#25677,
#25678,#25679,#25680,#25681,#25682,#25683,#25684,#25685,#25686,#25687,#25688,
#25689,#25690,#25691,#25692,#25693,#25694,#25695,#25696,#25697),
 .UNSPECIFIED.,.F.,.F.,(4,2,2,2,2,2,2,2,2,2,2,2,2,2,2,2,2,2,2,2,2,2,2,2,
2,2,2,2,2,2,2,2,2,2,2,2,2,2,2,2,2,2,2,2,2,2,2,2,2,2,2,2,2,2,2,2,2,2,2,2,
2,2,2,2,2,2,2,2,2,2,2,2,2,2,2,2,2,2,2,2,2,2,2,2,2,2,2,2,2,2,2,2,2,2,4),
(-5.59412685259837,-5.59079749322766,-5.58706650607828,-5.58325343288845,
-5.57816116599502,-5.56703780700355,-5.55515778378523,-5.52852241784322,
-5.50624596204639,-5.50081915829663,-5.49814446445037,-5.49620376172452,
-5.49357538154047,-5.48832539662164,-5.44800403895801,-5.42206233474434,
-5.41422411608657,-5.40983907550084,-5.40603862202533,-5.40131995821258,
-5.39389820250337,-5.36222593143895,-5.33716186302814,-5.32894506223185,
-5.32307482262384,-5.32033251940357,-5.31818374485663,-5.31552536636805,
-5.31016011256005,-5.28001907319866,-5.26691352921521,-5.24678523095788,
-5.2372719210887,-5.23253588769219,-5.22870608381427,-5.22426871236286,
-5.2164973218407,-5.17337899731163,-5.15076202123844,-5.1453029460488,-5.1426215065187,
-5.14067493464708,-5.13803367491682,-5.13292813033915,-5.09216515141719,
-5.07358446581026,-5.06116526850781,-5.05593904557034,-5.05205763222523,
-5.04789803646789,-5.04122847992687,-5.01557096191177,-4.98367582600429,
-4.97444231866549,-4.96804160561886,-4.96519274997924,-4.96303123623948,
-4.96044185452032,-4.95556893832469,-4.91973687145443,-4.89137995357993,
-4.88196568341991,-4.87725561231467,-4.87343668509704,-4.8690010824479,
-4.86120608588939,-4.82140137807094,-4.79333583803964,-4.78903001248988,
-4.7865895642039,-4.78439568255832,-4.78128742872615,-4.77381971697473,
-4.73603092395748,-4.71084072008013,-4.70308375071154,-4.69869793736525,
-4.69486983733739,-4.69008022840632,-4.682466772192,-4.63995977772311,-4.61749354531017,
-4.61205413732695,-4.60938064304101,-4.60743790905339,-4.60479978098107,
-4.59953957600136,-4.55924132226508,-4.53329226432026,-4.52543286037423,
-4.52102660453907,-4.51720154419937,-4.51244309002777,-4.50278325045138,
-4.47541535506956),.UNSPECIFIED.);
#1509=B_SPLINE_CURVE_WITH_KNOTS('',3,(#25698,#25699,#25700,#25701,#25702,
#25703,#25704,#25705,#25706,#25707,#25708,#25709,#25710,#25711,#25712,#25713,
#25714,#25715,#25716,#25717,#25718,#25719,#25720,#25721,#25722,#25723,#25724,
#25725,#25726,#25727,#25728,#25729,#25730,#25731,#25732,#25733,#25734,#25735,
#25736,#25737,#25738,#25739,#25740,#25741,#25742,#25743,#25744,#25745,#25746,
#25747,#25748,#25749,#25750,#25751,#25752,#25753,#25754,#25755,#25756,#25757,
#25758,#25759,#25760,#25761,#25762,#25763,#25764,#25765,#25766,#25767,#25768,
#25769,#25770,#25771,#25772,#25773,#25774,#25775,#25776,#25777,#25778,#25779,
#25780,#25781,#25782,#25783,#25784,#25785,#25786,#25787,#25788,#25789,#25790,
#25791,#25792,#25793,#25794,#25795,#25796,#25797,#25798,#25799,#25800,#25801,
#25802,#25803,#25804,#25805,#25806,#25807,#25808,#25809,#25810,#25811,#25812,
#25813,#25814,#25815,#25816,#25817,#25818,#25819,#25820,#25821,#25822,#25823,
#25824,#25825,#25826,#25827,#25828,#25829,#25830,#25831,#25832,#25833,#25834,
#25835,#25836,#25837,#25838,#25839,#25840,#25841,#25842,#25843,#25844,#25845,
#25846,#25847,#25848,#25849,#25850,#25851,#25852,#25853,#25854,#25855,#25856,
#25857,#25858,#25859,#25860,#25861,#25862,#25863,#25864,#25865,#25866,#25867,
#25868,#25869,#25870,#25871,#25872,#25873,#25874,#25875,#25876,#25877,#25878,
#25879,#25880,#25881,#25882,#25883,#25884,#25885,#25886,#25887,#25888,#25889,
#25890,#25891),.UNSPECIFIED.,.F.,.F.,(4,2,2,2,2,2,2,2,2,2,2,2,2,2,2,2,2,
2,2,2,2,2,2,2,2,2,2,2,2,2,2,2,2,2,2,2,2,2,2,2,2,2,2,2,2,2,2,2,2,2,2,2,2,
2,2,2,2,2,2,2,2,2,2,2,2,2,2,2,2,2,2,2,2,2,2,2,2,2,2,2,2,2,2,2,2,2,2,2,2,
2,2,2,2,2,2,2,4),(-1.95100679492342,-1.94553554215874,-1.94213804667716,
-1.93990677847412,-1.93760342501637,-1.93386827799253,-1.9211061129625,
-1.89205500980332,-1.86516454365593,-1.85721285694531,-1.85281552171066,
-1.8490327262702,-1.84437262323765,-1.83711752238394,-1.79960420208942,
-1.77886519124092,-1.76795054004047,-1.76450259684623,-1.76226086455139,
-1.75997037499978,-1.75629508311787,-1.74420221440886,-1.71467095383175,
-1.68753171550091,-1.6795476308099,-1.67514356190614,-1.67136099812686,
-1.66670883466499,-1.65948140456391,-1.61342297959296,-1.59858137919268,
-1.5897072467776,-1.58650130339884,-1.58430710390816,-1.58194401922727,
-1.57793351072505,-1.5615167452042,-1.52840572645558,-1.5065328814406,-1.50029265420715,
-1.49625140444382,-1.49241959655834,-1.48706498107939,-1.47448297266626,
-1.42888359813295,-1.41329652895715,-1.40945124094734,-1.40712386440035,
-1.40493521178522,-1.40164279743205,-1.39278676886684,-1.3776007473694,
-1.34099707081957,-1.32723999252894,-1.3217014440573,-1.31783681791631,
-1.31384474109794,-1.30784874779921,-1.28885002096639,-1.24763459236768,
-1.23527343263245,-1.2315727575126,-1.22927636683713,-1.22703745359635,
-1.22360767810163,-1.21287322602267,-1.19272101647304,-1.15434161743092,
-1.14714426159606,-1.14249979135334,-1.13871603367635,-1.13430210616619,
-1.1262755604058,-1.09882103744547,-1.06870098323283,-1.05736223775691,
-1.05376093847029,-1.05148614440694,-1.04923168946894,-1.04571900156196,
-1.03416374504659,-1.01122841272118,-0.976885677006135,-0.969525378929181,
-0.964835896402267,-0.961053219295875,-0.95668279022599,-0.948856123583707,
-0.922899839858273,-0.882464950763336,-0.877231291446488,-0.874614949859364,
-0.872693355038265,-0.870058734919367,-0.864737193551888,-0.84317229986637,
-0.832307780531444),.UNSPECIFIED.);
#1510=B_SPLINE_CURVE_WITH_KNOTS('',3,(#25894,#25895,#25896,#25897,#25898,
#25899,#25900,#25901,#25902,#25903,#25904,#25905,#25906,#25907,#25908,#25909,
#25910,#25911,#25912,#25913,#25914,#25915,#25916,#25917,#25918,#25919,#25920,
#25921,#25922,#25923,#25924,#25925,#25926,#25927,#25928,#25929,#25930,#25931,
#25932,#25933,#25934,#25935,#25936,#25937,#25938,#25939,#25940,#25941,#25942,
#25943,#25944,#25945,#25946,#25947,#25948,#25949,#25950,#25951,#25952,#25953,
#25954,#25955,#25956,#25957,#25958,#25959,#25960,#25961,#25962,#25963,#25964,
#25965,#25966,#25967,#25968,#25969,#25970,#25971,#25972,#25973,#25974,#25975,
#25976,#25977,#25978,#25979,#25980,#25981,#25982,#25983,#25984,#25985,#25986,
#25987,#25988,#25989,#25990,#25991,#25992,#25993,#25994,#25995,#25996,#25997,
#25998,#25999,#26000,#26001,#26002,#26003,#26004,#26005,#26006,#26007,#26008,
#26009,#26010,#26011,#26012,#26013,#26014,#26015,#26016,#26017,#26018,#26019,
#26020,#26021,#26022,#26023,#26024,#26025,#26026,#26027,#26028,#26029),
 .UNSPECIFIED.,.F.,.F.,(4,2,2,2,2,2,2,2,2,2,2,2,2,2,2,2,2,2,2,2,2,2,2,2,
2,2,2,2,2,2,2,2,2,2,2,2,2,2,2,2,2,2,2,2,2,2,2,2,2,2,2,2,2,2,2,2,2,2,2,2,
2,2,2,2,2,2,2,4),(-0.832307780531444,-0.803606962550582,-0.792532170867328,
-0.787604593523706,-0.783784651759978,-0.779597549081722,-0.772669392876491,
-0.736864982324837,-0.704657593195993,-0.699432919648634,-0.696815583722776,
-0.694888675712656,-0.692239894271248,-0.686870239755252,-0.664899577261703,
-0.623967025926869,-0.614309574681314,-0.609574598285637,-0.605779361378094,
-0.601420409921478,-0.59368514277229,-0.568473347132404,-0.53078202781163,
-0.523131006997847,-0.520017135668432,-0.517841181344571,-0.515459817405454,
-0.511318375460975,-0.489224089921067,-0.453364914229101,-0.438613909661366,
-0.432952124786665,-0.429433073020253,-0.425561083238544,-0.420101227587134,
-0.405685289338776,-0.38210524528157,-0.348919550486812,-0.343768735724256,
-0.341174915133529,-0.339059128014593,-0.336300366826654,-0.33034234242747,
-0.32196005697253,-0.295896905419883,-0.265630080528906,-0.25816004805516,
-0.25342267499459,-0.249614257711656,-0.245227481539917,-0.237405466381312,
-0.211605047688619,-0.171183813116732,-0.165958067294306,-0.163327191202409,
-0.161148882230516,-0.158303798009289,-0.152045195291431,-0.14310176820436,
-0.113102447558771,-0.0868888313403523,-0.0802339149149218,-0.0760706983808306,
-0.0721754751008024,-0.0669130928135195,-0.0543151460759675,-0.0354023257144985,
-8.33025589524125E-5),.UNSPECIFIED.);
#1511=B_SPLINE_CURVE_WITH_KNOTS('',3,(#26033,#26034,#26035,#26036,#26037,
#26038,#26039,#26040,#26041,#26042,#26043,#26044,#26045,#26046,#26047,#26048,
#26049,#26050,#26051,#26052,#26053,#26054,#26055,#26056,#26057,#26058,#26059,
#26060,#26061,#26062,#26063,#26064,#26065,#26066,#26067,#26068,#26069,#26070,
#26071,#26072,#26073,#26074,#26075,#26076,#26077,#26078,#26079,#26080,#26081,
#26082,#26083,#26084,#26085,#26086,#26087,#26088,#26089,#26090,#26091,#26092),
 .UNSPECIFIED.,.F.,.F.,(4,2,2,2,2,2,2,2,2,2,2,2,2,2,2,2,2,2,2,2,2,2,2,2,
2,2,2,2,2,4),(9.3173987231798E-5,0.0292812570885843,0.0454952117975465,
0.0567410279340209,0.0615976477439388,0.0652310829591134,0.0691415936521615,
0.0754297094370028,0.0985636797155863,0.13271691496439,0.1421093260704,
0.146574060412193,0.150075744261853,0.152251280319118,0.154401966945945,
0.15748619652452,0.164866877593732,0.176361847037279,0.221040972857858,
0.238352711784817,0.244744219454318,0.248677461565565,0.252990814812306,
0.259080628847928,0.274571258417318,0.297181812282976,0.321068730177084,
0.325774599264223,0.327856094682295,0.329629722149541),.UNSPECIFIED.);
#1512=B_SPLINE_CURVE_WITH_KNOTS('',3,(#26093,#26094,#26095,#26096,#26097,
#26098,#26099,#26100,#26101,#26102,#26103,#26104,#26105,#26106,#26107,#26108,
#26109,#26110,#26111,#26112,#26113,#26114,#26115,#26116,#26117,#26118,#26119,
#26120,#26121,#26122,#26123,#26124,#26125,#26126,#26127,#26128,#26129,#26130,
#26131,#26132,#26133,#26134,#26135,#26136,#26137,#26138),.UNSPECIFIED.,
 .F.,.F.,(4,3,3,3,3,3,3,3,3,3,3,3,3,3,3,4),(95.7916386070333,95.90709073475,
96.0227926009489,96.1389321454556,96.2444160663824,96.3525294056605,96.4637895762893,
96.5716115215476,96.6793694345904,96.7871019690566,96.8948477359185,97.0027147634683,
97.1106552609226,97.2187783742407,97.2426107706909,97.3893722612835),
 .UNSPECIFIED.);
#1513=B_SPLINE_CURVE_WITH_KNOTS('',3,(#26146,#26147,#26148,#26149,#26150,
#26151,#26152,#26153,#26154,#26155,#26156,#26157,#26158,#26159,#26160,#26161,
#26162,#26163,#26164,#26165,#26166,#26167,#26168,#26169,#26170,#26171,#26172,
#26173,#26174,#26175,#26176,#26177,#26178,#26179,#26180,#26181,#26182,#26183,
#26184,#26185,#26186,#26187,#26188,#26189,#26190,#26191,#26192,#26193,#26194,
#26195,#26196,#26197,#26198,#26199,#26200,#26201,#26202,#26203,#26204,#26205,
#26206,#26207,#26208,#26209,#26210,#26211,#26212,#26213,#26214,#26215,#26216,
#26217,#26218,#26219,#26220,#26221,#26222,#26223,#26224,#26225,#26226,#26227,
#26228,#26229,#26230,#26231,#26232,#26233,#26234,#26235,#26236,#26237,#26238,
#26239,#26240,#26241,#26242,#26243,#26244,#26245,#26246,#26247,#26248,#26249,
#26250,#26251,#26252,#26253,#26254,#26255,#26256,#26257,#26258,#26259,#26260,
#26261,#26262,#26263,#26264,#26265,#26266,#26267,#26268,#26269,#26270,#26271,
#26272,#26273,#26274,#26275,#26276,#26277,#26278,#26279,#26280,#26281,#26282,
#26283,#26284,#26285,#26286,#26287,#26288,#26289,#26290,#26291,#26292,#26293,
#26294,#26295,#26296,#26297,#26298,#26299,#26300,#26301,#26302,#26303,#26304,
#26305,#26306,#26307,#26308,#26309,#26310,#26311,#26312,#26313,#26314,#26315,
#26316,#26317,#26318,#26319,#26320,#26321,#26322,#26323,#26324,#26325,#26326),
 .UNSPECIFIED.,.F.,.F.,(4,3,3,3,3,3,3,3,3,3,3,3,3,3,3,3,3,3,3,3,3,3,3,3,
3,3,3,3,3,3,3,3,3,3,3,3,3,3,3,3,3,3,3,3,3,3,3,3,3,3,3,3,3,3,3,3,3,3,3,3,
4),(77.7119313453268,77.8591869360628,77.9615391956776,78.0637410289376,
78.165823297785,78.2678407930593,78.3698265486816,78.4718135562898,78.5739050791433,
78.6760500242308,78.7783777791865,78.8573816403713,78.9597691695305,79.0620062241828,
79.1641234778989,79.2661757966064,79.3681961664517,79.4702175311155,79.5723427771074,
79.6745211468974,79.7768814598886,79.8555763446798,79.9579596081616,80.0601927548315,
80.1623066471868,80.2643559400271,80.3663736207563,80.4683926346484,80.5705160644065,
80.6726929115159,80.7750521951542,80.8537710489883,80.9560238596925,81.0581259805397,
81.1601086101123,81.2620265559288,81.363912988911,81.4658010378375,81.567794847017,
81.669842611414,81.7720751652035,81.8519657532968,81.9545178689531,82.056919116762,
82.1591991976819,82.2614134219783,82.3635945480862,82.4657752909354,82.5680566830683,
82.6703896429752,82.7729002617409,82.8501604576053,82.9514894633638,83.0544770780961,
83.1555435477812,83.2565511171417,83.3575340696214,83.4619981475216,83.5630941776532,
83.6692422794376,83.7753903812219),.UNSPECIFIED.);
#1514=B_SPLINE_CURVE_WITH_KNOTS('',3,(#26329,#26330,#26331,#26332,#26333,
#26334,#26335,#26336,#26337,#26338,#26339,#26340,#26341,#26342,#26343,#26344,
#26345,#26346,#26347,#26348,#26349,#26350,#26351,#26352,#26353,#26354,#26355,
#26356,#26357,#26358,#26359,#26360,#26361,#26362,#26363,#26364,#26365,#26366,
#26367,#26368,#26369,#26370,#26371,#26372,#26373,#26374,#26375,#26376,#26377,
#26378,#26379,#26380,#26381,#26382,#26383,#26384,#26385,#26386,#26387,#26388,
#26389,#26390,#26391,#26392,#26393,#26394,#26395,#26396,#26397,#26398,#26399,
#26400,#26401,#26402,#26403,#26404,#26405,#26406,#26407,#26408,#26409,#26410,
#26411,#26412,#26413,#26414,#26415,#26416,#26417,#26418,#26419,#26420,#26421,
#26422,#26423,#26424,#26425,#26426,#26427,#26428,#26429,#26430,#26431,#26432,
#26433,#26434,#26435,#26436,#26437,#26438,#26439,#26440,#26441,#26442,#26443,
#26444,#26445,#26446,#26447,#26448,#26449,#26450,#26451,#26452,#26453,#26454,
#26455,#26456,#26457,#26458,#26459,#26460,#26461,#26462,#26463,#26464,#26465,
#26466,#26467,#26468,#26469,#26470,#26471,#26472,#26473,#26474,#26475,#26476,
#26477,#26478,#26479,#26480,#26481,#26482),.UNSPECIFIED.,.F.,.F.,(4,3,3,
3,3,3,3,3,3,3,3,3,3,3,3,3,3,3,3,3,3,3,3,3,3,3,3,3,3,3,3,3,3,3,3,3,3,3,3,
3,3,3,3,3,3,3,3,3,3,3,3,4),(-85.8447445705308,-85.7400831110115,-85.6354889468789,
-85.5309076570425,-85.4263287010924,-85.3217250850249,-85.2170697942132,
-85.1122558989224,-85.0073555350632,-84.9022530950634,-84.8465498662224,
-84.7450804571866,-84.6437754871337,-84.5426070737962,-84.4415135370295,
-84.3404606582202,-84.2394142729296,-84.1382691275365,-84.0370754030879,
-83.9356960178488,-83.8483551619139,-83.7459059067046,-83.643607801843,
-83.5414308389324,-83.4393196685829,-83.3372413992224,-83.2351631826449,
-83.1329831398502,-83.030751029681,-82.9283393507923,-82.8501604576054,
-82.7476259452047,-82.6452384015215,-82.5429661432666,-82.4407561340788,
-82.338575621552,-82.2363918932184,-82.1341019724148,-82.0317573913236,
-81.9292302304148,-81.8519657532969,-81.7497073069701,-81.647600809257,
-81.5456157032775,-81.4436964451327,-81.3418098618395,-81.2399228237298,
-81.1379318179721,-81.0358878546504,-80.9336606981718,-80.8537710489884,
-80.6873799771529),.UNSPECIFIED.);
#1515=B_SPLINE_CURVE_WITH_KNOTS('',3,(#26859,#26860,#26861,#26862,#26863,
#26864,#26865,#26866,#26867,#26868,#26869,#26870,#26871,#26872,#26873,#26874,
#26875,#26876,#26877,#26878,#26879,#26880,#26881,#26882,#26883,#26884,#26885,
#26886,#26887,#26888,#26889,#26890,#26891,#26892,#26893,#26894,#26895,#26896,
#26897,#26898,#26899,#26900,#26901,#26902,#26903,#26904,#26905,#26906,#26907,
#26908,#26909,#26910,#26911,#26912,#26913,#26914,#26915,#26916,#26917,#26918,
#26919,#26920,#26921,#26922,#26923,#26924,#26925,#26926,#26927,#26928,#26929,
#26930,#26931,#26932,#26933,#26934,#26935,#26936,#26937,#26938,#26939,#26940),
 .UNSPECIFIED.,.F.,.F.,(4,3,3,3,3,3,3,3,3,3,3,3,3,3,3,3,3,3,3,3,3,3,3,3,
3,3,3,4),(0.,0.0160334974104419,0.0395642075561535,0.0633644118263318,0.0837263817738086,
0.0874470583914756,0.110604406527102,0.133695295125757,0.156786183724411,
0.165329376229777,0.169027049684205,0.19120783931272,0.212732869209134,
0.226227078758941,0.24288151240858,0.246186438911864,0.267772589721302,
0.289583909371892,0.305496742371809,0.315196008042082,0.319047580844878,
0.340135104073168,0.359186757307379,0.366235629765007,0.370741076209788,
0.390853652067857,0.410818111358785,0.415993328865216),.UNSPECIFIED.);
#1516=B_SPLINE_CURVE_WITH_KNOTS('',3,(#26942,#26943,#26944,#26945,#26946,
#26947,#26948,#26949,#26950,#26951,#26952,#26953,#26954,#26955,#26956,#26957,
#26958,#26959,#26960,#26961,#26962,#26963,#26964,#26965,#26966,#26967,#26968,
#26969,#26970,#26971,#26972,#26973,#26974,#26975,#26976,#26977,#26978,#26979,
#26980,#26981,#26982,#26983,#26984,#26985,#26986,#26987,#26988,#26989,#26990,
#26991,#26992,#26993,#26994,#26995,#26996,#26997,#26998,#26999,#27000,#27001,
#27002,#27003,#27004,#27005,#27006,#27007,#27008,#27009,#27010,#27011,#27012,
#27013,#27014,#27015,#27016,#27017,#27018,#27019,#27020,#27021,#27022,#27023),
 .UNSPECIFIED.,.F.,.F.,(4,3,3,3,3,3,3,3,3,3,3,3,3,3,3,3,3,3,3,3,3,3,3,3,
3,3,3,4),(-0.415993328865187,-0.402901270545643,-0.382908564831211,-0.371774763313882,
-0.367435224694355,-0.346675516489467,-0.32591580828458,-0.321433315753078,
-0.315781547589586,-0.294240898198231,-0.27242808429252,-0.250757332701903,
-0.244873415404794,-0.24111480505867,-0.218638203108128,-0.211619958938312,
-0.189699687125207,-0.167779415312101,-0.162843814523672,-0.14037333732053,
-0.117486011716815,-0.0943539309902553,-0.0856507589901794,-0.0817563326016671,
-0.0580189261111904,-0.0342375412874052,-0.010964771881335,0.),
 .UNSPECIFIED.);
#1517=B_SPLINE_CURVE_WITH_KNOTS('',3,(#27024,#27025,#27026,#27027),
 .UNSPECIFIED.,.F.,.F.,(4,4),(-0.013270419803488,0.),.UNSPECIFIED.);
#1518=B_SPLINE_CURVE_WITH_KNOTS('',3,(#27029,#27030,#27031,#27032,#27033,
#27034,#27035,#27036,#27037,#27038,#27039,#27040,#27041,#27042,#27043,#27044,
#27045,#27046,#27047,#27048,#27049,#27050,#27051,#27052,#27053,#27054,#27055,
#27056,#27057,#27058,#27059,#27060,#27061,#27062,#27063,#27064,#27065,#27066,
#27067,#27068,#27069,#27070,#27071,#27072,#27073,#27074,#27075,#27076,#27077,
#27078,#27079,#27080,#27081,#27082,#27083,#27084,#27085,#27086,#27087,#27088,
#27089,#27090,#27091,#27092,#27093,#27094,#27095,#27096,#27097,#27098,#27099,
#27100,#27101,#27102,#27103,#27104,#27105,#27106,#27107,#27108,#27109,#27110,
#27111,#27112,#27113,#27114,#27115,#27116),.UNSPECIFIED.,.F.,.F.,(4,3,3,
3,3,3,3,3,3,3,3,3,3,3,3,3,3,3,3,3,3,3,3,3,3,3,3,3,3,4),(-0.410048543780163,
-0.398139186466655,-0.374410169279448,-0.362901775202635,-0.357252904496043,
-0.353226071091677,-0.329831664546775,-0.312242260164576,-0.303769719034645,
-0.299630020912383,-0.276842045832635,-0.254514602197622,-0.232670178061085,
-0.225307920334055,-0.221146019951397,-0.21755552666877,-0.195982423127032,
-0.189116736674495,-0.166997686104259,-0.146198385794381,-0.141443407849317,
-0.12001432471249,-0.0987103641811844,-0.0775869942730841,-0.0725417907976872,
-0.0674800293840683,-0.0468865361744227,-0.0269015552315733,-0.00767557047989959,
0.),.UNSPECIFIED.);
#1519=B_SPLINE_CURVE_WITH_KNOTS('',3,(#27474,#27475,#27476,#27477,#27478,
#27479,#27480,#27481,#27482,#27483,#27484,#27485,#27486,#27487,#27488,#27489,
#27490,#27491,#27492,#27493,#27494,#27495,#27496,#27497,#27498,#27499,#27500,
#27501,#27502,#27503,#27504,#27505,#27506,#27507,#27508,#27509,#27510,#27511,
#27512,#27513,#27514,#27515,#27516,#27517,#27518,#27519,#27520,#27521,#27522,
#27523,#27524,#27525,#27526,#27527,#27528,#27529,#27530,#27531,#27532,#27533,
#27534,#27535,#27536,#27537,#27538,#27539,#27540,#27541,#27542,#27543,#27544,
#27545,#27546,#27547,#27548,#27549,#27550,#27551,#27552,#27553,#27554,#27555,
#27556,#27557,#27558,#27559,#27560,#27561),.UNSPECIFIED.,.F.,.F.,(4,3,3,
3,3,3,3,3,3,3,3,3,3,3,3,3,3,3,3,3,3,3,3,3,3,3,3,3,3,4),(0.,0.0130464519754968,
0.0327301024266493,0.0529569041528836,0.0626751748968586,0.0683819350422815,
0.0728898740513483,0.0938311318830955,0.115156107462477,0.136611032509031,
0.143309507195499,0.146634619759991,0.168716970870795,0.190720450842287,
0.203657142534596,0.22030049657604,0.223957438687906,0.245741331031745,
0.268250311172619,0.290759291313493,0.295289317391233,0.299519479633725,
0.303835795791196,0.327161928089292,0.350378655359791,0.356293009821619,
0.360744190415631,0.384491412450957,0.408026460803736,0.414097116159586),
 .UNSPECIFIED.);
#1520=B_SPLINE_CURVE_WITH_KNOTS('',3,(#27562,#27563,#27564,#27565),
 .UNSPECIFIED.,.F.,.F.,(4,4),(0.,0.0132705018374832),.UNSPECIFIED.);
#1782=VERTEX_POINT('',#15720);
#1783=VERTEX_POINT('',#15721);
#1784=VERTEX_POINT('',#15723);
#1785=VERTEX_POINT('',#15728);
#1786=VERTEX_POINT('',#15853);
#1787=VERTEX_POINT('',#15860);
#1788=VERTEX_POINT('',#15862);
#1789=VERTEX_POINT('',#15865);
#1790=VERTEX_POINT('',#15937);
#1791=VERTEX_POINT('',#15938);
#1792=VERTEX_POINT('',#15976);
#1793=VERTEX_POINT('',#15977);
#1794=VERTEX_POINT('',#16400);
#1795=VERTEX_POINT('',#16401);
#1796=VERTEX_POINT('',#16800);
#1797=VERTEX_POINT('',#16801);
#1798=VERTEX_POINT('',#16803);
#1799=VERTEX_POINT('',#17018);
#1800=VERTEX_POINT('',#17234);
#1801=VERTEX_POINT('',#17235);
#1802=VERTEX_POINT('',#17237);
#1803=VERTEX_POINT('',#17442);
#1804=VERTEX_POINT('',#17646);
#1805=VERTEX_POINT('',#17647);
#1806=VERTEX_POINT('',#18050);
#1807=VERTEX_POINT('',#18051);
#1808=VERTEX_POINT('',#18053);
#1809=VERTEX_POINT('',#18258);
#1810=VERTEX_POINT('',#18468);
#1811=VERTEX_POINT('',#18469);
#1812=VERTEX_POINT('',#18870);
#1813=VERTEX_POINT('',#18871);
#1814=VERTEX_POINT('',#19294);
#1815=VERTEX_POINT('',#19295);
#1816=VERTEX_POINT('',#19297);
#1817=VERTEX_POINT('',#19496);
#1818=VERTEX_POINT('',#19718);
#1819=VERTEX_POINT('',#19719);
#1820=VERTEX_POINT('',#19721);
#1821=VERTEX_POINT('',#19932);
#1822=VERTEX_POINT('',#20144);
#1823=VERTEX_POINT('',#20145);
#1824=VERTEX_POINT('',#20552);
#1825=VERTEX_POINT('',#20553);
#1826=VERTEX_POINT('',#20958);
#1827=VERTEX_POINT('',#20959);
#1828=VERTEX_POINT('',#20961);
#1829=VERTEX_POINT('',#21112);
#1830=VERTEX_POINT('',#21257);
#1831=VERTEX_POINT('',#21258);
#1832=VERTEX_POINT('',#21633);
#1833=VERTEX_POINT('',#21634);
#1834=VERTEX_POINT('',#21636);
#1835=VERTEX_POINT('',#22034);
#1836=VERTEX_POINT('',#22035);
#1837=VERTEX_POINT('',#22416);
#1838=VERTEX_POINT('',#22417);
#1839=VERTEX_POINT('',#22802);
#1840=VERTEX_POINT('',#22803);
#1841=VERTEX_POINT('',#23194);
#1842=VERTEX_POINT('',#23195);
#1843=VERTEX_POINT('',#23576);
#1844=VERTEX_POINT('',#23577);
#1845=VERTEX_POINT('',#23966);
#1846=VERTEX_POINT('',#23967);
#1847=VERTEX_POINT('',#24344);
#1848=VERTEX_POINT('',#24345);
#1849=VERTEX_POINT('',#24730);
#1850=VERTEX_POINT('',#24731);
#1851=VERTEX_POINT('',#25114);
#1852=VERTEX_POINT('',#25115);
#1853=VERTEX_POINT('',#25309);
#1854=VERTEX_POINT('',#25505);
#1855=VERTEX_POINT('',#25506);
#1856=VERTEX_POINT('',#25893);
#1857=VERTEX_POINT('',#26030);
#1858=VERTEX_POINT('',#26032);
#1859=VERTEX_POINT('',#26140);
#1860=VERTEX_POINT('',#26145);
#1861=VERTEX_POINT('',#26327);
#1862=VERTEX_POINT('',#26484);
#1863=VERTEX_POINT('',#26486);
#1864=VERTEX_POINT('',#26489);
#1865=VERTEX_POINT('',#26491);
#1866=VERTEX_POINT('',#26495);
#1867=VERTEX_POINT('',#26501);
#1868=VERTEX_POINT('',#26941);
#1869=VERTEX_POINT('',#27473);
#1870=VERTEX_POINT('',#27568);
#1871=VERTEX_POINT('',#27570);
#1872=VERTEX_POINT('',#27574);
#1873=VERTEX_POINT('',#27579);
#1874=VERTEX_POINT('',#27581);
#1875=VERTEX_POINT('',#27585);
#1876=VERTEX_POINT('',#27590);
#1877=VERTEX_POINT('',#27594);
#1878=VERTEX_POINT('',#27597);
#1879=VERTEX_POINT('',#27599);
#1880=VERTEX_POINT('',#27603);
#1881=VERTEX_POINT('',#27607);
#1882=VERTEX_POINT('',#27612);
#1883=VERTEX_POINT('',#27616);
#1884=VERTEX_POINT('',#27620);
#1885=VERTEX_POINT('',#27624);
#1886=VERTEX_POINT('',#27627);
#1887=VERTEX_POINT('',#27629);
#1888=VERTEX_POINT('',#27633);
#1889=VERTEX_POINT('',#27637);
#1890=VERTEX_POINT('',#27640);
#1891=VERTEX_POINT('',#27644);
#1892=VERTEX_POINT('',#27647);
#1893=VERTEX_POINT('',#27649);
#2286=EDGE_CURVE('',#1782,#1783,#1052,.T.);
#2287=EDGE_CURVE('',#1782,#1784,#1442,.T.);
#2288=EDGE_CURVE('',#1784,#1785,#1443,.T.);
#2289=EDGE_CURVE('',#1785,#1786,#1444,.T.);
#2290=EDGE_CURVE('',#1786,#1787,#291,.T.);
#2291=EDGE_CURVE('',#1787,#1788,#1053,.T.);
#2292=EDGE_CURVE('',#1788,#1788,#292,.F.);
#2293=EDGE_CURVE('',#1787,#1789,#293,.T.);
#2294=EDGE_CURVE('',#1789,#1783,#1445,.T.);
#2295=EDGE_CURVE('',#1790,#1791,#1446,.T.);
#2296=EDGE_CURVE('',#1791,#1790,#1447,.T.);
#2297=EDGE_CURVE('',#1792,#1793,#1054,.T.);
#2298=EDGE_CURVE('',#1792,#1782,#1448,.T.);
#2299=EDGE_CURVE('',#1783,#1793,#1449,.T.);
#2300=EDGE_CURVE('',#1794,#1795,#1055,.T.);
#2301=EDGE_CURVE('',#1794,#1792,#1450,.T.);
#2302=EDGE_CURVE('',#1793,#1795,#1451,.T.);
#2303=EDGE_CURVE('',#1796,#1797,#1056,.T.);
#2304=EDGE_CURVE('',#1796,#1798,#1452,.T.);
#2305=EDGE_CURVE('',#1798,#1794,#1453,.T.);
#2306=EDGE_CURVE('',#1795,#1799,#1454,.T.);
#2307=EDGE_CURVE('',#1799,#1797,#1455,.T.);
#2308=EDGE_CURVE('',#1800,#1801,#1057,.T.);
#2309=EDGE_CURVE('',#1800,#1802,#1456,.T.);
#2310=EDGE_CURVE('',#1802,#1796,#1457,.T.);
#2311=EDGE_CURVE('',#1797,#1803,#1458,.T.);
#2312=EDGE_CURVE('',#1803,#1801,#1459,.T.);
#2313=EDGE_CURVE('',#1804,#1805,#1058,.T.);
#2314=EDGE_CURVE('',#1804,#1800,#1460,.T.);
#2315=EDGE_CURVE('',#1801,#1805,#1461,.T.);
#2316=EDGE_CURVE('',#1806,#1807,#1059,.T.);
#2317=EDGE_CURVE('',#1806,#1808,#1462,.T.);
#2318=EDGE_CURVE('',#1808,#1804,#1463,.T.);
#2319=EDGE_CURVE('',#1805,#1809,#1464,.T.);
#2320=EDGE_CURVE('',#1809,#1807,#1465,.T.);
#2321=EDGE_CURVE('',#1810,#1811,#1060,.T.);
#2322=EDGE_CURVE('',#1810,#1806,#1466,.T.);
#2323=EDGE_CURVE('',#1807,#1811,#1467,.T.);
#2324=EDGE_CURVE('',#1812,#1813,#1061,.T.);
#2325=EDGE_CURVE('',#1812,#1810,#1468,.T.);
#2326=EDGE_CURVE('',#1811,#1813,#1469,.T.);
#2327=EDGE_CURVE('',#1814,#1815,#1062,.T.);
#2328=EDGE_CURVE('',#1814,#1816,#1470,.T.);
#2329=EDGE_CURVE('',#1816,#1812,#1471,.T.);
#2330=EDGE_CURVE('',#1813,#1817,#1472,.T.);
#2331=EDGE_CURVE('',#1817,#1815,#1473,.T.);
#2332=EDGE_CURVE('',#1818,#1819,#1063,.T.);
#2333=EDGE_CURVE('',#1818,#1820,#1474,.T.);
#2334=EDGE_CURVE('',#1820,#1814,#1475,.T.);
#2335=EDGE_CURVE('',#1815,#1821,#1476,.T.);
#2336=EDGE_CURVE('',#1821,#1819,#1477,.T.);
#2337=EDGE_CURVE('',#1822,#1823,#1064,.T.);
#2338=EDGE_CURVE('',#1822,#1818,#1478,.T.);
#2339=EDGE_CURVE('',#1819,#1823,#1479,.T.);
#2340=EDGE_CURVE('',#1824,#1825,#1065,.T.);
#2341=EDGE_CURVE('',#1824,#1822,#1480,.T.);
#2342=EDGE_CURVE('',#1823,#1825,#1481,.T.);
#2343=EDGE_CURVE('',#1826,#1827,#1066,.T.);
#2344=EDGE_CURVE('',#1828,#1826,#1482,.F.);
#2345=EDGE_CURVE('',#1829,#1828,#294,.T.);
#2346=EDGE_CURVE('',#1829,#1827,#1483,.T.);
#2347=EDGE_CURVE('',#1830,#1831,#1067,.T.);
#2348=EDGE_CURVE('',#1826,#1830,#1484,.F.);
#2349=EDGE_CURVE('',#1827,#1831,#1485,.T.);
#2350=EDGE_CURVE('',#1832,#1833,#1068,.T.);
#2351=EDGE_CURVE('',#1834,#1832,#1486,.F.);
#2352=EDGE_CURVE('',#1830,#1834,#1487,.F.);
#2353=EDGE_CURVE('',#1831,#1833,#1488,.T.);
#2354=EDGE_CURVE('',#1835,#1836,#1069,.T.);
#2355=EDGE_CURVE('',#1832,#1835,#1489,.F.);
#2356=EDGE_CURVE('',#1833,#1836,#1490,.T.);
#2357=EDGE_CURVE('',#1837,#1838,#1070,.T.);
#2358=EDGE_CURVE('',#1835,#1837,#1491,.F.);
#2359=EDGE_CURVE('',#1836,#1838,#1492,.T.);
#2360=EDGE_CURVE('',#1839,#1840,#1071,.T.);
#2361=EDGE_CURVE('',#1837,#1839,#1493,.F.);
#2362=EDGE_CURVE('',#1838,#1840,#1494,.T.);
#2363=EDGE_CURVE('',#1841,#1842,#1072,.T.);
#2364=EDGE_CURVE('',#1839,#1841,#1495,.F.);
#2365=EDGE_CURVE('',#1840,#1842,#1496,.T.);
#2366=EDGE_CURVE('',#1843,#1844,#1073,.T.);
#2367=EDGE_CURVE('',#1841,#1843,#1497,.F.);
#2368=EDGE_CURVE('',#1842,#1844,#1498,.T.);
#2369=EDGE_CURVE('',#1845,#1846,#1074,.T.);
#2370=EDGE_CURVE('',#1843,#1845,#1499,.F.);
#2371=EDGE_CURVE('',#1844,#1846,#1500,.T.);
#2372=EDGE_CURVE('',#1847,#1848,#1075,.T.);
#2373=EDGE_CURVE('',#1845,#1847,#1501,.F.);
#2374=EDGE_CURVE('',#1846,#1848,#1502,.T.);
#2375=EDGE_CURVE('',#1849,#1850,#1076,.T.);
#2376=EDGE_CURVE('',#1847,#1849,#1503,.F.);
#2377=EDGE_CURVE('',#1848,#1850,#1504,.T.);
#2378=EDGE_CURVE('',#1851,#1852,#1077,.T.);
#2379=EDGE_CURVE('',#1849,#1851,#1505,.F.);
#2380=EDGE_CURVE('',#1850,#1853,#1506,.T.);
#2381=EDGE_CURVE('',#1853,#1852,#1507,.T.);
#2382=EDGE_CURVE('',#1854,#1855,#1078,.T.);
#2383=EDGE_CURVE('',#1851,#1854,#1508,.F.);
#2384=EDGE_CURVE('',#1852,#1855,#1509,.T.);
#2385=EDGE_CURVE('',#1855,#1856,#1510,.T.);
#2386=EDGE_CURVE('',#1857,#1856,#295,.T.);
#2387=EDGE_CURVE('',#1858,#1857,#1511,.T.);
#2388=EDGE_CURVE('',#1854,#1858,#1512,.T.);
#2389=EDGE_CURVE('',#1859,#1859,#296,.T.);
#2390=EDGE_CURVE('',#1859,#1791,#1079,.T.);
#2391=EDGE_CURVE('',#1825,#1860,#1513,.T.);
#2392=EDGE_CURVE('',#1861,#1860,#297,.F.);
#2393=EDGE_CURVE('',#1861,#1824,#1514,.T.);
#2394=EDGE_CURVE('',#1862,#1862,#298,.T.);
#2395=EDGE_CURVE('',#1863,#1863,#299,.T.);
#2396=EDGE_CURVE('',#1864,#1864,#300,.T.);
#2397=EDGE_CURVE('',#1864,#1865,#301,.T.);
#2398=EDGE_CURVE('',#1865,#1865,#302,.T.);
#2399=EDGE_CURVE('',#1865,#1866,#1080,.T.);
#2400=EDGE_CURVE('',#1866,#1866,#303,.T.);
#2401=EDGE_CURVE('',#1866,#1862,#304,.T.);
#2402=EDGE_CURVE('',#1867,#1867,#305,.T.);
#2403=EDGE_CURVE('',#1860,#1857,#1515,.T.);
#2404=EDGE_CURVE('',#1868,#1789,#1516,.T.);
#2405=EDGE_CURVE('',#1868,#1828,#1517,.T.);
#2406=EDGE_CURVE('',#1786,#1829,#1518,.T.);
#2407=EDGE_CURVE('',#1869,#1861,#1519,.T.);
#2408=EDGE_CURVE('',#1856,#1869,#1520,.T.);
#2409=EDGE_CURVE('',#1870,#1870,#306,.T.);
#2410=EDGE_CURVE('',#1870,#1871,#307,.T.);
#2411=EDGE_CURVE('',#1871,#1871,#308,.T.);
#2412=EDGE_CURVE('',#1871,#1872,#1081,.T.);
#2413=EDGE_CURVE('',#1872,#1872,#309,.T.);
#2414=EDGE_CURVE('',#1873,#1873,#310,.T.);
#2415=EDGE_CURVE('',#1873,#1874,#311,.T.);
#2416=EDGE_CURVE('',#1874,#1874,#312,.T.);
#2417=EDGE_CURVE('',#1874,#1875,#1082,.T.);
#2418=EDGE_CURVE('',#1875,#1875,#313,.T.);
#2419=EDGE_CURVE('',#1875,#1876,#314,.T.);
#2420=EDGE_CURVE('',#1876,#1876,#315,.T.);
#2421=EDGE_CURVE('',#1877,#1877,#316,.T.);
#2422=EDGE_CURVE('',#1878,#1878,#317,.T.);
#2423=EDGE_CURVE('',#1878,#1879,#318,.T.);
#2424=EDGE_CURVE('',#1879,#1879,#319,.T.);
#2425=EDGE_CURVE('',#1879,#1880,#1083,.T.);
#2426=EDGE_CURVE('',#1880,#1880,#320,.T.);
#2427=EDGE_CURVE('',#1881,#1881,#321,.T.);
#2428=EDGE_CURVE('',#1880,#1867,#322,.T.);
#2429=EDGE_CURVE('',#1863,#1882,#323,.T.);
#2430=EDGE_CURVE('',#1882,#1882,#324,.T.);
#2431=EDGE_CURVE('',#1882,#1883,#1084,.T.);
#2432=EDGE_CURVE('',#1883,#1883,#325,.T.);
#2433=EDGE_CURVE('',#1883,#1884,#326,.T.);
#2434=EDGE_CURVE('',#1884,#1884,#327,.T.);
#2435=EDGE_CURVE('',#1885,#1885,#328,.T.);
#2436=EDGE_CURVE('',#1886,#1886,#329,.T.);
#2437=EDGE_CURVE('',#1886,#1887,#330,.T.);
#2438=EDGE_CURVE('',#1887,#1887,#331,.T.);
#2439=EDGE_CURVE('',#1887,#1888,#1085,.T.);
#2440=EDGE_CURVE('',#1888,#1888,#332,.T.);
#2441=EDGE_CURVE('',#1889,#1889,#333,.T.);
#2442=EDGE_CURVE('',#1888,#1890,#334,.T.);
#2443=EDGE_CURVE('',#1890,#1890,#335,.T.);
#2444=EDGE_CURVE('',#1891,#1891,#336,.T.);
#2445=EDGE_CURVE('',#1892,#1892,#337,.T.);
#2446=EDGE_CURVE('',#1892,#1893,#338,.T.);
#2447=EDGE_CURVE('',#1893,#1893,#339,.T.);
#2448=EDGE_CURVE('',#1891,#1892,#1086,.T.);
#2449=EDGE_CURVE('',#1885,#1889,#1087,.T.);
#2450=EDGE_CURVE('',#1877,#1881,#1088,.T.);
#3233=ORIENTED_EDGE('',*,*,#2286,.F.);
#3234=ORIENTED_EDGE('',*,*,#2287,.T.);
#3235=ORIENTED_EDGE('',*,*,#2288,.T.);
#3236=ORIENTED_EDGE('',*,*,#2289,.T.);
#3237=ORIENTED_EDGE('',*,*,#2290,.T.);
#3238=ORIENTED_EDGE('',*,*,#2291,.T.);
#3239=ORIENTED_EDGE('',*,*,#2292,.T.);
#3240=ORIENTED_EDGE('',*,*,#2291,.F.);
#3241=ORIENTED_EDGE('',*,*,#2293,.T.);
#3242=ORIENTED_EDGE('',*,*,#2294,.T.);
#3243=ORIENTED_EDGE('',*,*,#2295,.T.);
#3244=ORIENTED_EDGE('',*,*,#2296,.T.);
#3245=ORIENTED_EDGE('',*,*,#2297,.F.);
#3246=ORIENTED_EDGE('',*,*,#2298,.T.);
#3247=ORIENTED_EDGE('',*,*,#2286,.T.);
#3248=ORIENTED_EDGE('',*,*,#2299,.T.);
#3249=ORIENTED_EDGE('',*,*,#2300,.F.);
#3250=ORIENTED_EDGE('',*,*,#2301,.T.);
#3251=ORIENTED_EDGE('',*,*,#2297,.T.);
#3252=ORIENTED_EDGE('',*,*,#2302,.T.);
#3253=ORIENTED_EDGE('',*,*,#2303,.F.);
#3254=ORIENTED_EDGE('',*,*,#2304,.T.);
#3255=ORIENTED_EDGE('',*,*,#2305,.T.);
#3256=ORIENTED_EDGE('',*,*,#2300,.T.);
#3257=ORIENTED_EDGE('',*,*,#2306,.T.);
#3258=ORIENTED_EDGE('',*,*,#2307,.T.);
#3259=ORIENTED_EDGE('',*,*,#2308,.F.);
#3260=ORIENTED_EDGE('',*,*,#2309,.T.);
#3261=ORIENTED_EDGE('',*,*,#2310,.T.);
#3262=ORIENTED_EDGE('',*,*,#2303,.T.);
#3263=ORIENTED_EDGE('',*,*,#2311,.T.);
#3264=ORIENTED_EDGE('',*,*,#2312,.T.);
#3265=ORIENTED_EDGE('',*,*,#2313,.F.);
#3266=ORIENTED_EDGE('',*,*,#2314,.T.);
#3267=ORIENTED_EDGE('',*,*,#2308,.T.);
#3268=ORIENTED_EDGE('',*,*,#2315,.T.);
#3269=ORIENTED_EDGE('',*,*,#2316,.F.);
#3270=ORIENTED_EDGE('',*,*,#2317,.T.);
#3271=ORIENTED_EDGE('',*,*,#2318,.T.);
#3272=ORIENTED_EDGE('',*,*,#2313,.T.);
#3273=ORIENTED_EDGE('',*,*,#2319,.T.);
#3274=ORIENTED_EDGE('',*,*,#2320,.T.);
#3275=ORIENTED_EDGE('',*,*,#2321,.F.);
#3276=ORIENTED_EDGE('',*,*,#2322,.T.);
#3277=ORIENTED_EDGE('',*,*,#2316,.T.);
#3278=ORIENTED_EDGE('',*,*,#2323,.T.);
#3279=ORIENTED_EDGE('',*,*,#2324,.F.);
#3280=ORIENTED_EDGE('',*,*,#2325,.T.);
#3281=ORIENTED_EDGE('',*,*,#2321,.T.);
#3282=ORIENTED_EDGE('',*,*,#2326,.T.);
#3283=ORIENTED_EDGE('',*,*,#2327,.F.);
#3284=ORIENTED_EDGE('',*,*,#2328,.T.);
#3285=ORIENTED_EDGE('',*,*,#2329,.T.);
#3286=ORIENTED_EDGE('',*,*,#2324,.T.);
#3287=ORIENTED_EDGE('',*,*,#2330,.T.);
#3288=ORIENTED_EDGE('',*,*,#2331,.T.);
#3289=ORIENTED_EDGE('',*,*,#2332,.F.);
#3290=ORIENTED_EDGE('',*,*,#2333,.T.);
#3291=ORIENTED_EDGE('',*,*,#2334,.T.);
#3292=ORIENTED_EDGE('',*,*,#2327,.T.);
#3293=ORIENTED_EDGE('',*,*,#2335,.T.);
#3294=ORIENTED_EDGE('',*,*,#2336,.T.);
#3295=ORIENTED_EDGE('',*,*,#2337,.F.);
#3296=ORIENTED_EDGE('',*,*,#2338,.T.);
#3297=ORIENTED_EDGE('',*,*,#2332,.T.);
#3298=ORIENTED_EDGE('',*,*,#2339,.T.);
#3299=ORIENTED_EDGE('',*,*,#2340,.F.);
#3300=ORIENTED_EDGE('',*,*,#2341,.T.);
#3301=ORIENTED_EDGE('',*,*,#2337,.T.);
#3302=ORIENTED_EDGE('',*,*,#2342,.T.);
#3303=ORIENTED_EDGE('',*,*,#2343,.F.);
#3304=ORIENTED_EDGE('',*,*,#2344,.F.);
#3305=ORIENTED_EDGE('',*,*,#2345,.F.);
#3306=ORIENTED_EDGE('',*,*,#2346,.T.);
#3307=ORIENTED_EDGE('',*,*,#2347,.F.);
#3308=ORIENTED_EDGE('',*,*,#2348,.F.);
#3309=ORIENTED_EDGE('',*,*,#2343,.T.);
#3310=ORIENTED_EDGE('',*,*,#2349,.T.);
#3311=ORIENTED_EDGE('',*,*,#2350,.F.);
#3312=ORIENTED_EDGE('',*,*,#2351,.F.);
#3313=ORIENTED_EDGE('',*,*,#2352,.F.);
#3314=ORIENTED_EDGE('',*,*,#2347,.T.);
#3315=ORIENTED_EDGE('',*,*,#2353,.T.);
#3316=ORIENTED_EDGE('',*,*,#2354,.F.);
#3317=ORIENTED_EDGE('',*,*,#2355,.F.);
#3318=ORIENTED_EDGE('',*,*,#2350,.T.);
#3319=ORIENTED_EDGE('',*,*,#2356,.T.);
#3320=ORIENTED_EDGE('',*,*,#2357,.F.);
#3321=ORIENTED_EDGE('',*,*,#2358,.F.);
#3322=ORIENTED_EDGE('',*,*,#2354,.T.);
#3323=ORIENTED_EDGE('',*,*,#2359,.T.);
#3324=ORIENTED_EDGE('',*,*,#2360,.F.);
#3325=ORIENTED_EDGE('',*,*,#2361,.F.);
#3326=ORIENTED_EDGE('',*,*,#2357,.T.);
#3327=ORIENTED_EDGE('',*,*,#2362,.T.);
#3328=ORIENTED_EDGE('',*,*,#2363,.F.);
#3329=ORIENTED_EDGE('',*,*,#2364,.F.);
#3330=ORIENTED_EDGE('',*,*,#2360,.T.);
#3331=ORIENTED_EDGE('',*,*,#2365,.T.);
#3332=ORIENTED_EDGE('',*,*,#2366,.F.);
#3333=ORIENTED_EDGE('',*,*,#2367,.F.);
#3334=ORIENTED_EDGE('',*,*,#2363,.T.);
#3335=ORIENTED_EDGE('',*,*,#2368,.T.);
#3336=ORIENTED_EDGE('',*,*,#2369,.F.);
#3337=ORIENTED_EDGE('',*,*,#2370,.F.);
#3338=ORIENTED_EDGE('',*,*,#2366,.T.);
#3339=ORIENTED_EDGE('',*,*,#2371,.T.);
#3340=ORIENTED_EDGE('',*,*,#2372,.F.);
#3341=ORIENTED_EDGE('',*,*,#2373,.F.);
#3342=ORIENTED_EDGE('',*,*,#2369,.T.);
#3343=ORIENTED_EDGE('',*,*,#2374,.T.);
#3344=ORIENTED_EDGE('',*,*,#2375,.F.);
#3345=ORIENTED_EDGE('',*,*,#2376,.F.);
#3346=ORIENTED_EDGE('',*,*,#2372,.T.);
#3347=ORIENTED_EDGE('',*,*,#2377,.T.);
#3348=ORIENTED_EDGE('',*,*,#2378,.F.);
#3349=ORIENTED_EDGE('',*,*,#2379,.F.);
#3350=ORIENTED_EDGE('',*,*,#2375,.T.);
#3351=ORIENTED_EDGE('',*,*,#2380,.T.);
#3352=ORIENTED_EDGE('',*,*,#2381,.T.);
#3353=ORIENTED_EDGE('',*,*,#2382,.F.);
#3354=ORIENTED_EDGE('',*,*,#2383,.F.);
#3355=ORIENTED_EDGE('',*,*,#2378,.T.);
#3356=ORIENTED_EDGE('',*,*,#2384,.T.);
#3357=ORIENTED_EDGE('',*,*,#2382,.T.);
#3358=ORIENTED_EDGE('',*,*,#2385,.T.);
#3359=ORIENTED_EDGE('',*,*,#2386,.F.);
#3360=ORIENTED_EDGE('',*,*,#2387,.F.);
#3361=ORIENTED_EDGE('',*,*,#2388,.F.);
#3362=ORIENTED_EDGE('',*,*,#2389,.F.);
#3363=ORIENTED_EDGE('',*,*,#2390,.T.);
#3364=ORIENTED_EDGE('',*,*,#2295,.F.);
#3365=ORIENTED_EDGE('',*,*,#2296,.F.);
#3366=ORIENTED_EDGE('',*,*,#2390,.F.);
#3367=ORIENTED_EDGE('',*,*,#2389,.T.);
#3368=ORIENTED_EDGE('',*,*,#2340,.T.);
#3369=ORIENTED_EDGE('',*,*,#2391,.T.);
#3370=ORIENTED_EDGE('',*,*,#2392,.F.);
#3371=ORIENTED_EDGE('',*,*,#2393,.T.);
#3372=ORIENTED_EDGE('',*,*,#2394,.F.);
#3373=ORIENTED_EDGE('',*,*,#2395,.F.);
#3374=ORIENTED_EDGE('',*,*,#2396,.T.);
#3375=ORIENTED_EDGE('',*,*,#2397,.T.);
#3376=ORIENTED_EDGE('',*,*,#2398,.T.);
#3377=ORIENTED_EDGE('',*,*,#2397,.F.);
#3378=ORIENTED_EDGE('',*,*,#2398,.F.);
#3379=ORIENTED_EDGE('',*,*,#2399,.T.);
#3380=ORIENTED_EDGE('',*,*,#2400,.F.);
#3381=ORIENTED_EDGE('',*,*,#2399,.F.);
#3382=ORIENTED_EDGE('',*,*,#2400,.T.);
#3383=ORIENTED_EDGE('',*,*,#2401,.T.);
#3384=ORIENTED_EDGE('',*,*,#2394,.T.);
#3385=ORIENTED_EDGE('',*,*,#2401,.F.);
#3386=ORIENTED_EDGE('',*,*,#2402,.F.);
#3387=ORIENTED_EDGE('',*,*,#2396,.F.);
#3388=ORIENTED_EDGE('',*,*,#2403,.F.);
#3389=ORIENTED_EDGE('',*,*,#2391,.F.);
#3390=ORIENTED_EDGE('',*,*,#2342,.F.);
#3391=ORIENTED_EDGE('',*,*,#2339,.F.);
#3392=ORIENTED_EDGE('',*,*,#2336,.F.);
#3393=ORIENTED_EDGE('',*,*,#2335,.F.);
#3394=ORIENTED_EDGE('',*,*,#2331,.F.);
#3395=ORIENTED_EDGE('',*,*,#2330,.F.);
#3396=ORIENTED_EDGE('',*,*,#2326,.F.);
#3397=ORIENTED_EDGE('',*,*,#2323,.F.);
#3398=ORIENTED_EDGE('',*,*,#2320,.F.);
#3399=ORIENTED_EDGE('',*,*,#2319,.F.);
#3400=ORIENTED_EDGE('',*,*,#2315,.F.);
#3401=ORIENTED_EDGE('',*,*,#2312,.F.);
#3402=ORIENTED_EDGE('',*,*,#2311,.F.);
#3403=ORIENTED_EDGE('',*,*,#2307,.F.);
#3404=ORIENTED_EDGE('',*,*,#2306,.F.);
#3405=ORIENTED_EDGE('',*,*,#2302,.F.);
#3406=ORIENTED_EDGE('',*,*,#2299,.F.);
#3407=ORIENTED_EDGE('',*,*,#2294,.F.);
#3408=ORIENTED_EDGE('',*,*,#2404,.F.);
#3409=ORIENTED_EDGE('',*,*,#2405,.T.);
#3410=ORIENTED_EDGE('',*,*,#2344,.T.);
#3411=ORIENTED_EDGE('',*,*,#2348,.T.);
#3412=ORIENTED_EDGE('',*,*,#2352,.T.);
#3413=ORIENTED_EDGE('',*,*,#2351,.T.);
#3414=ORIENTED_EDGE('',*,*,#2355,.T.);
#3415=ORIENTED_EDGE('',*,*,#2358,.T.);
#3416=ORIENTED_EDGE('',*,*,#2361,.T.);
#3417=ORIENTED_EDGE('',*,*,#2364,.T.);
#3418=ORIENTED_EDGE('',*,*,#2367,.T.);
#3419=ORIENTED_EDGE('',*,*,#2370,.T.);
#3420=ORIENTED_EDGE('',*,*,#2373,.T.);
#3421=ORIENTED_EDGE('',*,*,#2376,.T.);
#3422=ORIENTED_EDGE('',*,*,#2379,.T.);
#3423=ORIENTED_EDGE('',*,*,#2383,.T.);
#3424=ORIENTED_EDGE('',*,*,#2388,.T.);
#3425=ORIENTED_EDGE('',*,*,#2387,.T.);
#3426=ORIENTED_EDGE('',*,*,#2290,.F.);
#3427=ORIENTED_EDGE('',*,*,#2406,.T.);
#3428=ORIENTED_EDGE('',*,*,#2345,.T.);
#3429=ORIENTED_EDGE('',*,*,#2405,.F.);
#3430=ORIENTED_EDGE('',*,*,#2404,.T.);
#3431=ORIENTED_EDGE('',*,*,#2293,.F.);
#3432=ORIENTED_EDGE('',*,*,#2407,.F.);
#3433=ORIENTED_EDGE('',*,*,#2408,.F.);
#3434=ORIENTED_EDGE('',*,*,#2385,.F.);
#3435=ORIENTED_EDGE('',*,*,#2384,.F.);
#3436=ORIENTED_EDGE('',*,*,#2381,.F.);
#3437=ORIENTED_EDGE('',*,*,#2380,.F.);
#3438=ORIENTED_EDGE('',*,*,#2377,.F.);
#3439=ORIENTED_EDGE('',*,*,#2374,.F.);
#3440=ORIENTED_EDGE('',*,*,#2371,.F.);
#3441=ORIENTED_EDGE('',*,*,#2368,.F.);
#3442=ORIENTED_EDGE('',*,*,#2365,.F.);
#3443=ORIENTED_EDGE('',*,*,#2362,.F.);
#3444=ORIENTED_EDGE('',*,*,#2359,.F.);
#3445=ORIENTED_EDGE('',*,*,#2356,.F.);
#3446=ORIENTED_EDGE('',*,*,#2353,.F.);
#3447=ORIENTED_EDGE('',*,*,#2349,.F.);
#3448=ORIENTED_EDGE('',*,*,#2346,.F.);
#3449=ORIENTED_EDGE('',*,*,#2406,.F.);
#3450=ORIENTED_EDGE('',*,*,#2289,.F.);
#3451=ORIENTED_EDGE('',*,*,#2288,.F.);
#3452=ORIENTED_EDGE('',*,*,#2287,.F.);
#3453=ORIENTED_EDGE('',*,*,#2298,.F.);
#3454=ORIENTED_EDGE('',*,*,#2301,.F.);
#3455=ORIENTED_EDGE('',*,*,#2305,.F.);
#3456=ORIENTED_EDGE('',*,*,#2304,.F.);
#3457=ORIENTED_EDGE('',*,*,#2310,.F.);
#3458=ORIENTED_EDGE('',*,*,#2309,.F.);
#3459=ORIENTED_EDGE('',*,*,#2314,.F.);
#3460=ORIENTED_EDGE('',*,*,#2318,.F.);
#3461=ORIENTED_EDGE('',*,*,#2317,.F.);
#3462=ORIENTED_EDGE('',*,*,#2322,.F.);
#3463=ORIENTED_EDGE('',*,*,#2325,.F.);
#3464=ORIENTED_EDGE('',*,*,#2329,.F.);
#3465=ORIENTED_EDGE('',*,*,#2328,.F.);
#3466=ORIENTED_EDGE('',*,*,#2334,.F.);
#3467=ORIENTED_EDGE('',*,*,#2333,.F.);
#3468=ORIENTED_EDGE('',*,*,#2338,.F.);
#3469=ORIENTED_EDGE('',*,*,#2341,.F.);
#3470=ORIENTED_EDGE('',*,*,#2393,.F.);
#3471=ORIENTED_EDGE('',*,*,#2403,.T.);
#3472=ORIENTED_EDGE('',*,*,#2386,.T.);
#3473=ORIENTED_EDGE('',*,*,#2408,.T.);
#3474=ORIENTED_EDGE('',*,*,#2407,.T.);
#3475=ORIENTED_EDGE('',*,*,#2392,.T.);
#3476=ORIENTED_EDGE('',*,*,#2409,.T.);
#3477=ORIENTED_EDGE('',*,*,#2410,.T.);
#3478=ORIENTED_EDGE('',*,*,#2411,.T.);
#3479=ORIENTED_EDGE('',*,*,#2410,.F.);
#3480=ORIENTED_EDGE('',*,*,#2411,.F.);
#3481=ORIENTED_EDGE('',*,*,#2412,.T.);
#3482=ORIENTED_EDGE('',*,*,#2413,.T.);
#3483=ORIENTED_EDGE('',*,*,#2412,.F.);
#3484=ORIENTED_EDGE('',*,*,#2409,.F.);
#3485=ORIENTED_EDGE('',*,*,#2292,.F.);
#3486=ORIENTED_EDGE('',*,*,#2414,.T.);
#3487=ORIENTED_EDGE('',*,*,#2415,.T.);
#3488=ORIENTED_EDGE('',*,*,#2416,.T.);
#3489=ORIENTED_EDGE('',*,*,#2415,.F.);
#3490=ORIENTED_EDGE('',*,*,#2416,.F.);
#3491=ORIENTED_EDGE('',*,*,#2417,.T.);
#3492=ORIENTED_EDGE('',*,*,#2418,.F.);
#3493=ORIENTED_EDGE('',*,*,#2417,.F.);
#3494=ORIENTED_EDGE('',*,*,#2414,.F.);
#3495=ORIENTED_EDGE('',*,*,#2413,.F.);
#3496=ORIENTED_EDGE('',*,*,#2418,.T.);
#3497=ORIENTED_EDGE('',*,*,#2419,.T.);
#3498=ORIENTED_EDGE('',*,*,#2420,.T.);
#3499=ORIENTED_EDGE('',*,*,#2419,.F.);
#3500=ORIENTED_EDGE('',*,*,#2420,.F.);
#3501=ORIENTED_EDGE('',*,*,#2421,.T.);
#3502=ORIENTED_EDGE('',*,*,#2422,.T.);
#3503=ORIENTED_EDGE('',*,*,#2423,.T.);
#3504=ORIENTED_EDGE('',*,*,#2424,.T.);
#3505=ORIENTED_EDGE('',*,*,#2423,.F.);
#3506=ORIENTED_EDGE('',*,*,#2424,.F.);
#3507=ORIENTED_EDGE('',*,*,#2425,.T.);
#3508=ORIENTED_EDGE('',*,*,#2426,.F.);
#3509=ORIENTED_EDGE('',*,*,#2425,.F.);
#3510=ORIENTED_EDGE('',*,*,#2422,.F.);
#3511=ORIENTED_EDGE('',*,*,#2427,.F.);
#3512=ORIENTED_EDGE('',*,*,#2426,.T.);
#3513=ORIENTED_EDGE('',*,*,#2428,.T.);
#3514=ORIENTED_EDGE('',*,*,#2402,.T.);
#3515=ORIENTED_EDGE('',*,*,#2428,.F.);
#3516=ORIENTED_EDGE('',*,*,#2395,.T.);
#3517=ORIENTED_EDGE('',*,*,#2429,.T.);
#3518=ORIENTED_EDGE('',*,*,#2430,.T.);
#3519=ORIENTED_EDGE('',*,*,#2429,.F.);
#3520=ORIENTED_EDGE('',*,*,#2430,.F.);
#3521=ORIENTED_EDGE('',*,*,#2431,.T.);
#3522=ORIENTED_EDGE('',*,*,#2432,.F.);
#3523=ORIENTED_EDGE('',*,*,#2431,.F.);
#3524=ORIENTED_EDGE('',*,*,#2432,.T.);
#3525=ORIENTED_EDGE('',*,*,#2433,.T.);
#3526=ORIENTED_EDGE('',*,*,#2434,.T.);
#3527=ORIENTED_EDGE('',*,*,#2433,.F.);
#3528=ORIENTED_EDGE('',*,*,#2434,.F.);
#3529=ORIENTED_EDGE('',*,*,#2435,.T.);
#3530=ORIENTED_EDGE('',*,*,#2436,.T.);
#3531=ORIENTED_EDGE('',*,*,#2437,.T.);
#3532=ORIENTED_EDGE('',*,*,#2438,.T.);
#3533=ORIENTED_EDGE('',*,*,#2437,.F.);
#3534=ORIENTED_EDGE('',*,*,#2438,.F.);
#3535=ORIENTED_EDGE('',*,*,#2439,.T.);
#3536=ORIENTED_EDGE('',*,*,#2440,.F.);
#3537=ORIENTED_EDGE('',*,*,#2439,.F.);
#3538=ORIENTED_EDGE('',*,*,#2436,.F.);
#3539=ORIENTED_EDGE('',*,*,#2441,.F.);
#3540=ORIENTED_EDGE('',*,*,#2440,.T.);
#3541=ORIENTED_EDGE('',*,*,#2442,.T.);
#3542=ORIENTED_EDGE('',*,*,#2443,.T.);
#3543=ORIENTED_EDGE('',*,*,#2442,.F.);
#3544=ORIENTED_EDGE('',*,*,#2443,.F.);
#3545=ORIENTED_EDGE('',*,*,#2444,.T.);
#3546=ORIENTED_EDGE('',*,*,#2445,.T.);
#3547=ORIENTED_EDGE('',*,*,#2446,.T.);
#3548=ORIENTED_EDGE('',*,*,#2447,.T.);
#3549=ORIENTED_EDGE('',*,*,#2446,.F.);
#3550=ORIENTED_EDGE('',*,*,#2447,.F.);
#3551=ORIENTED_EDGE('',*,*,#2444,.F.);
#3552=ORIENTED_EDGE('',*,*,#2448,.T.);
#3553=ORIENTED_EDGE('',*,*,#2445,.F.);
#3554=ORIENTED_EDGE('',*,*,#2448,.F.);
#3555=ORIENTED_EDGE('',*,*,#2435,.F.);
#3556=ORIENTED_EDGE('',*,*,#2449,.T.);
#3557=ORIENTED_EDGE('',*,*,#2441,.T.);
#3558=ORIENTED_EDGE('',*,*,#2449,.F.);
#3559=ORIENTED_EDGE('',*,*,#2421,.F.);
#3560=ORIENTED_EDGE('',*,*,#2450,.T.);
#3561=ORIENTED_EDGE('',*,*,#2427,.T.);
#3562=ORIENTED_EDGE('',*,*,#2450,.F.);
#3611=B_SPLINE_SURFACE_WITH_KNOTS('',3,3,((#26503,#26504,#26505,#26506,
#26507,#26508,#26509,#26510,#26511,#26512,#26513,#26514,#26515,#26516,#26517,
#26518,#26519,#26520,#26521,#26522,#26523,#26524,#26525,#26526,#26527,#26528,
#26529,#26530,#26531,#26532,#26533,#26534,#26535,#26536,#26537,#26538,#26539,
#26540,#26541,#26542,#26543,#26544,#26545,#26546,#26547,#26548,#26549,#26550,
#26551,#26552,#26553,#26554,#26555,#26556,#26557,#26558,#26559,#26560,#26561,
#26562,#26563,#26564,#26565,#26566,#26567,#26568,#26569,#26570,#26571,#26572,
#26573,#26574,#26575,#26576,#26577,#26578,#26579,#26580,#26581,#26582,#26583,
#26584,#26585,#26586,#26587,#26588,#26589,#26590,#26591),(#26592,#26593,
#26594,#26595,#26596,#26597,#26598,#26599,#26600,#26601,#26602,#26603,#26604,
#26605,#26606,#26607,#26608,#26609,#26610,#26611,#26612,#26613,#26614,#26615,
#26616,#26617,#26618,#26619,#26620,#26621,#26622,#26623,#26624,#26625,#26626,
#26627,#26628,#26629,#26630,#26631,#26632,#26633,#26634,#26635,#26636,#26637,
#26638,#26639,#26640,#26641,#26642,#26643,#26644,#26645,#26646,#26647,#26648,
#26649,#26650,#26651,#26652,#26653,#26654,#26655,#26656,#26657,#26658,#26659,
#26660,#26661,#26662,#26663,#26664,#26665,#26666,#26667,#26668,#26669,#26670,
#26671,#26672,#26673,#26674,#26675,#26676,#26677,#26678,#26679,#26680),
(#26681,#26682,#26683,#26684,#26685,#26686,#26687,#26688,#26689,#26690,
#26691,#26692,#26693,#26694,#26695,#26696,#26697,#26698,#26699,#26700,#26701,
#26702,#26703,#26704,#26705,#26706,#26707,#26708,#26709,#26710,#26711,#26712,
#26713,#26714,#26715,#26716,#26717,#26718,#26719,#26720,#26721,#26722,#26723,
#26724,#26725,#26726,#26727,#26728,#26729,#26730,#26731,#26732,#26733,#26734,
#26735,#26736,#26737,#26738,#26739,#26740,#26741,#26742,#26743,#26744,#26745,
#26746,#26747,#26748,#26749,#26750,#26751,#26752,#26753,#26754,#26755,#26756,
#26757,#26758,#26759,#26760,#26761,#26762,#26763,#26764,#26765,#26766,#26767,
#26768,#26769),(#26770,#26771,#26772,#26773,#26774,#26775,#26776,#26777,
#26778,#26779,#26780,#26781,#26782,#26783,#26784,#26785,#26786,#26787,#26788,
#26789,#26790,#26791,#26792,#26793,#26794,#26795,#26796,#26797,#26798,#26799,
#26800,#26801,#26802,#26803,#26804,#26805,#26806,#26807,#26808,#26809,#26810,
#26811,#26812,#26813,#26814,#26815,#26816,#26817,#26818,#26819,#26820,#26821,
#26822,#26823,#26824,#26825,#26826,#26827,#26828,#26829,#26830,#26831,#26832,
#26833,#26834,#26835,#26836,#26837,#26838,#26839,#26840,#26841,#26842,#26843,
#26844,#26845,#26846,#26847,#26848,#26849,#26850,#26851,#26852,#26853,#26854,
#26855,#26856,#26857,#26858)),.UNSPECIFIED.,.F.,.F.,.F.,(4,4),(4,1,1,1,
1,1,1,1,1,1,1,1,1,1,1,1,1,1,1,1,1,1,1,1,1,1,1,1,1,1,1,1,1,1,1,1,1,1,1,1,
1,1,1,1,1,1,1,1,1,1,1,1,1,1,1,1,1,1,1,1,1,1,1,1,1,1,1,1,1,1,1,1,1,1,1,1,
1,1,1,1,1,1,1,1,1,1,4),(-0.000803760615569271,0.050103355208433),(13.3936548749541,
14.3924503130856,15.3906450173941,16.3888397217026,17.3870344260111,18.3852291303196,
19.3834238346281,20.3816185389366,21.3798132432451,22.3780079475536,23.3762026518621,
24.3743973561706,25.3725920604791,26.3707867647876,27.3689814690961,28.3671761734046,
29.365370877713,30.3635655820215,31.36176028633,32.3599549906385,33.358149694947,
34.3563443992555,35.354539103564,36.3527338078725,37.350928512181,38.3491232164895,
39.347317920798,40.3455126251065,41.343707329415,42.3419020337235,43.340096738032,
44.3382914423405,45.336486146649,46.3346808509575,47.332875555266,48.3310702595745,
49.329264963883,50.3274596681915,51.3256543725,52.3238490768085,53.322043781117,
54.3202384854255,55.318433189734,56.3166278940425,57.314822598351,58.3130173026595,
59.311212006968,60.3094067112765,61.307601415585,62.3057961198935,63.303990824202,
64.3021855285105,65.300380232819,66.2985749371275,67.296769641436,68.2949643457444,
69.2931590500529,70.2913537543614,71.2895484586699,72.2877431629784,73.2859378672869,
74.2841325715954,75.2823272759039,76.2805219802124,77.2787166845209,78.2769113888294,
79.2751060931379,80.2733007974464,81.2714955017549,82.2696902060634,83.2678849103719,
84.2660796146804,85.2642743189889,86.2624690232974,87.2606637276059,88.2588584319144,
89.2570531362229,90.2552478405314,91.2534425448399,92.2516372491484,93.2498319534569,
94.2480266577654,95.2462213620739,96.2444160663824,97.2426107706909,98.2408054749994,
99.2393733588525),.UNSPECIFIED.);
#3612=B_SPLINE_SURFACE_WITH_KNOTS('',3,3,((#27117,#27118,#27119,#27120,
#27121,#27122,#27123,#27124,#27125,#27126,#27127,#27128,#27129,#27130,#27131,
#27132,#27133,#27134,#27135,#27136,#27137,#27138,#27139,#27140,#27141,#27142,
#27143,#27144,#27145,#27146,#27147,#27148,#27149,#27150,#27151,#27152,#27153,
#27154,#27155,#27156,#27157,#27158,#27159,#27160,#27161,#27162,#27163,#27164,
#27165,#27166,#27167,#27168,#27169,#27170,#27171,#27172,#27173,#27174,#27175,
#27176,#27177,#27178,#27179,#27180,#27181,#27182,#27183,#27184,#27185,#27186,
#27187,#27188,#27189,#27190,#27191,#27192,#27193,#27194,#27195,#27196,#27197,
#27198,#27199,#27200,#27201,#27202,#27203,#27204,#27205),(#27206,#27207,
#27208,#27209,#27210,#27211,#27212,#27213,#27214,#27215,#27216,#27217,#27218,
#27219,#27220,#27221,#27222,#27223,#27224,#27225,#27226,#27227,#27228,#27229,
#27230,#27231,#27232,#27233,#27234,#27235,#27236,#27237,#27238,#27239,#27240,
#27241,#27242,#27243,#27244,#27245,#27246,#27247,#27248,#27249,#27250,#27251,
#27252,#27253,#27254,#27255,#27256,#27257,#27258,#27259,#27260,#27261,#27262,
#27263,#27264,#27265,#27266,#27267,#27268,#27269,#27270,#27271,#27272,#27273,
#27274,#27275,#27276,#27277,#27278,#27279,#27280,#27281,#27282,#27283,#27284,
#27285,#27286,#27287,#27288,#27289,#27290,#27291,#27292,#27293,#27294),
(#27295,#27296,#27297,#27298,#27299,#27300,#27301,#27302,#27303,#27304,
#27305,#27306,#27307,#27308,#27309,#27310,#27311,#27312,#27313,#27314,#27315,
#27316,#27317,#27318,#27319,#27320,#27321,#27322,#27323,#27324,#27325,#27326,
#27327,#27328,#27329,#27330,#27331,#27332,#27333,#27334,#27335,#27336,#27337,
#27338,#27339,#27340,#27341,#27342,#27343,#27344,#27345,#27346,#27347,#27348,
#27349,#27350,#27351,#27352,#27353,#27354,#27355,#27356,#27357,#27358,#27359,
#27360,#27361,#27362,#27363,#27364,#27365,#27366,#27367,#27368,#27369,#27370,
#27371,#27372,#27373,#27374,#27375,#27376,#27377,#27378,#27379,#27380,#27381,
#27382,#27383),(#27384,#27385,#27386,#27387,#27388,#27389,#27390,#27391,
#27392,#27393,#27394,#27395,#27396,#27397,#27398,#27399,#27400,#27401,#27402,
#27403,#27404,#27405,#27406,#27407,#27408,#27409,#27410,#27411,#27412,#27413,
#27414,#27415,#27416,#27417,#27418,#27419,#27420,#27421,#27422,#27423,#27424,
#27425,#27426,#27427,#27428,#27429,#27430,#27431,#27432,#27433,#27434,#27435,
#27436,#27437,#27438,#27439,#27440,#27441,#27442,#27443,#27444,#27445,#27446,
#27447,#27448,#27449,#27450,#27451,#27452,#27453,#27454,#27455,#27456,#27457,
#27458,#27459,#27460,#27461,#27462,#27463,#27464,#27465,#27466,#27467,#27468,
#27469,#27470,#27471,#27472)),.UNSPECIFIED.,.F.,.F.,.F.,(4,4),(4,1,1,1,
1,1,1,1,1,1,1,1,1,1,1,1,1,1,1,1,1,1,1,1,1,1,1,1,1,1,1,1,1,1,1,1,1,1,1,1,
1,1,1,1,1,1,1,1,1,1,1,1,1,1,1,1,1,1,1,1,1,1,1,1,1,1,1,1,1,1,1,1,1,1,1,1,
1,1,1,1,1,1,1,1,1,1,4),(-0.000630172471168558,0.0497654761150975),(16.7016191235447,
17.7001869884391,18.6983816927476,19.6965763970561,20.6947711013646,21.6929658056731,
22.6911605099816,23.6893552142901,24.6875499185986,25.6857446229071,26.6839393272156,
27.6821340315241,28.6803287358326,29.6785234401411,30.6767181444496,31.6749128487581,
32.6731075530666,33.6713022573751,34.6694969616836,35.6676916659921,36.6658863703006,
37.6640810746091,38.6622757789176,39.6604704832261,40.6586651875346,41.6568598918431,
42.6550545961516,43.65324930046,44.6514440047685,45.6496387090771,46.6478334133855,
47.646028117694,48.6442228220025,49.642417526311,50.6406122306195,51.638806934928,
52.6370016392365,53.635196343545,54.6333910478535,55.631585752162,56.6297804564705,
57.627975160779,58.6261698650875,59.624364569396,60.6225592737045,61.620753978013,
62.6189486823215,63.61714338663,64.6153380909385,65.613532795247,66.6117274995555,
67.609922203864,68.6081169081725,69.606311612481,70.6045063167895,71.602701021098,
72.6008957254065,73.599090429715,74.5972851340235,75.595479838332,76.5936745426405,
77.591869246949,78.5900639512575,79.588258655566,80.5864533598745,81.584648064183,
82.5828427684915,83.5810374728,84.5792321771085,85.577426881417,86.5756215857255,
87.573816290034,88.5720109943425,89.570205698651,90.5684004029595,91.566595107268,
92.5647898115765,93.562984515885,94.5611792201935,95.559373924502,96.5575686288105,
97.555763333119,98.5539580374275,99.552152741736,100.550347446044,101.548542150353,
102.547367027132),.UNSPECIFIED.);
#3765=ADVANCED_FACE('',(#590,#151),#403,.T.);
#3766=ADVANCED_FACE('',(#591),#404,.T.);
#3767=ADVANCED_FACE('',(#592),#405,.T.);
#3768=ADVANCED_FACE('',(#593),#406,.T.);
#3769=ADVANCED_FACE('',(#594),#407,.T.);
#3770=ADVANCED_FACE('',(#595),#408,.T.);
#3771=ADVANCED_FACE('',(#596),#409,.T.);
#3772=ADVANCED_FACE('',(#597),#410,.T.);
#3773=ADVANCED_FACE('',(#598),#411,.T.);
#3774=ADVANCED_FACE('',(#599),#412,.T.);
#3775=ADVANCED_FACE('',(#600),#413,.T.);
#3776=ADVANCED_FACE('',(#601),#414,.T.);
#3777=ADVANCED_FACE('',(#602),#415,.T.);
#3778=ADVANCED_FACE('',(#603),#416,.T.);
#3779=ADVANCED_FACE('',(#604),#417,.T.);
#3780=ADVANCED_FACE('',(#605),#418,.T.);
#3781=ADVANCED_FACE('',(#606),#419,.T.);
#3782=ADVANCED_FACE('',(#607),#420,.T.);
#3783=ADVANCED_FACE('',(#608),#421,.T.);
#3784=ADVANCED_FACE('',(#609),#422,.T.);
#3785=ADVANCED_FACE('',(#610),#423,.T.);
#3786=ADVANCED_FACE('',(#611),#424,.T.);
#3787=ADVANCED_FACE('',(#612),#425,.T.);
#3788=ADVANCED_FACE('',(#613),#426,.T.);
#3789=ADVANCED_FACE('',(#614),#427,.T.);
#3790=ADVANCED_FACE('',(#615),#428,.T.);
#3791=ADVANCED_FACE('',(#616),#429,.T.);
#3792=ADVANCED_FACE('',(#617),#430,.F.);
#3793=ADVANCED_FACE('',(#618),#203,.T.);
#3794=ADVANCED_FACE('',(#619),#431,.T.);
#3795=ADVANCED_FACE('',(#620,#152),#204,.T.);
#3796=ADVANCED_FACE('',(#621),#55,.T.);
#3797=ADVANCED_FACE('',(#622),#83,.T.);
#3798=ADVANCED_FACE('',(#623),#56,.T.);
#3799=ADVANCED_FACE('',(#624,#153),#205,.T.);
#3800=ADVANCED_FACE('',(#625),#3611,.F.);
#3801=ADVANCED_FACE('',(#626),#206,.T.);
#3802=ADVANCED_FACE('',(#627),#3612,.F.);
#3803=ADVANCED_FACE('',(#628),#207,.T.);
#3804=ADVANCED_FACE('',(#629),#57,.T.);
#3805=ADVANCED_FACE('',(#630),#432,.T.);
#3806=ADVANCED_FACE('',(#631,#154),#208,.T.);
#3807=ADVANCED_FACE('',(#632),#58,.T.);
#3808=ADVANCED_FACE('',(#633),#84,.T.);
#3809=ADVANCED_FACE('',(#634,#155),#209,.T.);
#3810=ADVANCED_FACE('',(#635),#59,.T.);
#3811=ADVANCED_FACE('',(#636,#156),#210,.T.);
#3812=ADVANCED_FACE('',(#637),#60,.T.);
#3813=ADVANCED_FACE('',(#638),#85,.T.);
#3814=ADVANCED_FACE('',(#639,#157),#211,.T.);
#3815=ADVANCED_FACE('',(#640),#61,.T.);
#3816=ADVANCED_FACE('',(#641),#62,.T.);
#3817=ADVANCED_FACE('',(#642),#86,.T.);
#3818=ADVANCED_FACE('',(#643),#63,.T.);
#3819=ADVANCED_FACE('',(#644,#158),#212,.T.);
#3820=ADVANCED_FACE('',(#645),#64,.T.);
#3821=ADVANCED_FACE('',(#646),#87,.T.);
#3822=ADVANCED_FACE('',(#647,#159),#213,.T.);
#3823=ADVANCED_FACE('',(#648),#65,.T.);
#3824=ADVANCED_FACE('',(#649,#160),#214,.T.);
#3825=ADVANCED_FACE('',(#650),#66,.T.);
#3826=ADVANCED_FACE('',(#651),#215,.T.);
#3827=ADVANCED_FACE('',(#652),#433,.T.);
#3828=ADVANCED_FACE('',(#653),#434,.T.);
#3829=ADVANCED_FACE('',(#654),#435,.T.);
#3842=CLOSED_SHELL('',(#3765,#3766,#3767,#3768,#3769,#3770,#3771,#3772,
#3773,#3774,#3775,#3776,#3777,#3778,#3779,#3780,#3781,#3782,#3783,#3784,
#3785,#3786,#3787,#3788,#3789,#3790,#3791,#3792,#3793,#3794,#3795,#3796,
#3797,#3798,#3799,#3800,#3801,#3802,#3803,#3804,#3805,#3806,#3807,#3808,
#3809,#3810,#3811,#3812,#3813,#3814,#3815,#3816,#3817,#3818,#3819,#3820,
#3821,#3822,#3823,#3824,#3825,#3826,#3827,#3828,#3829));
#4156=AXIS2_PLACEMENT_3D('',#15718,#4827,#4828);
#4157=AXIS2_PLACEMENT_3D('',#15719,#4829,#4830);
#4158=AXIS2_PLACEMENT_3D('',#15861,#4832,#4833);
#4159=AXIS2_PLACEMENT_3D('',#15864,#4835,#4836);
#4160=AXIS2_PLACEMENT_3D('',#15866,#4837,#4838);
#4161=AXIS2_PLACEMENT_3D('',#15975,#4839,#4840);
#4162=AXIS2_PLACEMENT_3D('',#16399,#4842,#4843);
#4163=AXIS2_PLACEMENT_3D('',#16799,#4845,#4846);
#4164=AXIS2_PLACEMENT_3D('',#17233,#4848,#4849);
#4165=AXIS2_PLACEMENT_3D('',#17645,#4851,#4852);
#4166=AXIS2_PLACEMENT_3D('',#18049,#4854,#4855);
#4167=AXIS2_PLACEMENT_3D('',#18467,#4857,#4858);
#4168=AXIS2_PLACEMENT_3D('',#18869,#4860,#4861);
#4169=AXIS2_PLACEMENT_3D('',#19293,#4863,#4864);
#4170=AXIS2_PLACEMENT_3D('',#19717,#4866,#4867);
#4171=AXIS2_PLACEMENT_3D('',#20143,#4869,#4870);
#4172=AXIS2_PLACEMENT_3D('',#20551,#4872,#4873);
#4173=AXIS2_PLACEMENT_3D('',#20957,#4875,#4876);
#4174=AXIS2_PLACEMENT_3D('',#21113,#4878,#4879);
#4175=AXIS2_PLACEMENT_3D('',#21256,#4880,#4881);
#4176=AXIS2_PLACEMENT_3D('',#21632,#4883,#4884);
#4177=AXIS2_PLACEMENT_3D('',#22033,#4886,#4887);
#4178=AXIS2_PLACEMENT_3D('',#22415,#4889,#4890);
#4179=AXIS2_PLACEMENT_3D('',#22801,#4892,#4893);
#4180=AXIS2_PLACEMENT_3D('',#23193,#4895,#4896);
#4181=AXIS2_PLACEMENT_3D('',#23575,#4898,#4899);
#4182=AXIS2_PLACEMENT_3D('',#23965,#4901,#4902);
#4183=AXIS2_PLACEMENT_3D('',#24343,#4904,#4905);
#4184=AXIS2_PLACEMENT_3D('',#24729,#4907,#4908);
#4185=AXIS2_PLACEMENT_3D('',#25113,#4910,#4911);
#4186=AXIS2_PLACEMENT_3D('',#25504,#4913,#4914);
#4187=AXIS2_PLACEMENT_3D('',#25892,#4916,#4917);
#4188=AXIS2_PLACEMENT_3D('',#26031,#4918,#4919);
#4189=AXIS2_PLACEMENT_3D('',#26139,#4920,#4921);
#4190=AXIS2_PLACEMENT_3D('',#26141,#4922,#4923);
#4191=AXIS2_PLACEMENT_3D('',#26143,#4925,#4926);
#4192=AXIS2_PLACEMENT_3D('',#26144,#4927,#4928);
#4193=AXIS2_PLACEMENT_3D('',#26328,#4929,#4930);
#4194=AXIS2_PLACEMENT_3D('',#26483,#4931,#4932);
#4195=AXIS2_PLACEMENT_3D('',#26485,#4933,#4934);
#4196=AXIS2_PLACEMENT_3D('',#26487,#4935,#4936);
#4197=AXIS2_PLACEMENT_3D('',#26488,#4937,#4938);
#4198=AXIS2_PLACEMENT_3D('',#26490,#4939,#4940);
#4199=AXIS2_PLACEMENT_3D('',#26492,#4941,#4942);
#4200=AXIS2_PLACEMENT_3D('',#26493,#4943,#4944);
#4201=AXIS2_PLACEMENT_3D('',#26494,#4945,#4946);
#4202=AXIS2_PLACEMENT_3D('',#26497,#4948,#4949);
#4203=AXIS2_PLACEMENT_3D('',#26498,#4950,#4951);
#4204=AXIS2_PLACEMENT_3D('',#26499,#4952,#4953);
#4205=AXIS2_PLACEMENT_3D('',#26500,#4954,#4955);
#4206=AXIS2_PLACEMENT_3D('',#26502,#4956,#4957);
#4207=AXIS2_PLACEMENT_3D('',#27028,#4958,#4959);
#4208=AXIS2_PLACEMENT_3D('',#27566,#4960,#4961);
#4209=AXIS2_PLACEMENT_3D('',#27567,#4962,#4963);
#4210=AXIS2_PLACEMENT_3D('',#27569,#4964,#4965);
#4211=AXIS2_PLACEMENT_3D('',#27571,#4966,#4967);
#4212=AXIS2_PLACEMENT_3D('',#27572,#4968,#4969);
#4213=AXIS2_PLACEMENT_3D('',#27573,#4970,#4971);
#4214=AXIS2_PLACEMENT_3D('',#27576,#4973,#4974);
#4215=AXIS2_PLACEMENT_3D('',#27577,#4975,#4976);
#4216=AXIS2_PLACEMENT_3D('',#27578,#4977,#4978);
#4217=AXIS2_PLACEMENT_3D('',#27580,#4979,#4980);
#4218=AXIS2_PLACEMENT_3D('',#27582,#4981,#4982);
#4219=AXIS2_PLACEMENT_3D('',#27583,#4983,#4984);
#4220=AXIS2_PLACEMENT_3D('',#27584,#4985,#4986);
#4221=AXIS2_PLACEMENT_3D('',#27587,#4988,#4989);
#4222=AXIS2_PLACEMENT_3D('',#27588,#4990,#4991);
#4223=AXIS2_PLACEMENT_3D('',#27589,#4992,#4993);
#4224=AXIS2_PLACEMENT_3D('',#27591,#4994,#4995);
#4225=AXIS2_PLACEMENT_3D('',#27592,#4996,#4997);
#4226=AXIS2_PLACEMENT_3D('',#27593,#4998,#4999);
#4227=AXIS2_PLACEMENT_3D('',#27595,#5000,#5001);
#4228=AXIS2_PLACEMENT_3D('',#27596,#5002,#5003);
#4229=AXIS2_PLACEMENT_3D('',#27598,#5004,#5005);
#4230=AXIS2_PLACEMENT_3D('',#27600,#5006,#5007);
#4231=AXIS2_PLACEMENT_3D('',#27601,#5008,#5009);
#4232=AXIS2_PLACEMENT_3D('',#27602,#5010,#5011);
#4233=AXIS2_PLACEMENT_3D('',#27605,#5013,#5014);
#4234=AXIS2_PLACEMENT_3D('',#27606,#5015,#5016);
#4235=AXIS2_PLACEMENT_3D('',#27608,#5017,#5018);
#4236=AXIS2_PLACEMENT_3D('',#27609,#5019,#5020);
#4237=AXIS2_PLACEMENT_3D('',#27610,#5021,#5022);
#4238=AXIS2_PLACEMENT_3D('',#27611,#5023,#5024);
#4239=AXIS2_PLACEMENT_3D('',#27613,#5025,#5026);
#4240=AXIS2_PLACEMENT_3D('',#27614,#5027,#5028);
#4241=AXIS2_PLACEMENT_3D('',#27615,#5029,#5030);
#4242=AXIS2_PLACEMENT_3D('',#27618,#5032,#5033);
#4243=AXIS2_PLACEMENT_3D('',#27619,#5034,#5035);
#4244=AXIS2_PLACEMENT_3D('',#27621,#5036,#5037);
#4245=AXIS2_PLACEMENT_3D('',#27622,#5038,#5039);
#4246=AXIS2_PLACEMENT_3D('',#27623,#5040,#5041);
#4247=AXIS2_PLACEMENT_3D('',#27625,#5042,#5043);
#4248=AXIS2_PLACEMENT_3D('',#27626,#5044,#5045);
#4249=AXIS2_PLACEMENT_3D('',#27628,#5046,#5047);
#4250=AXIS2_PLACEMENT_3D('',#27630,#5048,#5049);
#4251=AXIS2_PLACEMENT_3D('',#27631,#5050,#5051);
#4252=AXIS2_PLACEMENT_3D('',#27632,#5052,#5053);
#4253=AXIS2_PLACEMENT_3D('',#27635,#5055,#5056);
#4254=AXIS2_PLACEMENT_3D('',#27636,#5057,#5058);
#4255=AXIS2_PLACEMENT_3D('',#27638,#5059,#5060);
#4256=AXIS2_PLACEMENT_3D('',#27639,#5061,#5062);
#4257=AXIS2_PLACEMENT_3D('',#27641,#5063,#5064);
#4258=AXIS2_PLACEMENT_3D('',#27642,#5065,#5066);
#4259=AXIS2_PLACEMENT_3D('',#27643,#5067,#5068);
#4260=AXIS2_PLACEMENT_3D('',#27645,#5069,#5070);
#4261=AXIS2_PLACEMENT_3D('',#27646,#5071,#5072);
#4262=AXIS2_PLACEMENT_3D('',#27648,#5073,#5074);
#4263=AXIS2_PLACEMENT_3D('',#27650,#5075,#5076);
#4264=AXIS2_PLACEMENT_3D('',#27651,#5077,#5078);
#4265=AXIS2_PLACEMENT_3D('',#27652,#5079,#5080);
#4266=AXIS2_PLACEMENT_3D('',#27653,#5081,#5082);
#4267=AXIS2_PLACEMENT_3D('',#27655,#5084,#5085);
#4268=AXIS2_PLACEMENT_3D('',#27657,#5087,#5088);
#4827=DIRECTION('axis',(0.,0.,1.));
#4828=DIRECTION('refdir',(1.,0.,0.));
#4829=DIRECTION('center_axis',(1.,0.,0.));
#4830=DIRECTION('ref_axis',(0.,0.,-1.));
#4831=DIRECTION('',(-1.,0.,0.));
#4832=DIRECTION('center_axis',(-1.,0.,0.));
#4833=DIRECTION('ref_axis',(0.,0.,-1.));
#4834=DIRECTION('',(-1.,0.,0.));
#4835=DIRECTION('center_axis',(-1.,0.,0.));
#4836=DIRECTION('ref_axis',(0.,0.,-1.));
#4837=DIRECTION('center_axis',(-1.,0.,0.));
#4838=DIRECTION('ref_axis',(0.,0.,-1.));
#4839=DIRECTION('center_axis',(1.,0.,0.));
#4840=DIRECTION('ref_axis',(0.,0.,-1.));
#4841=DIRECTION('',(-1.,0.,0.));
#4842=DIRECTION('center_axis',(1.,0.,0.));
#4843=DIRECTION('ref_axis',(0.,0.,-1.));
#4844=DIRECTION('',(-1.,0.,0.));
#4845=DIRECTION('center_axis',(1.,0.,0.));
#4846=DIRECTION('ref_axis',(0.,0.,-1.));
#4847=DIRECTION('',(-1.,0.,0.));
#4848=DIRECTION('center_axis',(1.,0.,0.));
#4849=DIRECTION('ref_axis',(0.,0.,-1.));
#4850=DIRECTION('',(-1.,0.,0.));
#4851=DIRECTION('center_axis',(1.,0.,0.));
#4852=DIRECTION('ref_axis',(0.,0.,-1.));
#4853=DIRECTION('',(-1.,0.,0.));
#4854=DIRECTION('center_axis',(1.,0.,0.));
#4855=DIRECTION('ref_axis',(0.,0.,-1.));
#4856=DIRECTION('',(-1.,0.,0.));
#4857=DIRECTION('center_axis',(1.,0.,0.));
#4858=DIRECTION('ref_axis',(0.,0.,-1.));
#4859=DIRECTION('',(-1.,0.,0.));
#4860=DIRECTION('center_axis',(1.,0.,0.));
#4861=DIRECTION('ref_axis',(0.,0.,-1.));
#4862=DIRECTION('',(-1.,0.,0.));
#4863=DIRECTION('center_axis',(1.,0.,0.));
#4864=DIRECTION('ref_axis',(0.,0.,-1.));
#4865=DIRECTION('',(-1.,0.,0.));
#4866=DIRECTION('center_axis',(1.,0.,0.));
#4867=DIRECTION('ref_axis',(0.,0.,-1.));
#4868=DIRECTION('',(-1.,0.,0.));
#4869=DIRECTION('center_axis',(1.,0.,0.));
#4870=DIRECTION('ref_axis',(0.,0.,-1.));
#4871=DIRECTION('',(-1.,0.,0.));
#4872=DIRECTION('center_axis',(1.,0.,0.));
#4873=DIRECTION('ref_axis',(0.,0.,-1.));
#4874=DIRECTION('',(-1.,0.,0.));
#4875=DIRECTION('center_axis',(1.,0.,0.));
#4876=DIRECTION('ref_axis',(0.,-0.999641738703431,0.0267655420640338));
#4877=DIRECTION('',(-1.,0.,0.));
#4878=DIRECTION('center_axis',(-1.,0.,0.));
#4879=DIRECTION('ref_axis',(0.,9.28774802075533E-14,-1.));
#4880=DIRECTION('center_axis',(1.,0.,0.));
#4881=DIRECTION('ref_axis',(0.,-0.999641738703431,0.0267655420640338));
#4882=DIRECTION('',(-1.,0.,0.));
#4883=DIRECTION('center_axis',(1.,0.,0.));
#4884=DIRECTION('ref_axis',(0.,-0.999641738703431,0.0267655420640338));
#4885=DIRECTION('',(-1.,0.,0.));
#4886=DIRECTION('center_axis',(1.,0.,0.));
#4887=DIRECTION('ref_axis',(0.,-0.999641738703431,0.0267655420640338));
#4888=DIRECTION('',(-1.,0.,0.));
#4889=DIRECTION('center_axis',(1.,0.,0.));
#4890=DIRECTION('ref_axis',(0.,-0.999641738703431,0.0267655420640338));
#4891=DIRECTION('',(-1.,0.,0.));
#4892=DIRECTION('center_axis',(1.,0.,0.));
#4893=DIRECTION('ref_axis',(0.,-0.999641738703431,0.0267655420640338));
#4894=DIRECTION('',(-1.,0.,0.));
#4895=DIRECTION('center_axis',(1.,0.,0.));
#4896=DIRECTION('ref_axis',(0.,-0.999641738703431,0.0267655420640338));
#4897=DIRECTION('',(-1.,0.,0.));
#4898=DIRECTION('center_axis',(1.,0.,0.));
#4899=DIRECTION('ref_axis',(0.,-0.999641738703431,0.0267655420640338));
#4900=DIRECTION('',(-1.,0.,0.));
#4901=DIRECTION('center_axis',(1.,0.,0.));
#4902=DIRECTION('ref_axis',(0.,-0.999641738703431,0.0267655420640338));
#4903=DIRECTION('',(-1.,0.,0.));
#4904=DIRECTION('center_axis',(1.,0.,0.));
#4905=DIRECTION('ref_axis',(0.,-0.999641738703431,0.0267655420640338));
#4906=DIRECTION('',(-1.,0.,0.));
#4907=DIRECTION('center_axis',(1.,0.,0.));
#4908=DIRECTION('ref_axis',(0.,-0.999641738703431,0.0267655420640338));
#4909=DIRECTION('',(-1.,0.,0.));
#4910=DIRECTION('center_axis',(1.,0.,0.));
#4911=DIRECTION('ref_axis',(0.,-0.999641738703431,0.0267655420640338));
#4912=DIRECTION('',(-1.,0.,0.));
#4913=DIRECTION('center_axis',(1.,0.,0.));
#4914=DIRECTION('ref_axis',(0.,-0.999641738703431,0.0267655420640338));
#4915=DIRECTION('',(-1.,0.,0.));
#4916=DIRECTION('center_axis',(1.,0.,0.));
#4917=DIRECTION('ref_axis',(0.,-0.999641738703431,0.0267655420640338));
#4918=DIRECTION('center_axis',(1.,0.,0.));
#4919=DIRECTION('ref_axis',(0.,9.28774802075533E-14,-1.));
#4920=DIRECTION('center_axis',(0.,1.,0.));
#4921=DIRECTION('ref_axis',(1.,0.,0.));
#4922=DIRECTION('center_axis',(0.,1.,0.));
#4923=DIRECTION('ref_axis',(1.,0.,0.));
#4924=DIRECTION('',(0.,1.,0.));
#4925=DIRECTION('center_axis',(0.,1.,0.));
#4926=DIRECTION('ref_axis',(1.,0.,0.));
#4927=DIRECTION('center_axis',(1.,0.,0.));
#4928=DIRECTION('ref_axis',(0.,0.,-1.));
#4929=DIRECTION('center_axis',(-1.,0.,0.));
#4930=DIRECTION('ref_axis',(0.,0.,-1.));
#4931=DIRECTION('center_axis',(-1.,0.,0.));
#4932=DIRECTION('ref_axis',(0.,0.,1.));
#4933=DIRECTION('center_axis',(1.,0.,0.));
#4934=DIRECTION('ref_axis',(0.,1.22464679914735E-16,1.));
#4935=DIRECTION('center_axis',(-1.,0.,0.));
#4936=DIRECTION('ref_axis',(0.,1.22464679914735E-16,1.));
#4937=DIRECTION('center_axis',(1.,0.,0.));
#4938=DIRECTION('ref_axis',(0.,0.,-1.));
#4939=DIRECTION('center_axis',(-1.,0.,0.));
#4940=DIRECTION('ref_axis',(0.,0.,-1.));
#4941=DIRECTION('center_axis',(0.,-1.,-1.22464679914735E-16));
#4942=DIRECTION('ref_axis',(0.,-1.22464679914735E-16,1.));
#4943=DIRECTION('center_axis',(1.,0.,0.));
#4944=DIRECTION('ref_axis',(0.,0.,1.));
#4945=DIRECTION('center_axis',(1.,0.,0.));
#4946=DIRECTION('ref_axis',(0.,0.,-1.));
#4947=DIRECTION('',(-0.999999956307574,3.62016965809699E-20,-0.000295609285927787));
#4948=DIRECTION('center_axis',(-1.,0.,0.));
#4949=DIRECTION('ref_axis',(0.,0.,1.));
#4950=DIRECTION('center_axis',(1.,0.,0.));
#4951=DIRECTION('ref_axis',(0.,0.,-1.));
#4952=DIRECTION('center_axis',(0.,-1.,-1.22464679914735E-16));
#4953=DIRECTION('ref_axis',(0.,-1.22464679914735E-16,1.));
#4954=DIRECTION('center_axis',(-1.,0.,0.));
#4955=DIRECTION('ref_axis',(0.,0.,1.));
#4956=DIRECTION('center_axis',(1.,0.,0.));
#4957=DIRECTION('ref_axis',(0.,1.22464679914735E-16,1.));
#4958=DIRECTION('center_axis',(1.,0.,0.));
#4959=DIRECTION('ref_axis',(0.,0.,-1.));
#4960=DIRECTION('center_axis',(1.,0.,0.));
#4961=DIRECTION('ref_axis',(0.,0.,-1.));
#4962=DIRECTION('center_axis',(1.,0.,0.));
#4963=DIRECTION('ref_axis',(0.,0.,-1.));
#4964=DIRECTION('center_axis',(-1.,0.,0.));
#4965=DIRECTION('ref_axis',(0.,1.22464679914735E-16,1.));
#4966=DIRECTION('center_axis',(0.,-1.,-1.22464679914735E-16));
#4967=DIRECTION('ref_axis',(0.,-1.22464679914735E-16,1.));
#4968=DIRECTION('center_axis',(1.,0.,0.));
#4969=DIRECTION('ref_axis',(0.,1.22464679914735E-16,1.));
#4970=DIRECTION('center_axis',(1.,0.,0.));
#4971=DIRECTION('ref_axis',(0.,0.,-1.));
#4972=DIRECTION('',(-1.,0.,0.));
#4973=DIRECTION('center_axis',(1.,0.,0.));
#4974=DIRECTION('ref_axis',(0.,0.,-1.));
#4975=DIRECTION('center_axis',(1.,0.,0.));
#4976=DIRECTION('ref_axis',(0.,0.,-1.));
#4977=DIRECTION('center_axis',(1.,0.,0.));
#4978=DIRECTION('ref_axis',(0.,0.,-1.));
#4979=DIRECTION('center_axis',(-1.,0.,0.));
#4980=DIRECTION('ref_axis',(0.,1.22464679914735E-16,1.));
#4981=DIRECTION('center_axis',(0.,-1.,-1.22464679914735E-16));
#4982=DIRECTION('ref_axis',(0.,-1.22464679914735E-16,1.));
#4983=DIRECTION('center_axis',(1.,0.,0.));
#4984=DIRECTION('ref_axis',(0.,0.,1.));
#4985=DIRECTION('center_axis',(1.,0.,0.));
#4986=DIRECTION('ref_axis',(0.,0.,-1.));
#4987=DIRECTION('',(-0.999999956307574,3.62016965808668E-20,-0.000295609285926945));
#4988=DIRECTION('center_axis',(-1.,0.,0.));
#4989=DIRECTION('ref_axis',(0.,0.,1.));
#4990=DIRECTION('center_axis',(1.,0.,0.));
#4991=DIRECTION('ref_axis',(0.,0.,-1.));
#4992=DIRECTION('center_axis',(1.,0.,0.));
#4993=DIRECTION('ref_axis',(0.,0.,-1.));
#4994=DIRECTION('center_axis',(0.,-1.,-1.22464679914735E-16));
#4995=DIRECTION('ref_axis',(0.,-1.22464679914735E-16,1.));
#4996=DIRECTION('center_axis',(1.,0.,0.));
#4997=DIRECTION('ref_axis',(0.,1.22464679914735E-16,1.));
#4998=DIRECTION('center_axis',(-1.,0.,0.));
#4999=DIRECTION('ref_axis',(0.,0.,1.));
#5000=DIRECTION('center_axis',(1.,0.,0.));
#5001=DIRECTION('ref_axis',(0.,0.,-1.));
#5002=DIRECTION('center_axis',(1.,0.,0.));
#5003=DIRECTION('ref_axis',(0.,0.,-1.));
#5004=DIRECTION('center_axis',(-1.,0.,0.));
#5005=DIRECTION('ref_axis',(0.,1.22464679914735E-16,1.));
#5006=DIRECTION('center_axis',(0.,-1.,-1.22464679914735E-16));
#5007=DIRECTION('ref_axis',(0.,-1.22464679914735E-16,1.));
#5008=DIRECTION('center_axis',(1.,0.,0.));
#5009=DIRECTION('ref_axis',(0.,0.,1.));
#5010=DIRECTION('center_axis',(1.,0.,0.));
#5011=DIRECTION('ref_axis',(0.,0.,-1.));
#5012=DIRECTION('',(-0.999999956307574,3.62016965808707E-20,-0.000295609285926977));
#5013=DIRECTION('center_axis',(-1.,0.,0.));
#5014=DIRECTION('ref_axis',(0.,0.,1.));
#5015=DIRECTION('center_axis',(1.,0.,0.));
#5016=DIRECTION('ref_axis',(0.,0.,-1.));
#5017=DIRECTION('center_axis',(1.,0.,0.));
#5018=DIRECTION('ref_axis',(0.,0.,-1.));
#5019=DIRECTION('center_axis',(1.,0.,0.));
#5020=DIRECTION('ref_axis',(0.,0.,-1.));
#5021=DIRECTION('center_axis',(0.,-1.,-1.22464679914735E-16));
#5022=DIRECTION('ref_axis',(0.,-1.22464679914735E-16,1.));
#5023=DIRECTION('center_axis',(1.,0.,0.));
#5024=DIRECTION('ref_axis',(0.,0.,-1.));
#5025=DIRECTION('center_axis',(0.,-1.,-1.22464679914735E-16));
#5026=DIRECTION('ref_axis',(0.,-1.22464679914735E-16,1.));
#5027=DIRECTION('center_axis',(1.,0.,0.));
#5028=DIRECTION('ref_axis',(0.,0.,1.));
#5029=DIRECTION('center_axis',(1.,0.,0.));
#5030=DIRECTION('ref_axis',(0.,0.,-1.));
#5031=DIRECTION('',(-0.999999956307574,3.62016965808673E-20,-0.000295609285926949));
#5032=DIRECTION('center_axis',(-1.,0.,0.));
#5033=DIRECTION('ref_axis',(0.,0.,1.));
#5034=DIRECTION('center_axis',(1.,0.,0.));
#5035=DIRECTION('ref_axis',(0.,0.,-1.));
#5036=DIRECTION('center_axis',(0.,-1.,-1.22464679914735E-16));
#5037=DIRECTION('ref_axis',(0.,-1.22464679914735E-16,1.));
#5038=DIRECTION('center_axis',(1.,0.,0.));
#5039=DIRECTION('ref_axis',(0.,1.22464679914735E-16,1.));
#5040=DIRECTION('center_axis',(-1.,0.,0.));
#5041=DIRECTION('ref_axis',(0.,0.,1.));
#5042=DIRECTION('center_axis',(1.,0.,0.));
#5043=DIRECTION('ref_axis',(0.,0.,-1.));
#5044=DIRECTION('center_axis',(1.,0.,0.));
#5045=DIRECTION('ref_axis',(0.,0.,-1.));
#5046=DIRECTION('center_axis',(-1.,0.,0.));
#5047=DIRECTION('ref_axis',(0.,1.22464679914735E-16,1.));
#5048=DIRECTION('center_axis',(0.,-1.,-1.22464679914735E-16));
#5049=DIRECTION('ref_axis',(0.,-1.22464679914735E-16,1.));
#5050=DIRECTION('center_axis',(1.,0.,0.));
#5051=DIRECTION('ref_axis',(0.,0.,1.));
#5052=DIRECTION('center_axis',(1.,0.,0.));
#5053=DIRECTION('ref_axis',(0.,0.,-1.));
#5054=DIRECTION('',(-0.999999956307574,3.62016965810123E-20,-0.000295609285928133));
#5055=DIRECTION('center_axis',(-1.,0.,0.));
#5056=DIRECTION('ref_axis',(0.,0.,1.));
#5057=DIRECTION('center_axis',(1.,0.,0.));
#5058=DIRECTION('ref_axis',(0.,0.,-1.));
#5059=DIRECTION('center_axis',(1.,0.,0.));
#5060=DIRECTION('ref_axis',(0.,0.,-1.));
#5061=DIRECTION('center_axis',(1.,0.,0.));
#5062=DIRECTION('ref_axis',(0.,0.,-1.));
#5063=DIRECTION('center_axis',(0.,-1.,-1.22464679914735E-16));
#5064=DIRECTION('ref_axis',(0.,-1.22464679914735E-16,1.));
#5065=DIRECTION('center_axis',(1.,0.,0.));
#5066=DIRECTION('ref_axis',(0.,1.22464679914735E-16,1.));
#5067=DIRECTION('center_axis',(-1.,0.,0.));
#5068=DIRECTION('ref_axis',(0.,0.,1.));
#5069=DIRECTION('center_axis',(1.,0.,0.));
#5070=DIRECTION('ref_axis',(0.,0.,-1.));
#5071=DIRECTION('center_axis',(1.,0.,0.));
#5072=DIRECTION('ref_axis',(0.,0.,-1.));
#5073=DIRECTION('center_axis',(-1.,0.,0.));
#5074=DIRECTION('ref_axis',(0.,1.22464679914735E-16,1.));
#5075=DIRECTION('center_axis',(0.,-1.,-1.22464679914735E-16));
#5076=DIRECTION('ref_axis',(0.,-1.22464679914735E-16,1.));
#5077=DIRECTION('center_axis',(1.,0.,0.));
#5078=DIRECTION('ref_axis',(0.,1.22464679914735E-16,1.));
#5079=DIRECTION('center_axis',(-1.,0.,0.));
#5080=DIRECTION('ref_axis',(0.,0.,1.));
#5081=DIRECTION('center_axis',(1.,0.,0.));
#5082=DIRECTION('ref_axis',(0.,0.,-1.));
#5083=DIRECTION('',(-1.,0.,0.));
#5084=DIRECTION('center_axis',(1.,0.,0.));
#5085=DIRECTION('ref_axis',(0.,0.,-1.));
#5086=DIRECTION('',(-1.,0.,0.));
#5087=DIRECTION('center_axis',(1.,0.,0.));
#5088=DIRECTION('ref_axis',(0.,0.,-1.));
#5089=DIRECTION('',(-1.,0.,0.));
#15718=CARTESIAN_POINT('',(0.,0.,0.));
#15719=CARTESIAN_POINT('Origin',(66.9212607628943,0.,0.));
#15720=CARTESIAN_POINT('',(90.7335918111184,-2.00577712042713E-11,2.204));
#15721=CARTESIAN_POINT('',(90.6260478258334,0.0018616288768175,2.20399921377888));
#15722=CARTESIAN_POINT('',(66.9212607628943,-2.69912154532077E-16,2.204));
#15723=CARTESIAN_POINT('',(90.7336894293003,0.00186538422401548,2.20367257219299));
#15724=CARTESIAN_POINT('Ctrl Pts',(90.7335918111184,-2.00577712042713E-11,
2.204));
#15725=CARTESIAN_POINT('Ctrl Pts',(90.733561597852,0.000618820167389943,
2.20400000000001));
#15726=CARTESIAN_POINT('Ctrl Pts',(90.7335313878983,0.00123764367719169,
2.20399973937949));
#15727=CARTESIAN_POINT('Ctrl Pts',(90.7335011812186,0.0018564703451418,
2.20399921813005));
#15728=CARTESIAN_POINT('',(90.3514582376541,-0.174123623218802,-2.19796285666152));
#15729=CARTESIAN_POINT('Ctrl Pts',(90.7336894293003,0.00186538422401548,
2.20367257219299));
#15730=CARTESIAN_POINT('Ctrl Pts',(90.7297945009894,0.0795614518465619,
2.20378293938922));
#15731=CARTESIAN_POINT('Ctrl Pts',(90.7259488838733,0.157101568214134,2.19980889002447));
#15732=CARTESIAN_POINT('Ctrl Pts',(90.7220854782314,0.234095693825053,2.19178159250512));
#15733=CARTESIAN_POINT('Ctrl Pts',(90.7214381250115,0.246996848855024,2.19043653651615));
#15734=CARTESIAN_POINT('Ctrl Pts',(90.7207902723531,0.259882780727669,2.18897762717947));
#15735=CARTESIAN_POINT('Ctrl Pts',(90.720141604586,0.272751779700561,2.18740494157558));
#15736=CARTESIAN_POINT('Ctrl Pts',(90.7164410672004,0.346167192379334,2.1784330422952));
#15737=CARTESIAN_POINT('Ctrl Pts',(90.7127132590446,0.419029635902584,2.16575942048269));
#15738=CARTESIAN_POINT('Ctrl Pts',(90.7088849599204,0.490986234289347,2.14943329737029));
#15739=CARTESIAN_POINT('Ctrl Pts',(90.7079697249612,0.508188963819403,2.14553019624443));
#15740=CARTESIAN_POINT('Ctrl Pts',(90.7070487464506,0.525340152219468,2.14141830628492));
#15741=CARTESIAN_POINT('Ctrl Pts',(90.7061210239026,0.542435412378799,2.13709822000947));
#15742=CARTESIAN_POINT('Ctrl Pts',(90.7042020379602,0.577796807870508,2.12816215949207));
#15743=CARTESIAN_POINT('Ctrl Pts',(90.7022539890451,0.612917098866179,2.11833617853689));
#15744=CARTESIAN_POINT('Ctrl Pts',(90.7002675857539,0.647753314711685,2.10762898576747));
#15745=CARTESIAN_POINT('Ctrl Pts',(90.7002659993789,0.647781135499218,2.10762043482334));
#15746=CARTESIAN_POINT('Ctrl Pts',(90.7002644129794,0.647808956105774,2.10761188331721));
#15747=CARTESIAN_POINT('Ctrl Pts',(90.7002628265554,0.647836776531331,2.10760333124909));
#15748=CARTESIAN_POINT('Ctrl Pts',(90.6965577230164,0.712811561377226,2.08762992053154));
#15749=CARTESIAN_POINT('Ctrl Pts',(90.6927132629296,0.776943472303309,2.0645398564198));
#15750=CARTESIAN_POINT('Ctrl Pts',(90.6887955534437,0.839929315709657,2.03845326069095));
#15751=CARTESIAN_POINT('Ctrl Pts',(90.6884085760281,0.846150833407494,2.03587651950235));
#15752=CARTESIAN_POINT('Ctrl Pts',(90.6880208839337,0.852361146062634,2.03327057681406));
#15753=CARTESIAN_POINT('Ctrl Pts',(90.6876325408708,0.858559946859202,2.03063557170245));
#15754=CARTESIAN_POINT('Ctrl Pts',(90.6833190288938,0.927412989524639,2.00136731073919));
#15755=CARTESIAN_POINT('Ctrl Pts',(90.6789258022943,0.994849372636953,1.96850876260346));
#15756=CARTESIAN_POINT('Ctrl Pts',(90.6745280179299,1.06049739929679,1.93225792133409));
#15757=CARTESIAN_POINT('Ctrl Pts',(90.6701353803395,1.12606859737061,1.89604950481102));
#15758=CARTESIAN_POINT('Ctrl Pts',(90.6657385446255,1.18985584872898,1.85645702888921));
#15759=CARTESIAN_POINT('Ctrl Pts',(90.6613932375148,1.2515156647503,1.8137078109801));
#15760=CARTESIAN_POINT('Ctrl Pts',(90.6570506864659,1.3131363723121,1.77098570726246));
#15761=CARTESIAN_POINT('Ctrl Pts',(90.6527597693697,1.37263246530918,1.72511099080974));
#15762=CARTESIAN_POINT('Ctrl Pts',(90.6485531215493,1.42968534561502,1.67633745923008));
#15763=CARTESIAN_POINT('Ctrl Pts',(90.6443477744083,1.48672058538981,1.62757900823869));
#15764=CARTESIAN_POINT('Ctrl Pts',(90.6402329784846,1.5413063978217,1.57591591928549));
#15765=CARTESIAN_POINT('Ctrl Pts',(90.6362010534082,1.59316699803034,1.52164672579692));
#15766=CARTESIAN_POINT('Ctrl Pts',(90.632169064372,1.64502842092154,1.46737667141745));
#15767=CARTESIAN_POINT('Ctrl Pts',(90.6282324700559,1.6941492376414,1.41048483893202));
#15768=CARTESIAN_POINT('Ctrl Pts',(90.6243716777576,1.74026179806897,1.35128061019675));
#15769=CARTESIAN_POINT('Ctrl Pts',(90.6205068779001,1.78642222401146,1.2920149266026));
#15770=CARTESIAN_POINT('Ctrl Pts',(90.6167178746548,1.82956807036417,1.23043181827767));
#15771=CARTESIAN_POINT('Ctrl Pts',(90.6129652394984,1.8694534254963,1.16686432476613));
#15772=CARTESIAN_POINT('Ctrl Pts',(90.6092106191631,1.90935988035278,1.10326320345846));
#15773=CARTESIAN_POINT('Ctrl Pts',(90.6054920937299,1.94600205189049,1.03767547158359));
#15774=CARTESIAN_POINT('Ctrl Pts',(90.6017507504073,1.97916382080471,0.970463227410216));
#15775=CARTESIAN_POINT('Ctrl Pts',(90.5980026321539,2.01238563999263,0.903129273394721));
#15776=CARTESIAN_POINT('Ctrl Pts',(90.5942311045093,2.0421138920473,0.834164813775563));
#15777=CARTESIAN_POINT('Ctrl Pts',(90.5903635513674,2.06816820064445,0.763964378509355));
#15778=CARTESIAN_POINT('Ctrl Pts',(90.5873426674423,2.08851880453662,0.709131940878822));
#15779=CARTESIAN_POINT('Ctrl Pts',(90.5842627906181,2.10662855118927,0.653546080199383));
#15780=CARTESIAN_POINT('Ctrl Pts',(90.5810873112824,2.12243098826343,0.597407926020108));
#15781=CARTESIAN_POINT('Ctrl Pts',(90.5810857578706,2.12243871865304,0.597380463812735));
#15782=CARTESIAN_POINT('Ctrl Pts',(90.5810842044359,2.12244644849101,0.597353001472851));
#15783=CARTESIAN_POINT('Ctrl Pts',(90.5810826509783,2.12245417777735,0.597325539000468));
#15784=CARTESIAN_POINT('Ctrl Pts',(90.5773740556272,2.14090643281885,0.53176391766318));
#15785=CARTESIAN_POINT('Ctrl Pts',(90.5735258965146,2.15626954801148,0.465221864236195));
#15786=CARTESIAN_POINT('Ctrl Pts',(90.5696041138388,2.16848067480506,0.398020314951632));
#15787=CARTESIAN_POINT('Ctrl Pts',(90.5692131468832,2.16969801586171,0.391320916411502));
#15788=CARTESIAN_POINT('Ctrl Pts',(90.568821448233,2.17088404874851,0.384615002656172));
#15789=CARTESIAN_POINT('Ctrl Pts',(90.5684290832191,2.17203872326328,0.377902917265477));
#15790=CARTESIAN_POINT('Ctrl Pts',(90.5641072789612,2.18475717944205,0.30397094525284));
#15791=CARTESIAN_POINT('Ctrl Pts',(90.5597052322467,2.1936691058592,0.229284601525099));
#15792=CARTESIAN_POINT('Ctrl Pts',(90.5552981347378,2.19874006138384,0.154265805746006));
#15793=CARTESIAN_POINT('Ctrl Pts',(90.5508962519783,2.20380501664133,0.0793357768302387));
#15794=CARTESIAN_POINT('Ctrl Pts',(90.5464896818778,2.20503846321057,0.0040740489741147));
#15795=CARTESIAN_POINT('Ctrl Pts',(90.5421341666814,2.20244590853611,-0.0711054635678189));
#15796=CARTESIAN_POINT('Ctrl Pts',(90.5377814559523,2.19985502317853,-0.146236568865197));
#15797=CARTESIAN_POINT('Ctrl Pts',(90.5334799059467,2.19344323608003,-0.221285605287203));
#15798=CARTESIAN_POINT('Ctrl Pts',(90.5292621250607,2.18325177058937,-0.295845329434535));
#15799=CARTESIAN_POINT('Ctrl Pts',(90.52504570996,2.17306360525912,-0.370380909944266));
#15800=CARTESIAN_POINT('Ctrl Pts',(90.520915988809,2.15909328609742,-0.444426385491838));
#15801=CARTESIAN_POINT('Ctrl Pts',(90.5168735963798,2.14142863128311,-0.517583194118507));
#15802=CARTESIAN_POINT('Ctrl Pts',(90.5128312191312,2.12376404280608,-0.590739728014407));
#15803=CARTESIAN_POINT('Ctrl Pts',(90.5088819801313,2.10239512026904,-0.663005499997299));
#15804=CARTESIAN_POINT('Ctrl Pts',(90.5050078670583,2.07743449591428,-0.733985551508349));
#15805=CARTESIAN_POINT('Ctrl Pts',(90.5011299379722,2.05244928526926,-0.805035518584183));
#15806=CARTESIAN_POINT('Ctrl Pts',(90.4973271166733,2.02386508098874,-0.874797196413565));
#15807=CARTESIAN_POINT('Ctrl Pts',(90.4935598951022,1.99182912744931,-0.942881395836193));
#15808=CARTESIAN_POINT('Ctrl Pts',(90.4897907742079,1.95977702231683,-1.01099992132566));
#15809=CARTESIAN_POINT('Ctrl Pts',(90.486056972178,1.92426938925078,-1.0774390560734));
#15810=CARTESIAN_POINT('Ctrl Pts',(90.4822995779161,1.88549419873164,-1.14181879687684));
#15811=CARTESIAN_POINT('Ctrl Pts',(90.4785356605338,1.84665169155259,-1.20631030577369));
#15812=CARTESIAN_POINT('Ctrl Pts',(90.4747475531196,1.80452988119458,-1.26873485386227));
#15813=CARTESIAN_POINT('Ctrl Pts',(90.4708628272517,1.75936358523186,-1.32872489694982));
#15814=CARTESIAN_POINT('Ctrl Pts',(90.4679364284152,1.72533940940893,-1.37391593442875));
#15815=CARTESIAN_POINT('Ctrl Pts',(90.4649548266515,1.68958847284266,-1.41772564327571));
#15816=CARTESIAN_POINT('Ctrl Pts',(90.4618853553014,1.65223033111774,-1.46000507888003));
#15817=CARTESIAN_POINT('Ctrl Pts',(90.4618838551247,1.65221207265925,-1.460025742577));
#15818=CARTESIAN_POINT('Ctrl Pts',(90.4618823549269,1.65219381381683,-1.46004640590898));
#15819=CARTESIAN_POINT('Ctrl Pts',(90.4618808547082,1.65217555459052,-1.46006706887596));
#15820=CARTESIAN_POINT('Ctrl Pts',(90.4581925626705,1.60728519424155,-1.51086703256677));
#15821=CARTESIAN_POINT('Ctrl Pts',(90.454368077417,1.55991156807906,-1.55963231878916));
#15822=CARTESIAN_POINT('Ctrl Pts',(90.4504725371015,1.51028778213619,-1.60613397507167));
#15823=CARTESIAN_POINT('Ctrl Pts',(90.4501137585467,1.50571744047351,-1.6104167691603));
#15824=CARTESIAN_POINT('Ctrl Pts',(90.4497543772762,1.50112804824368,-1.61468035702652));
#15825=CARTESIAN_POINT('Ctrl Pts',(90.4493944441774,1.49651980955262,-1.61892455710779));
#15826=CARTESIAN_POINT('Ctrl Pts',(90.4450546253874,1.44095692598081,-1.67009812054065));
#15827=CARTESIAN_POINT('Ctrl Pts',(90.4406352299576,1.38264828060835,-1.71845427083435));
#15828=CARTESIAN_POINT('Ctrl Pts',(90.4362128090986,1.3219392900851,-1.76372396404811));
#15829=CARTESIAN_POINT('Ctrl Pts',(90.4318748345868,1.2623895407686,-1.80812923020853));
#15830=CARTESIAN_POINT('Ctrl Pts',(90.4275342347738,1.20053049057327,-1.8495651987225));
#15831=CARTESIAN_POINT('Ctrl Pts',(90.4232444676202,1.13670532799525,-1.88781504244614));
#15832=CARTESIAN_POINT('Ctrl Pts',(90.4189572002254,1.0729173579975,-1.92604259699218));
#15833=CARTESIAN_POINT('Ctrl Pts',(90.4147208685469,1.00716565231536,-1.96108787795614));
#15834=CARTESIAN_POINT('Ctrl Pts',(90.4105665447433,0.939807813952254,-1.99276793951803));
#15835=CARTESIAN_POINT('Ctrl Pts',(90.406413233415,0.872466391775119,-2.02444028014061));
#15836=CARTESIAN_POINT('Ctrl Pts',(90.4023419306153,0.80351966725319,-2.05274904906297));
#15837=CARTESIAN_POINT('Ctrl Pts',(90.3983599093118,0.733339033107106,-2.07754385959433));
#15838=CARTESIAN_POINT('Ctrl Pts',(90.3942374240011,0.660682808715153,-2.10321329589457));
#15839=CARTESIAN_POINT('Ctrl Pts',(90.3902107121892,0.586704040681358,-2.12511616524922));
#15840=CARTESIAN_POINT('Ctrl Pts',(90.386261178544,0.511830009240368,-2.14312305697451));
#15841=CARTESIAN_POINT('Ctrl Pts',(90.3824419404883,0.439426081094696,-2.16053589917779));
#15842=CARTESIAN_POINT('Ctrl Pts',(90.3786945635058,0.366185095016135,-2.17430556237347));
#15843=CARTESIAN_POINT('Ctrl Pts',(90.3749798984358,0.292506650500107,-2.18435136400926));
#15844=CARTESIAN_POINT('Ctrl Pts',(90.3710751413363,0.215057829709192,-2.19491124343806));
#15845=CARTESIAN_POINT('Ctrl Pts',(90.367206325069,0.137125588283632,-2.20135558254538));
#15846=CARTESIAN_POINT('Ctrl Pts',(90.3633062801793,0.0591887388210525,
-2.20363835003113));
#15847=CARTESIAN_POINT('Ctrl Pts',(90.359781207124,-0.0112548319128014,
-2.20570163965549));
#15848=CARTESIAN_POINT('Ctrl Pts',(90.3562300839869,-0.0817028455918926,
-2.20436504621134));
#15849=CARTESIAN_POINT('Ctrl Pts',(90.3525926877338,-0.151789755927138,
-2.19963533387595));
#15850=CARTESIAN_POINT('Ctrl Pts',(90.3522060658021,-0.159239353050694,
-2.19913260874168));
#15851=CARTESIAN_POINT('Ctrl Pts',(90.3518184691787,-0.166684913452266,
-2.19859157174713));
#15852=CARTESIAN_POINT('Ctrl Pts',(90.3514298255451,-0.174126029259769,
-2.19801224645037));
#15853=CARTESIAN_POINT('',(90.3498698986825,-0.214101726762253,-2.19357617843498));
#15854=CARTESIAN_POINT('Ctrl Pts',(90.3519463663221,-0.174082286703647,
-2.19711432507641));
#15855=CARTESIAN_POINT('Ctrl Pts',(90.3516028176952,-0.180756616910668,
-2.19658550295199));
#15856=CARTESIAN_POINT('Ctrl Pts',(90.3512580795196,-0.187428441846501,
-2.1960262757715));
#15857=CARTESIAN_POINT('Ctrl Pts',(90.3505659730386,-0.200768470428712,
-2.19484688993294));
#15858=CARTESIAN_POINT('Ctrl Pts',(90.3502186079292,-0.207436597587503,
-2.1942267214521));
#15859=CARTESIAN_POINT('Ctrl Pts',(90.3498698986825,-0.214101726762254,
-2.19357617843498));
#15860=CARTESIAN_POINT('',(90.3498698986825,-2.69912154532077E-16,2.204));
#15861=CARTESIAN_POINT('Origin',(90.3498698986825,0.,0.));
#15862=CARTESIAN_POINT('',(33.4926516271063,2.69912154532077E-16,2.204));
#15863=CARTESIAN_POINT('',(66.9212607628943,-2.69912154532077E-16,2.204));
#15864=CARTESIAN_POINT('Origin',(33.4926516271063,0.,0.));
#15865=CARTESIAN_POINT('',(90.3498698986825,1.62325119196235,-1.49086269246796));
#15866=CARTESIAN_POINT('Origin',(90.3498698986825,0.,0.));
#15867=CARTESIAN_POINT('Ctrl Pts',(90.3498698986825,1.62325119196235,-1.49086269246796));
#15868=CARTESIAN_POINT('Ctrl Pts',(90.3540342343737,1.67526300385128,-1.43423223543702));
#15869=CARTESIAN_POINT('Ctrl Pts',(90.358198570065,1.72434765652125,-1.37483397863705));
#15870=CARTESIAN_POINT('Ctrl Pts',(90.3623629057562,1.77021263623129,-1.31299779989422));
#15871=CARTESIAN_POINT('Ctrl Pts',(90.366524563556,1.8160481222971,-1.25120138513401));
#15872=CARTESIAN_POINT('Ctrl Pts',(90.3706862213558,1.8586677886908,-1.18697052503797));
#15873=CARTESIAN_POINT('Ctrl Pts',(90.3748478791556,1.89781988675447,-1.120667514225));
#15874=CARTESIAN_POINT('Ctrl Pts',(90.379009024366,1.93696716247229,-1.05437266992329));
#15875=CARTESIAN_POINT('Ctrl Pts',(90.3831701695763,1.97264748370526,-0.98600656164491));
#15876=CARTESIAN_POINT('Ctrl Pts',(90.3873313147867,2.00465335684887,-0.915959015936052));
#15877=CARTESIAN_POINT('Ctrl Pts',(90.3914923669492,2.03665851430572,-0.845913036567883));
#15878=CARTESIAN_POINT('Ctrl Pts',(90.3956534191117,2.06498920101561,-0.774186100698475));
#15879=CARTESIAN_POINT('Ctrl Pts',(90.3998144712743,2.08948530986951,-0.701189803005941));
#15880=CARTESIAN_POINT('Ctrl Pts',(90.4039765044813,2.11398719413109,-0.628176295095227));
#15881=CARTESIAN_POINT('Ctrl Pts',(90.4081385376883,2.13465256077998,-0.553893253843861));
#15882=CARTESIAN_POINT('Ctrl Pts',(90.4123005708953,2.15137097947947,-0.478768115744507));
#15883=CARTESIAN_POINT('Ctrl Pts',(90.4164646600594,2.16809765672722,-0.403605867402304));
#15884=CARTESIAN_POINT('Ctrl Pts',(90.4206287492236,2.18087341220672,-0.327601130908672));
#15885=CARTESIAN_POINT('Ctrl Pts',(90.4247928383877,2.1896390276492,-0.251191020133017));
#15886=CARTESIAN_POINT('Ctrl Pts',(90.4289632381674,2.19841792725226,-0.174665110964433));
#15887=CARTESIAN_POINT('Ctrl Pts',(90.4331336379471,2.203174502206,-0.0977330455384561));
#15888=CARTESIAN_POINT('Ctrl Pts',(90.4373040377268,2.20390150594005,-0.0208363172176138));
#15889=CARTESIAN_POINT('Ctrl Pts',(90.4414778779445,2.20462910942745,0.056123848288982));
#15890=CARTESIAN_POINT('Ctrl Pts',(90.4456517181622,2.20132053768274,0.133048172453329));
#15891=CARTESIAN_POINT('Ctrl Pts',(90.4498255583799,2.19402060648631,0.20949839692337));
#15892=CARTESIAN_POINT('Ctrl Pts',(90.4540074390487,2.18670661276303,0.286095894471075));
#15893=CARTESIAN_POINT('Ctrl Pts',(90.4581893197175,2.17538596621945,0.362217025950471));
#15894=CARTESIAN_POINT('Ctrl Pts',(90.4623712003864,2.16015491417952,0.437431990995269));
#15895=CARTESIAN_POINT('Ctrl Pts',(90.4645876718248,2.15208218458796,0.477297265728303));
#15896=CARTESIAN_POINT('Ctrl Pts',(90.4668041432632,2.14291180085852,0.516908206597404));
#15897=CARTESIAN_POINT('Ctrl Pts',(90.4690206147016,2.13266372326016,0.55620270000255));
#15898=CARTESIAN_POINT('Ctrl Pts',(90.473057969927,2.11399660717457,0.627778550485544));
#15899=CARTESIAN_POINT('Ctrl Pts',(90.4770953251523,2.09167923412068,0.698577635480653));
#15900=CARTESIAN_POINT('Ctrl Pts',(90.4811326803776,2.06579110704165,0.768194703228045));
#15901=CARTESIAN_POINT('Ctrl Pts',(90.4851634929537,2.03994493241042,0.837698954532925));
#15902=CARTESIAN_POINT('Ctrl Pts',(90.4891943055299,2.01053965260703,0.906024537409715));
#15903=CARTESIAN_POINT('Ctrl Pts',(90.493225118106,1.97770533275813,0.972778297856222));
#15904=CARTESIAN_POINT('Ctrl Pts',(90.4972504974604,1.94491527101734,1.03944207942818));
#15905=CARTESIAN_POINT('Ctrl Pts',(90.5012758768148,1.90870556178229,1.10453781181376));
#15906=CARTESIAN_POINT('Ctrl Pts',(90.5053012561693,1.86925480157049,1.16769109220105));
#15907=CARTESIAN_POINT('Ctrl Pts',(90.5093236563983,1.82983323829924,1.23079763375331));
#15908=CARTESIAN_POINT('Ctrl Pts',(90.5133460566273,1.78717563777286,1.291964162283));
#15909=CARTESIAN_POINT('Ctrl Pts',(90.5173684568564,1.74150642743007,1.35084098369118));
#15910=CARTESIAN_POINT('Ctrl Pts',(90.5213892394597,1.6958555831581,1.40969412753051));
#15911=CARTESIAN_POINT('Ctrl Pts',(90.5254100220631,1.64719583023854,1.46625900656898));
#15912=CARTESIAN_POINT('Ctrl Pts',(90.5294308046664,1.59579380100114,1.52021647954702));
#15913=CARTESIAN_POINT('Ctrl Pts',(90.5334513289884,1.54439507365432,1.57417048648151));
#15914=CARTESIAN_POINT('Ctrl Pts',(90.5374718533105,1.49025475691073,1.62551706820624));
#15915=CARTESIAN_POINT('Ctrl Pts',(90.5414923776325,1.43367730249767,1.67397293655035));
#15916=CARTESIAN_POINT('Ctrl Pts',(90.545516831533,1.37704455043435,1.72247616467211));
#15917=CARTESIAN_POINT('Ctrl Pts',(90.5495412854335,1.31797027415438,1.76808271884422));
#15918=CARTESIAN_POINT('Ctrl Pts',(90.553565739334,1.25679240448188,1.81054932328193));
#15919=CARTESIAN_POINT('Ctrl Pts',(90.5575921261865,1.19558515097667,1.85303632450049));
#15920=CARTESIAN_POINT('Ctrl Pts',(90.5616185130389,1.1322727072202,1.8923801166326));
#15921=CARTESIAN_POINT('Ctrl Pts',(90.5656448998913,1.06722004242361,1.92838206303869));
#15922=CARTESIAN_POINT('Ctrl Pts',(90.5696786738581,1.0020480270792,1.96445006134349));
#15923=CARTESIAN_POINT('Ctrl Pts',(90.5737124478249,0.935129852251466,1.99716375370825));
#15924=CARTESIAN_POINT('Ctrl Pts',(90.5777462217918,0.866852550327255,2.02637179609052));
#15925=CARTESIAN_POINT('Ctrl Pts',(90.5812212581014,0.808032669673591,2.0515340904202));
#15926=CARTESIAN_POINT('Ctrl Pts',(90.5846962944111,0.748204602075248,2.07409538561612));
#15927=CARTESIAN_POINT('Ctrl Pts',(90.5881713307208,0.687623727431014,2.09398892295873));
#15928=CARTESIAN_POINT('Ctrl Pts',(90.5930975172393,0.60174471456295,2.12218985864133));
#15929=CARTESIAN_POINT('Ctrl Pts',(90.5980237037578,0.514066413824007,2.14512431597063));
#15930=CARTESIAN_POINT('Ctrl Pts',(90.6029498902764,0.425177719435792,2.16260026516584));
#15931=CARTESIAN_POINT('Ctrl Pts',(90.6078130617383,0.337426076211533,2.1798526645777));
#15932=CARTESIAN_POINT('Ctrl Pts',(90.6126762332001,0.248494831068513,2.19178526875751));
#15933=CARTESIAN_POINT('Ctrl Pts',(90.617539404662,0.158971471143045,2.19825932759595));
#15934=CARTESIAN_POINT('Ctrl Pts',(90.6203755450525,0.106762574342893,2.20203491723039));
#15935=CARTESIAN_POINT('Ctrl Pts',(90.6232116854429,0.0543526856127783,
2.20395487670908));
#15936=CARTESIAN_POINT('Ctrl Pts',(90.6260478258334,0.0018616288768175,
2.20399921377888));
#15937=CARTESIAN_POINT('',(70.8,1.96408146470558,0.999999999999996));
#15938=CARTESIAN_POINT('',(69.8,2.204,1.22464679914735E-16));
#15939=CARTESIAN_POINT('Ctrl Pts',(70.8,1.96408146470558,0.999999999999995));
#15940=CARTESIAN_POINT('Ctrl Pts',(70.6722659399236,1.96408146470558,0.999999999999995));
#15941=CARTESIAN_POINT('Ctrl Pts',(70.5375729856138,1.97786636144381,0.974089083852149));
#15942=CARTESIAN_POINT('Ctrl Pts',(70.2919072356979,2.02515309008955,0.871527146747205));
#15943=CARTESIAN_POINT('Ctrl Pts',(70.1807303328797,2.05773682352636,0.794943895252836));
#15944=CARTESIAN_POINT('Ctrl Pts',(70.0052106451649,2.11719154668924,0.619424207537946));
#15945=CARTESIAN_POINT('Ctrl Pts',(69.9285120447932,2.14824329851503,0.508191937532767));
#15946=CARTESIAN_POINT('Ctrl Pts',(69.8258593644549,2.19189597286799,0.262298234370078));
#15947=CARTESIAN_POINT('Ctrl Pts',(69.8,2.204,0.127509325063069));
#15948=CARTESIAN_POINT('Ctrl Pts',(69.8,2.204,-1.04083408558608E-15));
#15949=CARTESIAN_POINT('Ctrl Pts',(69.8,2.204,9.36750677027476E-16));
#15950=CARTESIAN_POINT('Ctrl Pts',(69.8,2.204,-0.12750932506307));
#15951=CARTESIAN_POINT('Ctrl Pts',(69.8258593644549,2.19189597286799,-0.262298234370079));
#15952=CARTESIAN_POINT('Ctrl Pts',(69.9285120447932,2.14824329851503,-0.508191937532767));
#15953=CARTESIAN_POINT('Ctrl Pts',(70.0052106451649,2.11719154668924,-0.619424207537946));
#15954=CARTESIAN_POINT('Ctrl Pts',(70.1807303328797,2.05773682352636,-0.794943895252837));
#15955=CARTESIAN_POINT('Ctrl Pts',(70.2919072356979,2.02515309008955,-0.871527146747215));
#15956=CARTESIAN_POINT('Ctrl Pts',(70.5375729856138,1.97786636144381,-0.974089083852154));
#15957=CARTESIAN_POINT('Ctrl Pts',(70.6722659399236,1.96408146470558,-0.999999999999996));
#15958=CARTESIAN_POINT('Ctrl Pts',(70.9277340600764,1.96408146470558,-0.999999999999996));
#15959=CARTESIAN_POINT('Ctrl Pts',(71.0624270143862,1.97786636144381,-0.974089083852144));
#15960=CARTESIAN_POINT('Ctrl Pts',(71.3080927643021,2.02515309008955,-0.871527146747202));
#15961=CARTESIAN_POINT('Ctrl Pts',(71.4192696671203,2.05773682352636,-0.794943895252837));
#15962=CARTESIAN_POINT('Ctrl Pts',(71.5947893548351,2.11719154668924,-0.619424207537946));
#15963=CARTESIAN_POINT('Ctrl Pts',(71.6714879552068,2.14824329851503,-0.508191937532762));
#15964=CARTESIAN_POINT('Ctrl Pts',(71.7741406355451,2.19189597286799,-0.262298234370079));
#15965=CARTESIAN_POINT('Ctrl Pts',(71.8,2.204,-0.127509325063071));
#15966=CARTESIAN_POINT('Ctrl Pts',(71.8,2.204,0.12750932506307));
#15967=CARTESIAN_POINT('Ctrl Pts',(71.7741406355451,2.19189597286799,0.262298234370079));
#15968=CARTESIAN_POINT('Ctrl Pts',(71.6714879552068,2.14824329851503,0.508191937532767));
#15969=CARTESIAN_POINT('Ctrl Pts',(71.5947893548351,2.11719154668924,0.619424207537946));
#15970=CARTESIAN_POINT('Ctrl Pts',(71.4192696671203,2.05773682352636,0.794943895252837));
#15971=CARTESIAN_POINT('Ctrl Pts',(71.3080927643021,2.02515309008955,0.871527146747205));
#15972=CARTESIAN_POINT('Ctrl Pts',(71.0624270143862,1.97786636144381,0.974089083852149));
#15973=CARTESIAN_POINT('Ctrl Pts',(70.9277340600764,1.96408146470558,0.999999999999996));
#15974=CARTESIAN_POINT('Ctrl Pts',(70.8,1.96408146470558,0.999999999999996));
#15975=CARTESIAN_POINT('Origin',(66.9212607628943,0.,0.));
#15976=CARTESIAN_POINT('',(91.4824158962551,-3.3646198792706E-12,2.204));
#15977=CARTESIAN_POINT('',(91.3776298668357,4.55134372080087E-12,2.204));
#15978=CARTESIAN_POINT('',(66.9212607628943,-2.69912154532077E-16,2.204));
#15979=CARTESIAN_POINT('Ctrl Pts',(91.4824158962551,-3.3646198792706E-12,
2.204));
#15980=CARTESIAN_POINT('Ctrl Pts',(91.4801781402797,0.0394543598407125,
2.20400000000006));
#15981=CARTESIAN_POINT('Ctrl Pts',(91.4779713869581,0.0789033116011558,
2.20294058194433));
#15982=CARTESIAN_POINT('Ctrl Pts',(91.4749196852296,0.134210744976245,2.1999675487167));
#15983=CARTESIAN_POINT('Ctrl Pts',(91.4740474214224,0.150107529048946,2.19894008286232));
#15984=CARTESIAN_POINT('Ctrl Pts',(91.4725385729675,0.177755683031999,2.19685185866944));
#15985=CARTESIAN_POINT('Ctrl Pts',(91.4718995767405,0.189512119582209,2.19586892502936));
#15986=CARTESIAN_POINT('Ctrl Pts',(91.4705665597984,0.214133982223726,2.19361112414296));
#15987=CARTESIAN_POINT('Ctrl Pts',(91.4698731598011,0.226997251520984,2.19231735475216));
#15988=CARTESIAN_POINT('Ctrl Pts',(91.4682214240739,0.257766309931557,2.18894893085676));
#15989=CARTESIAN_POINT('Ctrl Pts',(91.4672664776349,0.275659637616388,2.18676763340557));
#15990=CARTESIAN_POINT('Ctrl Pts',(91.4639474872967,0.338186307846201,2.17836560523575));
#15991=CARTESIAN_POINT('Ctrl Pts',(91.4616194683117,0.382655249285325,2.17099562685355));
#15992=CARTESIAN_POINT('Ctrl Pts',(91.4559115143877,0.492756803489202,2.14925966686931));
#15993=CARTESIAN_POINT('Ctrl Pts',(91.4525792516709,0.558018222403516,2.13324702402587));
#15994=CARTESIAN_POINT('Ctrl Pts',(91.4423562410431,0.758380775879455,2.0742597226521));
#15995=CARTESIAN_POINT('Ctrl Pts',(91.4356619409826,0.890127883662804,2.02122821920269));
#15996=CARTESIAN_POINT('Ctrl Pts',(91.4256608296784,1.06843326519412,1.92861997232397));
#15997=CARTESIAN_POINT('Ctrl Pts',(91.4226505681136,1.11987386384554,1.89921196367638));
#15998=CARTESIAN_POINT('Ctrl Pts',(91.418782576099,1.18197488347845,1.86030882788842));
#15999=CARTESIAN_POINT('Ctrl Pts',(91.418034226323,1.19381429645149,1.85273337679333));
#16000=CARTESIAN_POINT('Ctrl Pts',(91.4168465492248,1.21230993013197,1.84064805438785));
#16001=CARTESIAN_POINT('Ctrl Pts',(91.4164120628725,1.21901550713279,1.83621398970867));
#16002=CARTESIAN_POINT('Ctrl Pts',(91.4155854183853,1.23165467731864,1.82775658928307));
#16003=CARTESIAN_POINT('Ctrl Pts',(91.4151937531492,1.23759307706115,1.8237408708577));
#16004=CARTESIAN_POINT('Ctrl Pts',(91.4142594981588,1.25164198962775,1.81414037494941));
#16005=CARTESIAN_POINT('Ctrl Pts',(91.4137152302728,1.25973480475251,1.80853011707421));
#16006=CARTESIAN_POINT('Ctrl Pts',(91.4118607479087,1.28701252139134,1.78934821077243));
#16007=CARTESIAN_POINT('Ctrl Pts',(91.4105349742071,1.30601725021243,1.77552445805128));
#16008=CARTESIAN_POINT('Ctrl Pts',(91.4072327079099,1.3522561000108,1.74074697169256));
#16009=CARTESIAN_POINT('Ctrl Pts',(91.4052391501105,1.37922776628106,1.71945547580777));
#16010=CARTESIAN_POINT('Ctrl Pts',(91.3964224042232,1.49497838962054,1.62360553138485));
#16011=CARTESIAN_POINT('Ctrl Pts',(91.3893940912104,1.57829249398324,1.54274017667738));
#16012=CARTESIAN_POINT('Ctrl Pts',(91.3750887937157,1.73622748421512,1.3631975731532));
#16013=CARTESIAN_POINT('Ctrl Pts',(91.3678528592593,1.80970648731728,1.26402655137352));
#16014=CARTESIAN_POINT('Ctrl Pts',(91.3591979627015,1.89075204382571,1.13297187962658));
#16015=CARTESIAN_POINT('Ctrl Pts',(91.3574839966505,1.90643258991293,1.10638306549075));
#16016=CARTESIAN_POINT('Ctrl Pts',(91.3549239995837,1.92928036877724,1.06571214141963));
#16017=CARTESIAN_POINT('Ctrl Pts',(91.3540631744631,1.93686275312465,1.05186871973477));
#16018=CARTESIAN_POINT('Ctrl Pts',(91.3525243078238,1.95023304031517,1.02682326907866));
#16019=CARTESIAN_POINT('Ctrl Pts',(91.3518443765184,1.95607471014771,1.01565086274235));
#16020=CARTESIAN_POINT('Ctrl Pts',(91.3503974079138,1.96836276081221,0.991650209408952));
#16021=CARTESIAN_POINT('Ctrl Pts',(91.3496314056636,1.97478033298395,0.978807818604067));
#16022=CARTESIAN_POINT('Ctrl Pts',(91.34754902315,1.99198104901975,0.943529076235189));
#16023=CARTESIAN_POINT('Ctrl Pts',(91.3462414464137,2.00251046811188,0.920970959756128));
#16024=CARTESIAN_POINT('Ctrl Pts',(91.336926036561,2.07547225740982,0.757487723957267));
#16025=CARTESIAN_POINT('Ctrl Pts',(91.329443973503,2.12335272623722,0.610534215965251));
#16026=CARTESIAN_POINT('Ctrl Pts',(91.3154590438008,2.18371514442958,0.327543255072804));
#16027=CARTESIAN_POINT('Ctrl Pts',(91.3089636843362,2.19968962679294,0.193012387603668));
#16028=CARTESIAN_POINT('Ctrl Pts',(91.3009677739356,2.2037152438386,0.0397857276844529));
#16029=CARTESIAN_POINT('Ctrl Pts',(91.300013456607,2.20396769519286,0.0216826630416138));
#16030=CARTESIAN_POINT('Ctrl Pts',(91.2985665448823,2.20401174040237,-0.00544011018295865));
#16031=CARTESIAN_POINT('Ctrl Pts',(91.2980825714011,2.2039710236282,-0.0144591830885269));
#16032=CARTESIAN_POINT('Ctrl Pts',(91.2972039685478,2.20379769732076,-0.0307295685720725));
#16033=CARTESIAN_POINT('Ctrl Pts',(91.2968104085057,2.20368464963887,-0.0379810569206739));
#16034=CARTESIAN_POINT('Ctrl Pts',(91.295996679291,2.20337850948319,-0.0528951323439904));
#16035=CARTESIAN_POINT('Ctrl Pts',(91.2955762981024,2.20318123234762,-0.0605574505010265));
#16036=CARTESIAN_POINT('Ctrl Pts',(91.2944730727269,2.20256178718748,-0.0805608770538496));
#16037=CARTESIAN_POINT('Ctrl Pts',(91.2937868365485,2.2020758697894,-0.0928995722403264));
#16038=CARTESIAN_POINT('Ctrl Pts',(91.2906575360942,2.19940691485961,-0.148734287476722));
#16039=CARTESIAN_POINT('Ctrl Pts',(91.2881578825651,2.1960387436545,-0.192161395489317));
#16040=CARTESIAN_POINT('Ctrl Pts',(91.2805869618852,2.18216995964079,-0.32123739224586));
#16041=CARTESIAN_POINT('Ctrl Pts',(91.275407878687,2.16792481370537,-0.406398663174594));
#16042=CARTESIAN_POINT('Ctrl Pts',(91.2604311365895,2.11244703903914,-0.649428606466381));
#16043=CARTESIAN_POINT('Ctrl Pts',(91.250710854518,2.05864191430014,-0.803865237988029));
#16044=CARTESIAN_POINT('Ctrl Pts',(91.2400206920276,1.97644576677972,-0.975720710666994));
#16045=CARTESIAN_POINT('Ctrl Pts',(91.2384965382159,1.96414602370372,-1.00024960259684));
#16046=CARTESIAN_POINT('Ctrl Pts',(91.2360889387296,1.94378590658349,-1.03902839588803));
#16047=CARTESIAN_POINT('Ctrl Pts',(91.2351953297012,1.93601954951955,-1.05342867928696));
#16048=CARTESIAN_POINT('Ctrl Pts',(91.2336179184206,1.92193856320357,-1.07885567519416));
#16049=CARTESIAN_POINT('Ctrl Pts',(91.23293188587,1.91568763550544,-1.08991664875825));
#16050=CARTESIAN_POINT('Ctrl Pts',(91.2315037355365,1.90240995760003,-1.11294425046954));
#16051=CARTESIAN_POINT('Ctrl Pts',(91.230762311013,1.89536511547899,-1.12489983666365));
#16052=CARTESIAN_POINT('Ctrl Pts',(91.2288213843301,1.87652588338641,-1.15619184060402));
#16053=CARTESIAN_POINT('Ctrl Pts',(91.2276287173098,1.86454537908809,-1.17541462598263));
#16054=CARTESIAN_POINT('Ctrl Pts',(91.2217305794806,1.80331407730494,-1.27036790582983));
#16055=CARTESIAN_POINT('Ctrl Pts',(91.2171888958627,1.74973425701063,-1.34320833345299));
#16056=CARTESIAN_POINT('Ctrl Pts',(91.2081357489223,1.63181796360114,-1.48443722380726));
#16057=CARTESIAN_POINT('Ctrl Pts',(91.2036405300379,1.56728530893299,-1.55241775699004));
#16058=CARTESIAN_POINT('Ctrl Pts',(91.1977522743822,1.47814337143887,-1.63508054515882));
#16059=CARTESIAN_POINT('Ctrl Pts',(91.1963959538015,1.45730292382031,-1.65368206473617));
#16060=CARTESIAN_POINT('Ctrl Pts',(91.1906734065766,1.36845661683924,-1.72999933951523));
#16061=CARTESIAN_POINT('Ctrl Pts',(91.1862372482116,1.29733928572496,-1.78395035269217));
#16062=CARTESIAN_POINT('Ctrl Pts',(91.180749987825,1.21063959493721,-1.84179103655169));
#16063=CARTESIAN_POINT('Ctrl Pts',(91.179950438576,1.19803652024295,-1.8500137628203));
#16064=CARTESIAN_POINT('Ctrl Pts',(91.1786948322767,1.17831612219093,-1.86259408827682));
#16065=CARTESIAN_POINT('Ctrl Pts',(91.1782444438249,1.1712563536404,-1.8670415557535));
#16066=CARTESIAN_POINT('Ctrl Pts',(91.1774054345939,1.15813586424978,-1.87520341503529));
#16067=CARTESIAN_POINT('Ctrl Pts',(91.1770175288974,1.15208223324073,-1.87892869771563));
#16068=CARTESIAN_POINT('Ctrl Pts',(91.176116045132,1.13804140460854,-1.88747577598316));
#16069=CARTESIAN_POINT('Ctrl Pts',(91.1756011282147,1.13004152511208,-1.89227619246865));
#16070=CARTESIAN_POINT('Ctrl Pts',(91.173945446253,1.10437265942562,-1.907458256576));
#16071=CARTESIAN_POINT('Ctrl Pts',(91.1727931761148,1.08658974413816,-1.91764403316666));
#16072=CARTESIAN_POINT('Ctrl Pts',(91.1663870173423,0.987996445036268,-1.97230506420663));
#16073=CARTESIAN_POINT('Ctrl Pts',(91.1609074946563,0.904602956887268,-2.01191822435199));
#16074=CARTESIAN_POINT('Ctrl Pts',(91.145420579204,0.664707189880399,-2.10793589015116));
#16075=CARTESIAN_POINT('Ctrl Pts',(91.135397274314,0.503920223382356,-2.15204740998207));
#16076=CARTESIAN_POINT('Ctrl Pts',(91.1234505367509,0.296591852644385,-2.18438823761559));
#16077=CARTESIAN_POINT('Ctrl Pts',(91.1210043986397,0.253301082733593,-2.18983050493573));
#16078=CARTESIAN_POINT('Ctrl Pts',(91.1175898111436,0.191676504015374,-2.19572546887252));
#16079=CARTESIAN_POINT('Ctrl Pts',(91.116588542128,0.17345665490953,-2.19723986723269));
#16080=CARTESIAN_POINT('Ctrl Pts',(91.1148957197791,0.142403616795862,-2.19943226310102));
#16081=CARTESIAN_POINT('Ctrl Pts',(91.1142006037765,0.129579708798338,-2.20022502915049));
#16082=CARTESIAN_POINT('Ctrl Pts',(91.1127941258068,0.10348776321749,-2.2016091044885));
#16083=CARTESIAN_POINT('Ctrl Pts',(91.1120830330832,0.0902198379230107,
-2.202192715812));
#16084=CARTESIAN_POINT('Ctrl Pts',(91.1103197421546,0.0571356243412686,
-2.20334847441452));
#16085=CARTESIAN_POINT('Ctrl Pts',(91.1092721809343,0.0373151597815744,
-2.20377326244858));
#16086=CARTESIAN_POINT('Ctrl Pts',(91.1051597604413,-0.0411051475227443,
-2.20439563534501));
#16087=CARTESIAN_POINT('Ctrl Pts',(91.1021591586453,-0.0996994388175074,
-2.20252367159185));
#16088=CARTESIAN_POINT('Ctrl Pts',(91.0941803563011,-0.258039267611667,
-2.19113227467141));
#16089=CARTESIAN_POINT('Ctrl Pts',(91.0893220315997,-0.357323449568237,
-2.17714639031626));
#16090=CARTESIAN_POINT('Ctrl Pts',(91.077652638277,-0.593504242587038,-2.12727907218789));
#16091=CARTESIAN_POINT('Ctrl Pts',(91.07089026408,-0.728553107449761,-2.08488961658958));
#16092=CARTESIAN_POINT('Ctrl Pts',(91.0624947438596,-0.876660070092227,
-2.02224320879027));
#16093=CARTESIAN_POINT('Ctrl Pts',(91.0614594181588,-0.894615674425303,
-2.01436422145357));
#16094=CARTESIAN_POINT('Ctrl Pts',(91.0599201315754,-0.920805593069546,
-2.0024527590993));
#16095=CARTESIAN_POINT('Ctrl Pts',(91.0594268475946,-0.929124142751027,
-1.99860659309374));
#16096=CARTESIAN_POINT('Ctrl Pts',(91.0585462936461,-0.943835430528812,
-1.99169298692826));
#16097=CARTESIAN_POINT('Ctrl Pts',(91.0581602939695,-0.950237685206415,
-1.98864642759259));
#16098=CARTESIAN_POINT('Ctrl Pts',(91.0573099592901,-0.964238339005941,
-1.98190106652062));
#16099=CARTESIAN_POINT('Ctrl Pts',(91.0568448713887,-0.97183010081582,-1.97818949096239));
#16100=CARTESIAN_POINT('Ctrl Pts',(91.0554912421186,-0.993743049685785,
-1.96731977234564));
#16101=CARTESIAN_POINT('Ctrl Pts',(91.0545961614286,-1.00800752955069,-1.96004926605665));
#16102=CARTESIAN_POINT('Ctrl Pts',(91.0525252856672,-1.0405336461502,-1.94302197192162));
#16103=CARTESIAN_POINT('Ctrl Pts',(91.0513442365129,-1.05873938360277,-1.93316205039062));
#16104=CARTESIAN_POINT('Ctrl Pts',(91.047314576823,-1.11980957672644,-1.89896603481867));
#16105=CARTESIAN_POINT('Ctrl Pts',(91.0444165918693,-1.16199416767576,-1.87344990124736));
#16106=CARTESIAN_POINT('Ctrl Pts',(91.0358744265014,-1.28243541750431,-1.79496527203492));
#16107=CARTESIAN_POINT('Ctrl Pts',(91.0301610603921,-1.35818659783151,-1.73835268346984));
#16108=CARTESIAN_POINT('Ctrl Pts',(91.0166397242476,-1.53026215195349,-1.59161903700953));
#16109=CARTESIAN_POINT('Ctrl Pts',(91.0089325982786,-1.62260729679554,-1.49736706598294));
#16110=CARTESIAN_POINT('Ctrl Pts',(91.0002374767894,-1.72142699463182,-1.37655338591616));
#16111=CARTESIAN_POINT('Ctrl Pts',(90.9988920432473,-1.73654568698149,-1.357431127749));
#16112=CARTESIAN_POINT('Ctrl Pts',(90.9967730952672,-1.76007287796891,-1.32663716327648));
#16113=CARTESIAN_POINT('Ctrl Pts',(90.9959914118325,-1.76868940103444,-1.31512756613624));
#16114=CARTESIAN_POINT('Ctrl Pts',(90.9945396947139,-1.78457104247931,-1.29347509431724));
#16115=CARTESIAN_POINT('Ctrl Pts',(90.9938686005316,-1.79186381548404,-1.28335330323643));
#16116=CARTESIAN_POINT('Ctrl Pts',(90.9923620777023,-1.80812133866769,-1.26038038655201));
#16117=CARTESIAN_POINT('Ctrl Pts',(90.9915285951134,-1.81703582701421,-1.24749441469915));
#16118=CARTESIAN_POINT('Ctrl Pts',(90.9890429038808,-1.84337072472549,-1.20854583191193));
#16119=CARTESIAN_POINT('Ctrl Pts',(90.9874063314547,-1.86037365650784,-1.18220499231589));
#16120=CARTESIAN_POINT('Ctrl Pts',(90.983671473719,-1.89831876705991,-1.12057352732373));
#16121=CARTESIAN_POINT('Ctrl Pts',(90.9815874536804,-1.91884909186674,-1.08504266262503));
#16122=CARTESIAN_POINT('Ctrl Pts',(90.9741115088847,-1.9897974032026,-0.953936813325641));
#16123=CARTESIAN_POINT('Ctrl Pts',(90.9688947326589,-2.03416360030641,-0.85525970787352));
#16124=CARTESIAN_POINT('Ctrl Pts',(90.9574430381797,-2.11519846482341,-0.632588915433794));
#16125=CARTESIAN_POINT('Ctrl Pts',(90.9512277224984,-2.14856530016115,-0.507831853855941));
#16126=CARTESIAN_POINT('Ctrl Pts',(90.9434490079919,-2.17434623604072,-0.360896830609277));
#16127=CARTESIAN_POINT('Ctrl Pts',(90.9423781358766,-2.17757786439909,-0.340855780621291));
#16128=CARTESIAN_POINT('Ctrl Pts',(90.9408012221957,-2.18186962429036,-0.311681564952728));
#16129=CARTESIAN_POINT('Ctrl Pts',(90.9403068029366,-2.18315024161461,-0.302581347376627));
#16130=CARTESIAN_POINT('Ctrl Pts',(90.9394244442498,-2.18532003665806,-0.286431191430478));
#16131=CARTESIAN_POINT('Ctrl Pts',(90.9390377841379,-2.18623208691783,-0.279384592817169));
#16132=CARTESIAN_POINT('Ctrl Pts',(90.9381938896706,-2.18813860883047,-0.264073317979917));
#16133=CARTESIAN_POINT('Ctrl Pts',(90.9377359914222,-2.18912032717815,-0.255807500258446));
#16134=CARTESIAN_POINT('Ctrl Pts',(90.936424766465,-2.19178298283505,-0.23224990874765));
#16135=CARTESIAN_POINT('Ctrl Pts',(90.935565504482,-2.19335063733117,-0.216946118943796));
#16136=CARTESIAN_POINT('Ctrl Pts',(90.9282071839857,-2.20529881230776,-0.0868877893682897));
#16137=CARTESIAN_POINT('Ctrl Pts',(90.9213189656286,-2.20682480008865,0.0284918618030112));
#16138=CARTESIAN_POINT('Ctrl Pts',(90.9039493902481,-2.18800114639563,0.317090697263738));
#16139=CARTESIAN_POINT('Ctrl Pts',(90.8935353510432,-2.15614915948067,0.48881034344095));
#16140=CARTESIAN_POINT('Ctrl Pts',(90.8822945800032,-2.09654469719752,0.680307456604186));
#16141=CARTESIAN_POINT('Ctrl Pts',(90.8808241811362,-2.08821535415084,0.705460575616805));
#16142=CARTESIAN_POINT('Ctrl Pts',(90.8784747258084,-2.0740418983742,0.745808906767966));
#16143=CARTESIAN_POINT('Ctrl Pts',(90.8775865117799,-2.06847962883379,0.761099708810144));
#16144=CARTESIAN_POINT('Ctrl Pts',(90.8760170498827,-2.05828814459545,0.788179079006374));
#16145=CARTESIAN_POINT('Ctrl Pts',(90.8753336121017,-2.05372573383445,0.799991853889391));
#16146=CARTESIAN_POINT('Ctrl Pts',(90.8738977487521,-2.04387793751207,0.82484972110277));
#16147=CARTESIAN_POINT('Ctrl Pts',(90.8731461568559,-2.03856887516801,0.837884860599564));
#16148=CARTESIAN_POINT('Ctrl Pts',(90.8711480228918,-2.02404337323315,0.872593292053562));
#16149=CARTESIAN_POINT('Ctrl Pts',(90.869909075878,-2.01460367768383,0.894171520629218));
#16150=CARTESIAN_POINT('Ctrl Pts',(90.8631477842513,-1.96072913298534,1.01213717464));
#16151=CARTESIAN_POINT('Ctrl Pts',(90.8578572638919,-1.90972078764351,1.10537336309242));
#16152=CARTESIAN_POINT('Ctrl Pts',(90.8456971390052,-1.77478695955714,1.31458741267225));
#16153=CARTESIAN_POINT('Ctrl Pts',(90.8389496611619,-1.6859119404452,1.42678145541832));
#16154=CARTESIAN_POINT('Ctrl Pts',(90.8291431705938,-1.54989704771596,1.56788556714735));
#16155=CARTESIAN_POINT('Ctrl Pts',(90.8264267835324,-1.51160551479694,1.60483455939629));
#16156=CARTESIAN_POINT('Ctrl Pts',(90.8228950905254,-1.46185338111679,1.64948089127736));
#16157=CARTESIAN_POINT('Ctrl Pts',(90.8221674408116,-1.45160451634587,1.65850740966788));
#16158=CARTESIAN_POINT('Ctrl Pts',(90.8210050416147,-1.43525221602499,1.67264174370351));
#16159=CARTESIAN_POINT('Ctrl Pts',(90.820574782883,-1.42920370277016,1.67781289132827));
#16160=CARTESIAN_POINT('Ctrl Pts',(90.8197494982183,-1.41761411565941,1.68761321130275));
#16161=CARTESIAN_POINT('Ctrl Pts',(90.8193548882596,-1.41207812640553,1.69224805842509));
#16162=CARTESIAN_POINT('Ctrl Pts',(90.8184047061873,-1.39875896122519,1.70328828323127));
#16163=CARTESIAN_POINT('Ctrl Pts',(90.8178473172664,-1.39095446286669,1.70966759388672));
#16164=CARTESIAN_POINT('Ctrl Pts',(90.8159054535254,-1.36378288602652,1.73156814236291));
#16165=CARTESIAN_POINT('Ctrl Pts',(90.8145035517347,-1.34419823472349,1.74681509965974));
#16166=CARTESIAN_POINT('Ctrl Pts',(90.810969646717,-1.2947845923879,1.78396131659869));
#16167=CARTESIAN_POINT('Ctrl Pts',(90.8088176930298,-1.26465413705216,1.80544586634922));
#16168=CARTESIAN_POINT('Ctrl Pts',(90.8016372987192,-1.16348612427445,1.87380852034797));
#16169=CARTESIAN_POINT('Ctrl Pts',(90.7965151083704,-1.09027514932016,1.91733085295948));
#16170=CARTESIAN_POINT('Ctrl Pts',(90.7851061102643,-0.921540553026482,
2.00484417933294));
#16171=CARTESIAN_POINT('Ctrl Pts',(90.7788449753409,-0.825006131776845,
2.0464616730939));
#16172=CARTESIAN_POINT('Ctrl Pts',(90.7691859279851,-0.667240068742853,
2.10149039191718));
#16173=CARTESIAN_POINT('Ctrl Pts',(90.7656656586162,-0.607772480574641,
2.11945390409258));
#16174=CARTESIAN_POINT('Ctrl Pts',(90.7610708726807,-0.527427312167493,
2.14006333019295));
#16175=CARTESIAN_POINT('Ctrl Pts',(90.7599251863802,-0.507160438180113,
2.14495663334007));
#16176=CARTESIAN_POINT('Ctrl Pts',(90.7580523622403,-0.473652088144785,
2.15254550985492));
#16177=CARTESIAN_POINT('Ctrl Pts',(90.7573199193736,-0.460450145187544,
2.15540811629268));
#16178=CARTESIAN_POINT('Ctrl Pts',(90.7558963198507,-0.434603938493177,
2.16076409692801));
#16179=CARTESIAN_POINT('Ctrl Pts',(90.7552048430207,-0.421962498429916,
2.16326829717963));
#16180=CARTESIAN_POINT('Ctrl Pts',(90.7538373225898,-0.396792261417112,
2.16802535117414));
#16181=CARTESIAN_POINT('Ctrl Pts',(90.7531612201785,-0.384264475209838,
2.17028082153423));
#16182=CARTESIAN_POINT('Ctrl Pts',(90.7515843459321,-0.354855740132947,
2.17531286319527));
#16183=CARTESIAN_POINT('Ctrl Pts',(90.7506863348501,-0.337960493038073,
2.17800169322356));
#16184=CARTESIAN_POINT('Ctrl Pts',(90.7478362013182,-0.283891309002596,
2.18596233051483));
#16185=CARTESIAN_POINT('Ctrl Pts',(90.7459069744405,-0.246612401598594,
2.19048125144737));
#16186=CARTESIAN_POINT('Ctrl Pts',(90.7404580552706,-0.139689516270678,
2.20067793500518));
#16187=CARTESIAN_POINT('Ctrl Pts',(90.7370029463319,-0.0698659755842112,
2.20399999999936));
#16188=CARTESIAN_POINT('Ctrl Pts',(90.7335918111184,-2.00577712042713E-11,
2.204));
#16189=CARTESIAN_POINT('Ctrl Pts',(90.6267804315841,0.00190491555487048,
2.2039991767913));
#16190=CARTESIAN_POINT('Ctrl Pts',(90.6326452887204,-0.097354835602562,
2.20408496695218));
#16191=CARTESIAN_POINT('Ctrl Pts',(90.6383718140951,-0.196518494825245,
2.1974653855676));
#16192=CARTESIAN_POINT('Ctrl Pts',(90.6448581573574,-0.312104610835634,
2.18185877429554));
#16193=CARTESIAN_POINT('Ctrl Pts',(90.6458167394167,-0.329270238770531,
2.17933433254394));
#16194=CARTESIAN_POINT('Ctrl Pts',(90.6474799876175,-0.359196947643492,
2.17457153049561));
#16195=CARTESIAN_POINT('Ctrl Pts',(90.6481874099946,-0.371971262077163,
2.17242288208958));
#16196=CARTESIAN_POINT('Ctrl Pts',(90.6496052293846,-0.397662593043945,
2.16786832508738));
#16197=CARTESIAN_POINT('Ctrl Pts',(90.650315496025,-0.410578522180935,2.16545928159995));
#16198=CARTESIAN_POINT('Ctrl Pts',(90.6517668489606,-0.437060214173424,
2.16027453739834));
#16199=CARTESIAN_POINT('Ctrl Pts',(90.6525075026649,-0.450622925502529,
2.15748619893469));
#16200=CARTESIAN_POINT('Ctrl Pts',(90.6543902654078,-0.485215726762072,
2.15003387790102));
#16201=CARTESIAN_POINT('Ctrl Pts',(90.6555266485398,-0.506205604615391,
2.14518901410195));
#16202=CARTESIAN_POINT('Ctrl Pts',(90.6601228410488,-0.591489096895206,
2.12418247666762));
#16203=CARTESIAN_POINT('Ctrl Pts',(90.6635013051919,-0.655111537125245,
2.10543117425174));
#16204=CARTESIAN_POINT('Ctrl Pts',(90.6736990886196,-0.847902868624687,
2.03902257270528));
#16205=CARTESIAN_POINT('Ctrl Pts',(90.6802701331931,-0.973523772099443,
1.98212107221013));
#16206=CARTESIAN_POINT('Ctrl Pts',(90.6900878577459,-1.14759248575074,1.88271003564006));
#16207=CARTESIAN_POINT('Ctrl Pts',(90.6932003776977,-1.20080476257532,1.84922488380863));
#16208=CARTESIAN_POINT('Ctrl Pts',(90.6982425140115,-1.28206240381173,1.79310397851002));
#16209=CARTESIAN_POINT('Ctrl Pts',(90.7001069248905,-1.31110941621345,1.77197565120365));
#16210=CARTESIAN_POINT('Ctrl Pts',(90.7026401304206,-1.34898454831256,1.74298467995302));
#16211=CARTESIAN_POINT('Ctrl Pts',(90.7032706556186,-1.35828561576675,1.73574626027305));
#16212=CARTESIAN_POINT('Ctrl Pts',(90.7043219638285,-1.37357445775793,1.72364980638154));
#16213=CARTESIAN_POINT('Ctrl Pts',(90.7047398743952,-1.37959569978158,1.71883424084938));
#16214=CARTESIAN_POINT('Ctrl Pts',(90.7055296706781,-1.39086602157835,1.70972328535681));
#16215=CARTESIAN_POINT('Ctrl Pts',(90.7059010528884,-1.39612074071251,1.70543509862382));
#16216=CARTESIAN_POINT('Ctrl Pts',(90.7067892588485,-1.40858398209242,1.69516809648338));
#16217=CARTESIAN_POINT('Ctrl Pts',(90.7073075950979,-1.41577432858068,1.68916747366788));
#16218=CARTESIAN_POINT('Ctrl Pts',(90.7091663352259,-1.44127441965073,1.66760946458652));
#16219=CARTESIAN_POINT('Ctrl Pts',(90.7105231696652,-1.45936714238669,1.65179923960171));
#16220=CARTESIAN_POINT('Ctrl Pts',(90.7223111948723,-1.612499732264,1.51350529212859));
#16221=CARTESIAN_POINT('Ctrl Pts',(90.7335208730586,-1.73211619815348,1.3750012234323));
#16222=CARTESIAN_POINT('Ctrl Pts',(90.7483127503244,-1.87096932705395,1.1669158449815));
#16223=CARTESIAN_POINT('Ctrl Pts',(90.7522658411997,-1.90600311809421,1.10877053820822));
#16224=CARTESIAN_POINT('Ctrl Pts',(90.7587239305597,-1.95994971842568,1.00909941843466));
#16225=CARTESIAN_POINT('Ctrl Pts',(90.7612755175112,-1.98035635047836,0.968438788152192));
#16226=CARTESIAN_POINT('Ctrl Pts',(90.7647905812224,-2.00716980563328,0.91061437450783));
#16227=CARTESIAN_POINT('Ctrl Pts',(90.7657901551802,-2.01464253676964,0.893960091324293));
#16228=CARTESIAN_POINT('Ctrl Pts',(90.7674961362505,-2.02712992069623,0.865177693913809));
#16229=CARTESIAN_POINT('Ctrl Pts',(90.7682059117345,-2.03224464934016,0.853094281436316));
#16230=CARTESIAN_POINT('Ctrl Pts',(90.7696440661534,-2.0424412542888,0.828392863272744));
#16231=CARTESIAN_POINT('Ctrl Pts',(90.7703721421267,-2.04751483784413,0.815772035130639));
#16232=CARTESIAN_POINT('Ctrl Pts',(90.7721981913294,-2.06001226370632,0.783832733050363));
#16233=CARTESIAN_POINT('Ctrl Pts',(90.7732909856817,-2.06728153564264,0.764454950266328));
#16234=CARTESIAN_POINT('Ctrl Pts',(90.777470796035,-2.09425117041366,0.689362059110674));
#16235=CARTESIAN_POINT('Ctrl Pts',(90.7804935068911,-2.11198151125229,0.632963562196727));
#16236=CARTESIAN_POINT('Ctrl Pts',(90.7918592134606,-2.1711293676271,0.414472775958202));
#16237=CARTESIAN_POINT('Ctrl Pts',(90.799732922515,-2.19631362398695,0.248586787085156));
#16238=CARTESIAN_POINT('Ctrl Pts',(90.8116022011743,-2.20524988113747,0.00694075432550717));
#16239=CARTESIAN_POINT('Ctrl Pts',(90.8153291748321,-2.20422236917874,-0.0676543622756929));
#16240=CARTESIAN_POINT('Ctrl Pts',(90.820204932275,-2.19821483892035,-0.160673280659657));
#16241=CARTESIAN_POINT('Ctrl Pts',(90.8211919102693,-2.19677536628233,-0.179282809545848));
#16242=CARTESIAN_POINT('Ctrl Pts',(90.822676060121,-2.19428689507821,-0.206888861870636));
#16243=CARTESIAN_POINT('Ctrl Pts',(90.8231637612441,-2.193418476558,-0.21590127357763));
#16244=CARTESIAN_POINT('Ctrl Pts',(90.8240047594265,-2.1918353102133,-0.231334628047367));
#16245=CARTESIAN_POINT('Ctrl Pts',(90.8243565367105,-2.19114782417496,-0.237758173441339));
#16246=CARTESIAN_POINT('Ctrl Pts',(90.8251686573448,-2.1895030780557,-0.252512546137206));
#16247=CARTESIAN_POINT('Ctrl Pts',(90.8256300500338,-2.18852653273285,-0.260840804905782));
#16248=CARTESIAN_POINT('Ctrl Pts',(90.8269304385665,-2.18565606088373,-0.284169274921833));
#16249=CARTESIAN_POINT('Ctrl Pts',(90.8277750649536,-2.18365530735656,-0.299155588367893));
#16250=CARTESIAN_POINT('Ctrl Pts',(90.8337066694941,-2.16865111886528,-0.40335677729367));
#16251=CARTESIAN_POINT('Ctrl Pts',(90.8390341673297,-2.15033931463097,-0.491713499498828));
#16252=CARTESIAN_POINT('Ctrl Pts',(90.8460251251684,-2.11965781886437,-0.604466953568136));
#16253=CARTESIAN_POINT('Ctrl Pts',(90.847628728038,-2.11217605699912,-0.630112569026625));
#16254=CARTESIAN_POINT('Ctrl Pts',(90.8549531641175,-2.07591641924759,-0.746489627894509));
#16255=CARTESIAN_POINT('Ctrl Pts',(90.8606783571139,-2.04174430628093,-0.835438591472057));
#16256=CARTESIAN_POINT('Ctrl Pts',(90.8697480836424,-1.97722188880606,-0.9755500975986));
#16257=CARTESIAN_POINT('Ctrl Pts',(90.8731693244949,-1.95036905128488,-1.02818567684173));
#16258=CARTESIAN_POINT('Ctrl Pts',(90.8788587876251,-1.90127298599547,-1.11555839638947));
#16259=CARTESIAN_POINT('Ctrl Pts',(90.8811610981769,-1.88011189162641,-1.15086450102903));
#16260=CARTESIAN_POINT('Ctrl Pts',(90.8843889066163,-1.84858353197804,-1.20027482218747));
#16261=CARTESIAN_POINT('Ctrl Pts',(90.8853437065736,-1.83901887259552,-1.21487873247678));
#16262=CARTESIAN_POINT('Ctrl Pts',(90.8869910068826,-1.82210372056902,-1.24004823475346));
#16263=CARTESIAN_POINT('Ctrl Pts',(90.8876864526316,-1.81483241762171,-1.25066578223748));
#16264=CARTESIAN_POINT('Ctrl Pts',(90.8891110388561,-1.7996705880225,-1.27239438292187));
#16265=CARTESIAN_POINT('Ctrl Pts',(90.8898397186364,-1.79176915487626,-1.28349717500584));
#16266=CARTESIAN_POINT('Ctrl Pts',(90.8916982398836,-1.77124429211631,-1.31177897881817));
#16267=CARTESIAN_POINT('Ctrl Pts',(90.8928223010737,-1.75847352556479,-1.32884962806599));
#16268=CARTESIAN_POINT('Ctrl Pts',(90.897390751715,-1.70513258025483,-1.3980344772883));
#16269=CARTESIAN_POINT('Ctrl Pts',(90.9007520663101,-1.662476028188,-1.44849991739415));
#16270=CARTESIAN_POINT('Ctrl Pts',(90.9113478275123,-1.51823294946866,-1.60436720373089));
#16271=CARTESIAN_POINT('Ctrl Pts',(90.918274116129,-1.4084076441104,-1.70159141246577));
#16272=CARTESIAN_POINT('Ctrl Pts',(90.9295646703694,-1.22053561938693,-1.83717063328024));
#16273=CARTESIAN_POINT('Ctrl Pts',(90.9337921035136,-1.14847574208645,-1.88305708896934));
#16274=CARTESIAN_POINT('Ctrl Pts',(90.9392781374331,-1.05664770789302,-1.93429675607218));
#16275=CARTESIAN_POINT('Ctrl Pts',(90.9403234251668,-1.03922245985327,-1.94371421349969));
#16276=CARTESIAN_POINT('Ctrl Pts',(90.9418757017544,-1.01350635399328,-1.95716780680309));
#16277=CARTESIAN_POINT('Ctrl Pts',(90.9423716932234,-1.00531286402195,-1.96138904677404));
#16278=CARTESIAN_POINT('Ctrl Pts',(90.9432206655296,-0.991334661380445,
-1.9684799426538));
#16279=CARTESIAN_POINT('Ctrl Pts',(90.9435720039391,-0.9855634532424,-1.97137575657455));
#16280=CARTESIAN_POINT('Ctrl Pts',(90.9443756280446,-0.972394512590901,
-1.97791124217561));
#16281=CARTESIAN_POINT('Ctrl Pts',(90.9448288771926,-0.964989163385836,
-1.98153472844662));
#16282=CARTESIAN_POINT('Ctrl Pts',(90.9460796873697,-0.94460709583906,-1.99136645848665));
#16283=CARTESIAN_POINT('Ctrl Pts',(90.9468821940927,-0.931589874775223,
-1.99748922909619));
#16284=CARTESIAN_POINT('Ctrl Pts',(90.9514426694677,-0.857885541462968,
-2.03127959817955));
#16285=CARTESIAN_POINT('Ctrl Pts',(90.9553322177099,-0.796031421974158,
-2.05630661342561));
#16286=CARTESIAN_POINT('Ctrl Pts',(90.9672467057016,-0.606435894172123,
-2.12318249433125));
#16287=CARTESIAN_POINT('Ctrl Pts',(90.9754203389746,-0.475905545911,-2.15619679018695));
#16288=CARTESIAN_POINT('Ctrl Pts',(90.9872968001492,-0.27743766252443,-2.18748104812074));
#16289=CARTESIAN_POINT('Ctrl Pts',(90.9911722597462,-0.211259320734743,
-2.19486118639416));
#16290=CARTESIAN_POINT('Ctrl Pts',(90.9975196444823,-0.100062030757739,
-2.20218475922974));
#16291=CARTESIAN_POINT('Ctrl Pts',(91.0000364675163,-0.055198358905565,
-2.20376579462566));
#16292=CARTESIAN_POINT('Ctrl Pts',(91.003510271349,0.0078082011853508,-2.20406068409168));
#16293=CARTESIAN_POINT('Ctrl Pts',(91.0045025148874,0.025932387546345,-2.20392196007757));
#16294=CARTESIAN_POINT('Ctrl Pts',(91.0061978414517,0.057112169692719,-2.20329861913878));
#16295=CARTESIAN_POINT('Ctrl Pts',(91.0069042413448,0.0701687573921278,
-2.2029214604185));
#16296=CARTESIAN_POINT('Ctrl Pts',(91.0082507787625,0.0951775988744194,
-2.20197647102864));
#16297=CARTESIAN_POINT('Ctrl Pts',(91.0088914750374,0.10713005681573,-2.20142733538414));
#16298=CARTESIAN_POINT('Ctrl Pts',(91.0103941129953,0.135282831295993,-2.19990407367748));
#16299=CARTESIAN_POINT('Ctrl Pts',(91.0112534836594,0.15147814608499,-2.19884828214841));
#16300=CARTESIAN_POINT('Ctrl Pts',(91.0142659503734,0.208562368717168,-2.19449320548174));
#16301=CARTESIAN_POINT('Ctrl Pts',(91.0163892343322,0.249370524910688,-2.19023133656061));
#16302=CARTESIAN_POINT('Ctrl Pts',(91.0270571261946,0.456637633807952,-2.1627165156347));
#16303=CARTESIAN_POINT('Ctrl Pts',(91.0350371392582,0.620156215127857,-2.12161940768778));
#16304=CARTESIAN_POINT('Ctrl Pts',(91.0477251057285,0.864146046090899,-2.02964470209689));
#16305=CARTESIAN_POINT('Ctrl Pts',(91.0522951794113,0.948715145275712,-1.99151762594507));
#16306=CARTESIAN_POINT('Ctrl Pts',(91.058200292359,1.0488651162554,-1.9385365037729));
#16307=CARTESIAN_POINT('Ctrl Pts',(91.0592884506128,1.06696810949395,-1.92863184708703));
#16308=CARTESIAN_POINT('Ctrl Pts',(91.060895556087,1.09313346633649,-1.91383491231301));
#16309=CARTESIAN_POINT('Ctrl Pts',(91.0614026145291,1.10130821736325,-1.9091424909212));
#16310=CARTESIAN_POINT('Ctrl Pts',(91.0622990709095,1.11561278366581,-1.90080902412767));
#16311=CARTESIAN_POINT('Ctrl Pts',(91.0626870410073,1.12175539713343,-1.89719046407876));
#16312=CARTESIAN_POINT('Ctrl Pts',(91.0635385486055,1.13513050978949,-1.8892236333736));
#16313=CARTESIAN_POINT('Ctrl Pts',(91.0640028078407,1.14235551495216,-1.88486367776403));
#16314=CARTESIAN_POINT('Ctrl Pts',(91.0653120018854,1.16254812396673,-1.8725196297723));
#16315=CARTESIAN_POINT('Ctrl Pts',(91.0661626198847,1.17545803549536,-1.86444262044296));
#16316=CARTESIAN_POINT('Ctrl Pts',(91.0722839155968,1.2669686416195,-1.80586134344359));
#16317=CARTESIAN_POINT('Ctrl Pts',(91.0778110851321,1.34236502443718,-1.75054209312594));
#16318=CARTESIAN_POINT('Ctrl Pts',(91.0889673667062,1.48536270543473,-1.63093983715516));
#16319=CARTESIAN_POINT('Ctrl Pts',(91.0945841385624,1.55286170479341,-1.56680835157321));
#16320=CARTESIAN_POINT('Ctrl Pts',(91.1067517796543,1.69214083235893,-1.41660852205035));
#16321=CARTESIAN_POINT('Ctrl Pts',(91.1132400255126,1.76183159901642,-1.32893772933579));
#16322=CARTESIAN_POINT('Ctrl Pts',(91.1207978931841,1.8380119167621,-1.21651226797715));
#16323=CARTESIAN_POINT('Ctrl Pts',(91.1221190854593,1.85112643173024,-1.19646182638423));
#16324=CARTESIAN_POINT('Ctrl Pts',(91.1242068108453,1.8715173042875,-1.16414865101554));
#16325=CARTESIAN_POINT('Ctrl Pts',(91.1249811548772,1.87900583413761,-1.15202265194626));
#16326=CARTESIAN_POINT('Ctrl Pts',(91.1264419361295,1.89298804266924,-1.12888250746689));
#16327=CARTESIAN_POINT('Ctrl Pts',(91.1271291881392,1.89950449814457,-1.11788287241177));
#16328=CARTESIAN_POINT('Ctrl Pts',(91.1286889668436,1.91414982215423,-1.09266403616065));
#16329=CARTESIAN_POINT('Ctrl Pts',(91.1295592303648,1.92221669237956,-1.07840959040759));
#16330=CARTESIAN_POINT('Ctrl Pts',(91.1318270318326,1.94295437362976,-1.04079323280673));
#16331=CARTESIAN_POINT('Ctrl Pts',(91.1332153083493,1.95536302511075,-1.01728942309624));
#16332=CARTESIAN_POINT('Ctrl Pts',(91.1450917469282,2.05887571486137,-0.812325678814625));
#16333=CARTESIAN_POINT('Ctrl Pts',(91.1546202630543,2.12491977230903,-0.619320684074938));
#16334=CARTESIAN_POINT('Ctrl Pts',(91.1674443760715,2.17487539091969,-0.361975956396143));
#16335=CARTESIAN_POINT('Ctrl Pts',(91.1703735351449,2.18379959145835,-0.303526171115663));
#16336=CARTESIAN_POINT('Ctrl Pts',(91.1751521196547,2.19419072316193,-0.210547809353404));
#16337=CARTESIAN_POINT('Ctrl Pts',(91.1769419170975,2.1972140151268,-0.176220397250195));
#16338=CARTESIAN_POINT('Ctrl Pts',(91.1793810230299,2.20016862701943,-0.130404325849278));
#16339=CARTESIAN_POINT('Ctrl Pts',(91.1799941767993,2.20081679071618,-0.118965195789882));
#16340=CARTESIAN_POINT('Ctrl Pts',(91.181017919216,2.20174267312989,-0.100008896740413));
#16341=CARTESIAN_POINT('Ctrl Pts',(91.1814257407627,2.20207115751675,-0.0924942825992905));
#16342=CARTESIAN_POINT('Ctrl Pts',(91.1822008422639,2.20261938775447,-0.0782859268993837));
#16343=CARTESIAN_POINT('Ctrl Pts',(91.1825676591037,2.20284710209822,-0.0715925691408228));
#16344=CARTESIAN_POINT('Ctrl Pts',(91.1834452175826,2.20331676375726,-0.0556494040281865));
#16345=CARTESIAN_POINT('Ctrl Pts',(91.1839574520496,2.20353097234369,-0.0463989798159462));
#16346=CARTESIAN_POINT('Ctrl Pts',(91.1855246181047,2.20400538663348,-0.0182555968829399));
#16347=CARTESIAN_POINT('Ctrl Pts',(91.1865887633008,2.2040808866569,0.000639150944144555));
#16348=CARTESIAN_POINT('Ctrl Pts',(91.1939716982295,2.202930395477,0.130456778283692));
#16349=CARTESIAN_POINT('Ctrl Pts',(91.2006180440115,2.19357438941952,0.241140712553303));
#16350=CARTESIAN_POINT('Ctrl Pts',(91.2134217847883,2.15966681699686,0.451557317539482));
#16351=CARTESIAN_POINT('Ctrl Pts',(91.2195612596613,2.13640254015311,0.551227138726623));
#16352=CARTESIAN_POINT('Ctrl Pts',(91.2302309579572,2.08269194356501,0.725562396785453));
#16353=CARTESIAN_POINT('Ctrl Pts',(91.2348167695877,2.0549147549709,0.800858362059234));
#16354=CARTESIAN_POINT('Ctrl Pts',(91.2404910108436,2.01434811643794,0.894708518273887));
#16355=CARTESIAN_POINT('Ctrl Pts',(91.241703818383,2.00530104858002,0.914805674071664));
#16356=CARTESIAN_POINT('Ctrl Pts',(91.2436608237272,1.99008890385953,0.947287379801753));
#16357=CARTESIAN_POINT('Ctrl Pts',(91.2444112336959,1.98410615045209,0.959755188154415));
#16358=CARTESIAN_POINT('Ctrl Pts',(91.2458528865144,1.97232365401225,0.983728307146277));
#16359=CARTESIAN_POINT('Ctrl Pts',(91.2465446382939,1.96653960351286,0.995240662371494));
#16360=CARTESIAN_POINT('Ctrl Pts',(91.2481363840608,1.95292968726279,1.02174736777968));
#16361=CARTESIAN_POINT('Ctrl Pts',(91.2490337878753,1.94503145297032,1.0367037741863));
#16362=CARTESIAN_POINT('Ctrl Pts',(91.2519634877876,1.91851244514409,1.08555111325186));
#16363=CARTESIAN_POINT('Ctrl Pts',(91.2539702043777,1.89917142430908,1.1190439482456));
#16364=CARTESIAN_POINT('Ctrl Pts',(91.264761568948,1.78896361845481,1.29879545029872));
#16365=CARTESIAN_POINT('Ctrl Pts',(91.2729318478896,1.68208320932294,1.43452394000362));
#16366=CARTESIAN_POINT('Ctrl Pts',(91.2858770212533,1.49398320987748,1.62311417647994));
#16367=CARTESIAN_POINT('Ctrl Pts',(91.2905137884267,1.42327640239945,1.68545734946492));
#16368=CARTESIAN_POINT('Ctrl Pts',(91.296501040871,1.33238898008588,1.75578660022845));
#16369=CARTESIAN_POINT('Ctrl Pts',(91.297595493826,1.31579233430909,1.76825831008208));
#16370=CARTESIAN_POINT('Ctrl Pts',(91.2992090931374,1.29140764741413,1.78604903129823));
#16371=CARTESIAN_POINT('Ctrl Pts',(91.2997161207993,1.28375727116081,1.79155578092814));
#16372=CARTESIAN_POINT('Ctrl Pts',(91.3006150435772,1.27022114846199,1.80116787872404));
#16373=CARTESIAN_POINT('Ctrl Pts',(91.3010055317506,1.26435034358085,1.8052937989297));
#16374=CARTESIAN_POINT('Ctrl Pts',(91.3018589264266,1.25154155048389,1.81420251155795));
#16375=CARTESIAN_POINT('Ctrl Pts',(91.3023225224186,1.24459634837588,1.81897414228444));
#16376=CARTESIAN_POINT('Ctrl Pts',(91.3036293407401,1.22504901590938,1.83223957684663));
#16377=CARTESIAN_POINT('Ctrl Pts',(91.3044782265253,1.21238638024956,1.84064287605444));
#16378=CARTESIAN_POINT('Ctrl Pts',(91.3105155569658,1.12248686899113,1.89897272355935));
#16379=CARTESIAN_POINT('Ctrl Pts',(91.3159529098435,1.04228466027102,1.94414858320991));
#16380=CARTESIAN_POINT('Ctrl Pts',(91.3227377034689,0.940192452085248,1.99351807562356));
#16381=CARTESIAN_POINT('Ctrl Pts',(91.3240244647457,0.920745314560739,2.00257439783287));
#16382=CARTESIAN_POINT('Ctrl Pts',(91.3305826079087,0.821072309124219,2.04723219089107));
#16383=CARTESIAN_POINT('Ctrl Pts',(91.3358644292024,0.738900107659062,2.07830390606254));
#16384=CARTESIAN_POINT('Ctrl Pts',(91.3449146092867,0.592604151018397,2.12384542922043));
#16385=CARTESIAN_POINT('Ctrl Pts',(91.3487228091861,0.52927763251353,2.14050586583685));
#16386=CARTESIAN_POINT('Ctrl Pts',(91.3549731701778,0.421965731992394,2.16368350628457));
#16387=CARTESIAN_POINT('Ctrl Pts',(91.3574585433306,0.378357675664242,2.17173369960022));
#16388=CARTESIAN_POINT('Ctrl Pts',(91.3608961712463,0.316719760133843,2.18119908054758));
#16389=CARTESIAN_POINT('Ctrl Pts',(91.3618827938221,0.298872150271845,2.1837161675648));
#16390=CARTESIAN_POINT('Ctrl Pts',(91.3635706694203,0.268073668796116,2.18767507532186));
#16391=CARTESIAN_POINT('Ctrl Pts',(91.3642751863364,0.255137388358216,2.18922147128726));
#16392=CARTESIAN_POINT('Ctrl Pts',(91.3656195439144,0.230300400161042,2.19196732798056));
#16393=CARTESIAN_POINT('Ctrl Pts',(91.3662599281512,0.21840218464924,2.19318479265922));
#16394=CARTESIAN_POINT('Ctrl Pts',(91.3679311333082,0.18718022466682,2.19612292635137));
#16395=CARTESIAN_POINT('Ctrl Pts',(91.3689569700343,0.167842418419153,2.19768544127829));
#16396=CARTESIAN_POINT('Ctrl Pts',(91.3725748857664,0.0990632065834146,
2.2023297297749));
#16397=CARTESIAN_POINT('Ctrl Pts',(91.3751232243473,0.0495399332369143,
2.204));
#16398=CARTESIAN_POINT('Ctrl Pts',(91.3776298668357,4.55134372080087E-12,
2.204));
#16399=CARTESIAN_POINT('Origin',(66.9212607628943,0.,0.));
#16400=CARTESIAN_POINT('',(92.2356508702176,-2.51612300885953E-11,2.204));
#16401=CARTESIAN_POINT('',(92.1243308360554,1.24847509279933E-11,2.204));
#16402=CARTESIAN_POINT('',(66.9212607628943,-2.69912154532077E-16,2.204));
#16403=CARTESIAN_POINT('Ctrl Pts',(92.2356508702176,-2.51603599066286E-11,
2.204));
#16404=CARTESIAN_POINT('Ctrl Pts',(92.2292589034109,0.108362820276164,2.20400000000124));
#16405=CARTESIAN_POINT('Ctrl Pts',(92.2226946757361,0.216577546288409,2.1960083774407));
#16406=CARTESIAN_POINT('Ctrl Pts',(92.2094793534317,0.435170017473937,2.16354518765205));
#16407=CARTESIAN_POINT('Ctrl Pts',(92.2028565183254,0.545153221931167,2.13848404676721));
#16408=CARTESIAN_POINT('Ctrl Pts',(92.1943936693437,0.688154827320078,2.09414254451766));
#16409=CARTESIAN_POINT('Ctrl Pts',(92.1923261000641,0.723278957464229,2.08227227989087));
#16410=CARTESIAN_POINT('Ctrl Pts',(92.1893675102199,0.773796971725582,2.06376697137654));
#16411=CARTESIAN_POINT('Ctrl Pts',(92.1884535116523,0.789439680567183,2.05783402589375));
#16412=CARTESIAN_POINT('Ctrl Pts',(92.1868552427004,0.816851609794035,2.04707868898289));
#16413=CARTESIAN_POINT('Ctrl Pts',(92.1861684893062,0.828649332558261,2.04233151188323));
#16414=CARTESIAN_POINT('Ctrl Pts',(92.1847417837419,0.853194852320118,2.03220715978855));
#16415=CARTESIAN_POINT('Ctrl Pts',(92.1840024937463,0.86593446000815,2.02681151547419));
#16416=CARTESIAN_POINT('Ctrl Pts',(92.1820737400488,0.899217268331408,2.01234405222682));
#16417=CARTESIAN_POINT('Ctrl Pts',(92.1808909526023,0.91967436673315,2.00307747940364));
#16418=CARTESIAN_POINT('Ctrl Pts',(92.1756329291041,1.01075067475344,1.96013263798239));
#16419=CARTESIAN_POINT('Ctrl Pts',(92.171676844361,1.07969131529775,1.92301980081122));
#16420=CARTESIAN_POINT('Ctrl Pts',(92.160912793194,1.26534000614474,1.80994133437855));
#16421=CARTESIAN_POINT('Ctrl Pts',(92.1543210805396,1.37703898871843,1.72648073941178));
#16422=CARTESIAN_POINT('Ctrl Pts',(92.1446812081425,1.52289466453686,1.5942835031326));
#16423=CARTESIAN_POINT('Ctrl Pts',(92.1418167677432,1.56412337990898,1.55385500366132));
#16424=CARTESIAN_POINT('Ctrl Pts',(92.1371358196637,1.62693705320157,1.48722487716522));
#16425=CARTESIAN_POINT('Ctrl Pts',(92.135376279173,1.64958691752246,1.46206182181309));
#16426=CARTESIAN_POINT('Ctrl Pts',(92.1329761841985,1.67902122393059,1.42780662433645));
#16427=CARTESIAN_POINT('Ctrl Pts',(92.132370540746,1.68632900262063,1.41916824612901));
#16428=CARTESIAN_POINT('Ctrl Pts',(92.1313587542599,1.69833158737897,1.40475662815667));
#16429=CARTESIAN_POINT('Ctrl Pts',(92.1309553043602,1.70306434595517,1.39901508063903));
#16430=CARTESIAN_POINT('Ctrl Pts',(92.1301880209674,1.71196211357715,1.38810869304045));
#16431=CARTESIAN_POINT('Ctrl Pts',(92.1298246374551,1.71613305115042,1.38294879527531));
#16432=CARTESIAN_POINT('Ctrl Pts',(92.1289552396416,1.72601196449929,1.37061400787798));
#16433=CARTESIAN_POINT('Ctrl Pts',(92.1284477592989,1.73169854804443,1.36342223571383));
#16434=CARTESIAN_POINT('Ctrl Pts',(92.126895317366,1.7488591753901,1.34143879155896));
#16435=CARTESIAN_POINT('Ctrl Pts',(92.1258413065812,1.76018950935915,1.32653657754112));
#16436=CARTESIAN_POINT('Ctrl Pts',(92.1186229649665,1.83574515312804,1.22448958767468));
#16437=CARTESIAN_POINT('Ctrl Pts',(92.1121455582501,1.8936595333111,1.13286577251837));
#16438=CARTESIAN_POINT('Ctrl Pts',(92.1000412918268,1.98851628772828,0.955051401001784));
#16439=CARTESIAN_POINT('Ctrl Pts',(92.0944317401465,2.02715958570171,0.870026308189507));
#16440=CARTESIAN_POINT('Ctrl Pts',(92.0836015185267,2.09254246197751,0.697942251155415));
#16441=CARTESIAN_POINT('Ctrl Pts',(92.0783846279476,2.11951464828223,0.611161350368453));
#16442=CARTESIAN_POINT('Ctrl Pts',(92.0720806754785,2.1464399985641,0.500924758781559));
#16443=CARTESIAN_POINT('Ctrl Pts',(92.0708316928622,2.15148067542277,0.478812321252053));
#16444=CARTESIAN_POINT('Ctrl Pts',(92.0688357689462,2.15905543247835,0.443044416788347));
#16445=CARTESIAN_POINT('Ctrl Pts',(92.0680820477926,2.16180322093066,0.429436330706117));
#16446=CARTESIAN_POINT('Ctrl Pts',(92.0666465314981,2.16681869998734,0.403328737558804));
#16447=CARTESIAN_POINT('Ctrl Pts',(92.0659640967017,2.16910724988882,0.390833848325662));
#16448=CARTESIAN_POINT('Ctrl Pts',(92.0644112576972,2.17409357221107,0.362215881542153));
#16449=CARTESIAN_POINT('Ctrl Pts',(92.0635431384464,2.17672026521733,0.346081077212601));
#16450=CARTESIAN_POINT('Ctrl Pts',(92.0612352638749,2.18326713039083,0.302837896303151));
#16451=CARTESIAN_POINT('Ctrl Pts',(92.0598057103574,2.18686196569118,0.275682758105604));
#16452=CARTESIAN_POINT('Ctrl Pts',(92.0499334775996,2.20840374751872,0.0858167061214575));
#16453=CARTESIAN_POINT('Ctrl Pts',(92.0420747003095,2.2086812416632,-0.0783817608894441));
#16454=CARTESIAN_POINT('Ctrl Pts',(92.0282231437749,2.17736107979107,-0.362965310556047));
#16455=CARTESIAN_POINT('Ctrl Pts',(92.0222638896055,2.15380762064295,-0.483477909052407));
#16456=CARTESIAN_POINT('Ctrl Pts',(92.0149784920738,2.11598575199715,-0.61682879972263));
#16457=CARTESIAN_POINT('Ctrl Pts',(92.0141269470507,2.11143908377422,-0.632217080300995));
#16458=CARTESIAN_POINT('Ctrl Pts',(92.0128121395605,2.10423867246123,-0.65564259924182));
#16459=CARTESIAN_POINT('Ctrl Pts',(92.0123555776976,2.10170588799374,-0.663716780081136));
#16460=CARTESIAN_POINT('Ctrl Pts',(92.0115113391599,2.096964992006,-0.67853085626438));
#16461=CARTESIAN_POINT('Ctrl Pts',(92.0111244620461,2.09477077347478,-0.685274910586024));
#16462=CARTESIAN_POINT('Ctrl Pts',(92.0102335584211,2.08966828156304,-0.700704190102408));
#16463=CARTESIAN_POINT('Ctrl Pts',(92.0097283035788,2.08673839860801,-0.709381941296212));
#16464=CARTESIAN_POINT('Ctrl Pts',(92.0081337137861,2.0773757097611,-0.736552458233469));
#16465=CARTESIAN_POINT('Ctrl Pts',(92.0070339834833,2.07075068137228,-0.754977433310458));
#16466=CARTESIAN_POINT('Ctrl Pts',(91.9978763183944,2.01412939086529,-0.906093372363755));
#16467=CARTESIAN_POINT('Ctrl Pts',(91.9892797493675,1.9516830603304,-1.03375560521944));
#16468=CARTESIAN_POINT('Ctrl Pts',(91.9719287786869,1.80015599103027,-1.28015889349355));
#16469=CARTESIAN_POINT('Ctrl Pts',(91.9632346386924,1.71047172036522,-1.39773653445652));
#16470=CARTESIAN_POINT('Ctrl Pts',(91.9535974999737,1.59240899594199,-1.52397187950321));
#16471=CARTESIAN_POINT('Ctrl Pts',(91.9521995715264,1.57480144341366,-1.54215991036318));
#16472=CARTESIAN_POINT('Ctrl Pts',(91.950025178691,1.54665866402641,-1.57024573459299));
#16473=CARTESIAN_POINT('Ctrl Pts',(91.9492396097857,1.53633313498483,-1.58034970887763));
#16474=CARTESIAN_POINT('Ctrl Pts',(91.9477772905553,1.5168183141829,-1.59907376797166));
#16475=CARTESIAN_POINT('Ctrl Pts',(91.9470995045348,1.50765305028828,-1.60771794876071));
#16476=CARTESIAN_POINT('Ctrl Pts',(91.9455869056911,1.48693203595516,-1.62692786125148));
#16477=CARTESIAN_POINT('Ctrl Pts',(91.9447539650389,1.47533673800317,-1.63745005173476));
#16478=CARTESIAN_POINT('Ctrl Pts',(91.9423267201468,1.44101343100652,-1.66793625292117));
#16479=CARTESIAN_POINT('Ctrl Pts',(91.9407466139509,1.41798494050082,-1.68755736994441));
#16480=CARTESIAN_POINT('Ctrl Pts',(91.9308945197218,1.2702782197703,-1.8082498664395));
#16481=CARTESIAN_POINT('Ctrl Pts',(91.9231771740635,1.13527811194518,-1.89592270148551));
#16482=CARTESIAN_POINT('Ctrl Pts',(91.9093122623397,0.879278297752528,-2.02494530864642));
#16483=CARTESIAN_POINT('Ctrl Pts',(91.903190707613,0.761957750317959,-2.07194273594277));
#16484=CARTESIAN_POINT('Ctrl Pts',(91.8957338898569,0.62634517940553,-2.11318512218995));
#16485=CARTESIAN_POINT('Ctrl Pts',(91.8949049601088,0.611363991790129,-2.11756787057247));
#16486=CARTESIAN_POINT('Ctrl Pts',(91.8936179581179,0.588279148973086,-2.12405595903169));
#16487=CARTESIAN_POINT('Ctrl Pts',(91.8931661562179,0.580207649863388,-2.12627494754705));
#16488=CARTESIAN_POINT('Ctrl Pts',(91.8923260822335,0.565265101118912,-2.13029148397796));
#16489=CARTESIAN_POINT('Ctrl Pts',(91.8919385459556,0.558397779714571,-2.13210186351864));
#16490=CARTESIAN_POINT('Ctrl Pts',(91.8910484528981,0.542682716396138,-2.13616357488154));
#16491=CARTESIAN_POINT('Ctrl Pts',(91.8905446920729,0.533829642173803,-2.13839314822935));
#16492=CARTESIAN_POINT('Ctrl Pts',(91.8889309677394,0.505590079216,-2.14531875496729));
#16493=CARTESIAN_POINT('Ctrl Pts',(91.8878101031735,0.486154098329247,-2.14980650858141));
#16494=CARTESIAN_POINT('Ctrl Pts',(91.8789429092045,0.333527782278194,-2.18287229632642));
#16495=CARTESIAN_POINT('Ctrl Pts',(91.8707011945206,0.198017004896817,-2.19930821391621));
#16496=CARTESIAN_POINT('Ctrl Pts',(91.8533571707245,-0.0908354350552137,
-2.2074196346521));
#16497=CARTESIAN_POINT('Ctrl Pts',(91.8443338211819,-0.243592257073614,
-2.19582084869509));
#16498=CARTESIAN_POINT('Ctrl Pts',(91.8344122704404,-0.418702875786694,
-2.16400955307388));
#16499=CARTESIAN_POINT('Ctrl Pts',(91.8330224797841,-0.44338770236666,-2.15908704399322));
#16500=CARTESIAN_POINT('Ctrl Pts',(91.8308578082635,-0.482070479621216,
-2.15068172066911));
#16501=CARTESIAN_POINT('Ctrl Pts',(91.8300739570427,-0.496127269191218,
-2.14748260938351));
#16502=CARTESIAN_POINT('Ctrl Pts',(91.8286132032865,-0.522411149182497,
-2.14122894343726));
#16503=CARTESIAN_POINT('Ctrl Pts',(91.8279352855326,-0.534645328525603,
-2.13820700093575));
#16504=CARTESIAN_POINT('Ctrl Pts',(91.8264203050548,-0.562062407453119,
-2.13118472882097));
#16505=CARTESIAN_POINT('Ctrl Pts',(91.8255851415365,-0.577229915056059,
-2.12712673357661));
#16506=CARTESIAN_POINT('Ctrl Pts',(91.8231448807168,-0.621690001683358,
-2.11472107088538));
#16507=CARTESIAN_POINT('Ctrl Pts',(91.8215542183305,-0.650854992629008,
-2.1059277202488));
#16508=CARTESIAN_POINT('Ctrl Pts',(91.8118917641264,-0.828852541915464,
-2.04820957818735));
#16509=CARTESIAN_POINT('Ctrl Pts',(91.8043442148215,-0.972299366408334,
-1.98413656711356));
#16510=CARTESIAN_POINT('Ctrl Pts',(91.7923917254874,-1.1860195688343,-1.859884515572));
#16511=CARTESIAN_POINT('Ctrl Pts',(91.7880061887851,-1.26140689016486,-1.80960315733449));
#16512=CARTESIAN_POINT('Ctrl Pts',(91.7811757802579,-1.36913612883749,-1.72774052240596));
#16513=CARTESIAN_POINT('Ctrl Pts',(91.7788712435987,-1.40395221871258,-1.6995701519728));
#16514=CARTESIAN_POINT('Ctrl Pts',(91.7758388653087,-1.44732806862101,-1.66223125549688));
#16515=CARTESIAN_POINT('Ctrl Pts',(91.7751734453719,-1.45670289370946,-1.65402175014187));
#16516=CARTESIAN_POINT('Ctrl Pts',(91.774088162018,-1.47174943637311,-1.64061839890208));
#16517=CARTESIAN_POINT('Ctrl Pts',(91.7736718343597,-1.47746459512303,-1.63547347906882));
#16518=CARTESIAN_POINT('Ctrl Pts',(91.7728592083842,-1.48850646148873,-1.62542822068468));
#16519=CARTESIAN_POINT('Ctrl Pts',(91.772463162685,-1.49383613424061,-1.62053138984471));
#16520=CARTESIAN_POINT('Ctrl Pts',(91.771572404995,-1.50571056742104,-1.60951296847784));
#16521=CARTESIAN_POINT('Ctrl Pts',(91.7710766691195,-1.51224230741066,-1.60337753088721));
#16522=CARTESIAN_POINT('Ctrl Pts',(91.7693205534058,-1.53511968954436,-1.5816240521812));
#16523=CARTESIAN_POINT('Ctrl Pts',(91.7680454757852,-1.55126174648873,-1.56579501107886));
#16524=CARTESIAN_POINT('Ctrl Pts',(91.7583708394835,-1.67052427240142,-1.44519068003146));
#16525=CARTESIAN_POINT('Ctrl Pts',(91.7494286567537,-1.76316839327559,-1.3305865807152));
#16526=CARTESIAN_POINT('Ctrl Pts',(91.7350743865384,-1.89452473885927,-1.13004107430255));
#16527=CARTESIAN_POINT('Ctrl Pts',(91.7295852564873,-1.94039567161276,-1.04932552983398));
#16528=CARTESIAN_POINT('Ctrl Pts',(91.7210390426506,-2.00553903071472,-0.915724834337237));
#16529=CARTESIAN_POINT('Ctrl Pts',(91.717884313861,-2.02811272669317,-0.864579857683288));
#16530=CARTESIAN_POINT('Ctrl Pts',(91.7137174048247,-2.05590711753306,-0.794507374510997));
#16531=CARTESIAN_POINT('Ctrl Pts',(91.7126478713954,-2.06285435441513,-0.776291176720659));
#16532=CARTESIAN_POINT('Ctrl Pts',(91.710867143915,-2.0741024470485,-0.745580015018834));
#16533=CARTESIAN_POINT('Ctrl Pts',(91.7101516181694,-2.07853418902356,-0.733134472906203));
#16534=CARTESIAN_POINT('Ctrl Pts',(91.7087450225014,-2.08707004861234,-0.708463749710086));
#16535=CARTESIAN_POINT('Ctrl Pts',(91.708053805019,-2.09117930068661,-0.696240917068855));
#16536=CARTESIAN_POINT('Ctrl Pts',(91.706376830118,-2.10093754151623,-0.666349391221354));
#16537=CARTESIAN_POINT('Ctrl Pts',(91.705394886591,-2.10647125442536,-0.64864392925449));
#16538=CARTESIAN_POINT('Ctrl Pts',(91.7020397650123,-2.12474419601195,-0.587476924950216));
#16539=CARTESIAN_POINT('Ctrl Pts',(91.6997025681194,-2.13636743309628,-0.543692553489345));
#16540=CARTESIAN_POINT('Ctrl Pts',(91.6890375462149,-2.18394678824568,-0.339249517722378));
#16541=CARTESIAN_POINT('Ctrl Pts',(91.681230242233,-2.20318018519569,-0.175249667298765));
#16542=CARTESIAN_POINT('Ctrl Pts',(91.6687584183441,-2.20441683530105,0.0810862893957523));
#16543=CARTESIAN_POINT('Ctrl Pts',(91.6642336862404,-2.1991334509297,0.172735538709611));
#16544=CARTESIAN_POINT('Ctrl Pts',(91.6583875930756,-2.18571214328869,0.284070644352944));
#16545=CARTESIAN_POINT('Ctrl Pts',(91.6573096193201,-2.182984064873,0.304325841682489));
#16546=CARTESIAN_POINT('Ctrl Pts',(91.6557186660863,-2.17860284762251,0.333755063207317));
#16547=CARTESIAN_POINT('Ctrl Pts',(91.6552174113932,-2.17717249237597,0.342961720874635));
#16548=CARTESIAN_POINT('Ctrl Pts',(91.6543281377425,-2.17454858312275,0.359172577760697));
#16549=CARTESIAN_POINT('Ctrl Pts',(91.6539414867107,-2.1733794756698,0.366180466757193));
#16550=CARTESIAN_POINT('Ctrl Pts',(91.6530962613843,-2.17076298476524,0.381410215844643));
#16551=CARTESIAN_POINT('Ctrl Pts',(91.6526370079661,-2.16930279018705,0.389629424653586));
#16552=CARTESIAN_POINT('Ctrl Pts',(91.6513417375729,-2.16507581827842,0.412661831270366));
#16553=CARTESIAN_POINT('Ctrl Pts',(91.6505001434403,-2.16220380953962,0.427454964131804));
#16554=CARTESIAN_POINT('Ctrl Pts',(91.6445678690501,-2.14107132115198,0.530636996928126));
#16555=CARTESIAN_POINT('Ctrl Pts',(91.6392369060706,-2.11754959161597,0.61785331576506));
#16556=CARTESIAN_POINT('Ctrl Pts',(91.6324450230468,-2.08130342556231,0.725490664067775));
#16557=CARTESIAN_POINT('Ctrl Pts',(91.6310452373882,-2.07350474498486,0.747488267342352));
#16558=CARTESIAN_POINT('Ctrl Pts',(91.62434902203,-2.03457634320534,0.851992448161574));
#16559=CARTESIAN_POINT('Ctrl Pts',(91.6190423037823,-1.99886162223261,0.932708625779653));
#16560=CARTESIAN_POINT('Ctrl Pts',(91.609975893247,-1.9284351121572,1.06912222443641));
#16561=CARTESIAN_POINT('Ctrl Pts',(91.6061750239318,-1.89589627490835,1.1258164640384));
#16562=CARTESIAN_POINT('Ctrl Pts',(91.5999399614086,-1.8372014427085,1.21830222802047));
#16563=CARTESIAN_POINT('Ctrl Pts',(91.5974625496646,-1.81240030819396,1.25490038556612));
#16564=CARTESIAN_POINT('Ctrl Pts',(91.594039917803,-1.77603503738983,1.30523397244636));
#16565=CARTESIAN_POINT('Ctrl Pts',(91.5930604675904,-1.76537961357666,1.31961017861556));
#16566=CARTESIAN_POINT('Ctrl Pts',(91.5913864298554,-1.74674069004093,1.34412777336433));
#16567=CARTESIAN_POINT('Ctrl Pts',(91.5906886072256,-1.73884113575029,1.35433157827334));
#16568=CARTESIAN_POINT('Ctrl Pts',(91.5893581876538,-1.72353268344536,1.3737506610727));
#16569=CARTESIAN_POINT('Ctrl Pts',(91.5887250454644,-1.71613837163128,1.38297682070981));
#16570=CARTESIAN_POINT('Ctrl Pts',(91.5870756340192,-1.69659182655424,1.40696759812028));
#16571=CARTESIAN_POINT('Ctrl Pts',(91.5860641919308,-1.68432092249591,1.42163452015283));
#16572=CARTESIAN_POINT('Ctrl Pts',(91.5824965827552,-1.64004350379028,1.47317939291205));
#16573=CARTESIAN_POINT('Ctrl Pts',(91.579982947469,-1.607003189443,1.50915254989417));
#16574=CARTESIAN_POINT('Ctrl Pts',(91.5693511268562,-1.45992062750809,1.65897797078968));
#16575=CARTESIAN_POINT('Ctrl Pts',(91.5617111185671,-1.3347844079203,1.76122910246705));
#16576=CARTESIAN_POINT('Ctrl Pts',(91.5494617479465,-1.12367950143193,1.8981976602712));
#16577=CARTESIAN_POINT('Ctrl Pts',(91.5449922625519,-1.04478538648991,1.94273788818145));
#16578=CARTESIAN_POINT('Ctrl Pts',(91.5392138171219,-0.94511276301666,1.99117819444384));
#16579=CARTESIAN_POINT('Ctrl Pts',(91.5381421039575,-0.926719158480925,
1.99980506055949));
#16580=CARTESIAN_POINT('Ctrl Pts',(91.5365587222451,-0.899740337264539,
2.01200639279583));
#16581=CARTESIAN_POINT('Ctrl Pts',(91.5360586214673,-0.891247095780816,
2.01578297619448));
#16582=CARTESIAN_POINT('Ctrl Pts',(91.5351705895025,-0.876221705145017,
2.02235060758127));
#16583=CARTESIAN_POINT('Ctrl Pts',(91.5347840116903,-0.869699594866195,
2.02516396119144));
#16584=CARTESIAN_POINT('Ctrl Pts',(91.5339379629519,-0.855467938706829,
2.03122144589011));
#16585=CARTESIAN_POINT('Ctrl Pts',(91.5334778018349,-0.847753600945764,
2.03445319035581));
#16586=CARTESIAN_POINT('Ctrl Pts',(91.5321776610022,-0.826024083013494,
2.04341122389381));
#16587=CARTESIAN_POINT('Ctrl Pts',(91.5313320410067,-0.811968283577297,
2.04903701680671));
#16588=CARTESIAN_POINT('Ctrl Pts',(91.525135540866,-0.70942853099964,2.0888575419592));
#16589=CARTESIAN_POINT('Ctrl Pts',(91.5195195484463,-0.618884030880044,
2.11744984807348));
#16590=CARTESIAN_POINT('Ctrl Pts',(91.5124900591962,-0.504872575052794,
2.14551372293018));
#16591=CARTESIAN_POINT('Ctrl Pts',(91.5111353931813,-0.482874269982661,
2.15057152408412));
#16592=CARTESIAN_POINT('Ctrl Pts',(91.5040061829274,-0.366801161465693,
2.17538801856326));
#16593=CARTESIAN_POINT('Ctrl Pts',(91.498227930365,-0.271581082322755,2.18931533262676));
#16594=CARTESIAN_POINT('Ctrl Pts',(91.4891595822157,-0.117678594080809,
2.2016271017));
#16595=CARTESIAN_POINT('Ctrl Pts',(91.4857881136124,-0.059440386435164,
2.20396864495139));
#16596=CARTESIAN_POINT('Ctrl Pts',(91.4824602988302,-0.000782819936893213,
2.20399989587492));
#16597=CARTESIAN_POINT('Ctrl Pts',(91.4824380960676,-0.000391409701139083,
2.204));
#16598=CARTESIAN_POINT('Ctrl Pts',(91.4824158962551,-3.3646198792706E-12,
2.204));
#16599=CARTESIAN_POINT('Ctrl Pts',(91.3776298668357,4.55134372080087E-12,
2.204));
#16600=CARTESIAN_POINT('Ctrl Pts',(91.3776497873187,-0.000393697700173932,
2.204));
#16601=CARTESIAN_POINT('Ctrl Pts',(91.3776697052255,-0.0007873964541778,
2.20399989455858));
#16602=CARTESIAN_POINT('Ctrl Pts',(91.3817409009304,-0.0812697516293409,
2.20395676479764));
#16603=CARTESIAN_POINT('Ctrl Pts',(91.3856766082689,-0.161299799345881,
2.19954852774969));
#16604=CARTESIAN_POINT('Ctrl Pts',(91.3950873875084,-0.353788069461133,
2.17838110266901));
#16605=CARTESIAN_POINT('Ctrl Pts',(91.4005006362243,-0.465527647417681,
2.15726502739082));
#16606=CARTESIAN_POINT('Ctrl Pts',(91.4063620569227,-0.579759015343803,
2.12638622936986));
#16607=CARTESIAN_POINT('Ctrl Pts',(91.4065995345294,-0.584375747435629,
2.12512209008459));
#16608=CARTESIAN_POINT('Ctrl Pts',(91.4098781767823,-0.647949740735055,
2.10749162497104));
#16609=CARTESIAN_POINT('Ctrl Pts',(91.412982708196,-0.706200208886684,2.08869334756884));
#16610=CARTESIAN_POINT('Ctrl Pts',(91.4169634216333,-0.77697600000046,2.06255375000772));
#16611=CARTESIAN_POINT('Ctrl Pts',(91.417723017175,-0.790314941408937,2.05747951346729));
#16612=CARTESIAN_POINT('Ctrl Pts',(91.4189273759722,-0.811180928265386,
2.04930908499334));
#16613=CARTESIAN_POINT('Ctrl Pts',(91.419367140723,-0.818741929583332,2.04630004462266));
#16614=CARTESIAN_POINT('Ctrl Pts',(91.4202030750725,-0.832999891793393,
2.04053415280962));
#16615=CARTESIAN_POINT('Ctrl Pts',(91.4205987319439,-0.839700135165113,
2.03778608444771));
#16616=CARTESIAN_POINT('Ctrl Pts',(91.4215420333139,-0.855562941688378,
2.03118852495752));
#16617=CARTESIAN_POINT('Ctrl Pts',(91.4220913818566,-0.864713170045411,
2.02731001499579));
#16618=CARTESIAN_POINT('Ctrl Pts',(91.4239617528901,-0.895585130120537,
2.0139772814237));
#16619=CARTESIAN_POINT('Ctrl Pts',(91.4252985594738,-0.917179859359909,
2.00423507311758));
#16620=CARTESIAN_POINT('Ctrl Pts',(91.4286290665147,-0.969961077375128,
1.97939181664637));
#16621=CARTESIAN_POINT('Ctrl Pts',(91.4306400661709,-1.00095603528033,1.96390001061502));
#16622=CARTESIAN_POINT('Ctrl Pts',(91.4395640170308,-1.13532990018562,1.89273025986807));
#16623=CARTESIAN_POINT('Ctrl Pts',(91.4466850750587,-1.23452874148243,1.8295736791617));
#16624=CARTESIAN_POINT('Ctrl Pts',(91.4615790492524,-1.43330479531993,1.67946206313205));
#16625=CARTESIAN_POINT('Ctrl Pts',(91.4692890590268,-1.53107594060421,1.59083972993484));
#16626=CARTESIAN_POINT('Ctrl Pts',(91.4780066811962,-1.63710596780252,1.47584225705893));
#16627=CARTESIAN_POINT('Ctrl Pts',(91.4793707631218,-1.65354614096831,1.45739889781873));
#16628=CARTESIAN_POINT('Ctrl Pts',(91.4815174627805,-1.6791686944301,1.42766246014448));
#16629=CARTESIAN_POINT('Ctrl Pts',(91.4823084792419,-1.688554971239,1.4165485264697));
#16630=CARTESIAN_POINT('Ctrl Pts',(91.483776805428,-1.70587152075336,1.39562795113253));
#16631=CARTESIAN_POINT('Ctrl Pts',(91.4844552060113,-1.71382894303037,1.38584464732226));
#16632=CARTESIAN_POINT('Ctrl Pts',(91.4859774240675,-1.73158288037588,1.36363015860112));
#16633=CARTESIAN_POINT('Ctrl Pts',(91.486819261979,-1.74133039584258,1.35116059418951));
#16634=CARTESIAN_POINT('Ctrl Pts',(91.489328478301,-1.77015958708026,1.31345047701963));
#16635=CARTESIAN_POINT('Ctrl Pts',(91.4909799468487,-1.78883331948359,1.28790240581569));
#16636=CARTESIAN_POINT('Ctrl Pts',(91.4947491260432,-1.83066877875324,1.22799985983965));
#16637=CARTESIAN_POINT('Ctrl Pts',(91.4968523060118,-1.85342509817297,1.19337650818241));
#16638=CARTESIAN_POINT('Ctrl Pts',(91.5044172079401,-1.93272958052811,1.0649703041475));
#16639=CARTESIAN_POINT('Ctrl Pts',(91.5096995520165,-1.98324583884367,0.96764811528813));
#16640=CARTESIAN_POINT('Ctrl Pts',(91.5210940804545,-2.0759772333159,0.750912928935033));
#16641=CARTESIAN_POINT('Ctrl Pts',(91.527189841773,-2.11556595370753,0.63081340941809));
#16642=CARTESIAN_POINT('Ctrl Pts',(91.5348377651341,-2.14938557500779,0.488035531981092));
#16643=CARTESIAN_POINT('Ctrl Pts',(91.5359198798327,-2.15383579872805,0.468004618669745));
#16644=CARTESIAN_POINT('Ctrl Pts',(91.5375134493021,-2.15989300235521,0.438821687131036));
#16645=CARTESIAN_POINT('Ctrl Pts',(91.5380130469979,-2.16172292181633,0.429716485297551));
#16646=CARTESIAN_POINT('Ctrl Pts',(91.5389046743222,-2.16486547723034,0.413551718194397));
#16647=CARTESIAN_POINT('Ctrl Pts',(91.5392953981207,-2.16620123892506,0.406496923906515));
#16648=CARTESIAN_POINT('Ctrl Pts',(91.5401485414847,-2.16902809379142,0.391157239176011));
#16649=CARTESIAN_POINT('Ctrl Pts',(91.5406116421218,-2.17050618442878,0.382870416649713));
#16650=CARTESIAN_POINT('Ctrl Pts',(91.5419397911224,-2.17458671010755,0.359209914847188));
#16651=CARTESIAN_POINT('Ctrl Pts',(91.5428109411612,-2.17707346922702,0.343817108458859));
#16652=CARTESIAN_POINT('Ctrl Pts',(91.5448145660014,-2.18237051306425,0.308663725131759));
#16653=CARTESIAN_POINT('Ctrl Pts',(91.5459518012419,-2.18507608418323,0.288888917409796));
#16654=CARTESIAN_POINT('Ctrl Pts',(91.5557129420421,-2.20580301674085,0.120387726461102));
#16655=CARTESIAN_POINT('Ctrl Pts',(91.564849446274,-2.20888459567789,-0.0297765807555846));
#16656=CARTESIAN_POINT('Ctrl Pts',(91.5813600640831,-2.18641846177745,-0.305349903894416));
#16657=CARTESIAN_POINT('Ctrl Pts',(91.5887617838061,-2.16525710446567,-0.430504484890412));
#16658=CARTESIAN_POINT('Ctrl Pts',(91.5971927709482,-2.12728360785889,-0.576961809773478));
#16659=CARTESIAN_POINT('Ctrl Pts',(91.5985501440626,-2.1207149871722,-0.600656716048967));
#16660=CARTESIAN_POINT('Ctrl Pts',(91.6006886795398,-2.10963887385296,-0.63816190934446));
#16661=CARTESIAN_POINT('Ctrl Pts',(91.6014781359966,-2.1053891159868,-0.652045615807265));
#16662=CARTESIAN_POINT('Ctrl Pts',(91.602944953952,-2.09719202497965,-0.677909042259047));
#16663=CARTESIAN_POINT('Ctrl Pts',(91.6036233886024,-2.09327847008446,-0.689898771617686));
#16664=CARTESIAN_POINT('Ctrl Pts',(91.6051474582162,-2.08421110636715,-0.716890266186869));
#16665=CARTESIAN_POINT('Ctrl Pts',(91.6059910905471,-2.07899780249331,-0.731871399031573));
#16666=CARTESIAN_POINT('Ctrl Pts',(91.6085118097496,-2.06283882042617,-0.776739976308074));
#16667=CARTESIAN_POINT('Ctrl Pts',(91.610172758436,-2.05140680688962,-0.806448533546961));
#16668=CARTESIAN_POINT('Ctrl Pts',(91.613967368431,-2.02350234654679,-0.874526693965781));
#16669=CARTESIAN_POINT('Ctrl Pts',(91.61608620494,-2.00657500557723,-0.912696931455176));
#16670=CARTESIAN_POINT('Ctrl Pts',(91.623742500892,-1.94068508660386,-1.050567054278));
#16671=CARTESIAN_POINT('Ctrl Pts',(91.6290953902265,-1.88529029342755,-1.14700993441016));
#16672=CARTESIAN_POINT('Ctrl Pts',(91.6404537402205,-1.75321620865761,-1.34134277806872));
#16673=CARTESIAN_POINT('Ctrl Pts',(91.6464448151753,-1.67506129404871,-1.43775194858175));
#16674=CARTESIAN_POINT('Ctrl Pts',(91.653974394663,-1.57495580647477,-1.5419321637822));
#16675=CARTESIAN_POINT('Ctrl Pts',(91.6550609477213,-1.56047176233966,-1.55658870891824));
#16676=CARTESIAN_POINT('Ctrl Pts',(91.6566598595932,-1.53915392840911,-1.57756385653583));
#16677=CARTESIAN_POINT('Ctrl Pts',(91.657160247883,-1.53248185702167,-1.58404604995512));
#16678=CARTESIAN_POINT('Ctrl Pts',(91.6580527425156,-1.52058634066934,-1.59545753955939));
#16679=CARTESIAN_POINT('Ctrl Pts',(91.6584435332603,-1.5153795583386,-1.6004038155088));
#16680=CARTESIAN_POINT('Ctrl Pts',(91.6592961754356,-1.50402471161696,-1.61108545850678));
#16681=CARTESIAN_POINT('Ctrl Pts',(91.6597587006576,-1.49786806769339,-1.61681103866241));
#16682=CARTESIAN_POINT('Ctrl Pts',(91.6610834479012,-1.48023736115415,-1.63302018170824));
#16683=CARTESIAN_POINT('Ctrl Pts',(91.66195172347,-1.4686851810235,-1.64341758853522));
#16684=CARTESIAN_POINT('Ctrl Pts',(91.6697166066552,-1.36530253341888,-1.73450532860287));
#16685=CARTESIAN_POINT('Ctrl Pts',(91.6770487328687,-1.26702414325333,-1.80754095284121));
#16686=CARTESIAN_POINT('Ctrl Pts',(91.6942956777497,-1.02318000030342,-1.95905523859537));
#16687=CARTESIAN_POINT('Ctrl Pts',(91.7041330887592,-0.873807593510924,
-2.03009147201441));
#16688=CARTESIAN_POINT('Ctrl Pts',(91.71492361511,-0.691996546468892,-2.09272714715062));
#16689=CARTESIAN_POINT('Ctrl Pts',(91.7164450489779,-0.665936806524459,
-2.10116500961688));
#16690=CARTESIAN_POINT('Ctrl Pts',(91.7188538399707,-0.624002490387734,
-2.113884305136));
#16691=CARTESIAN_POINT('Ctrl Pts',(91.7197512553216,-0.608226152910891,
-2.11847750308101));
#16692=CARTESIAN_POINT('Ctrl Pts',(91.721338645453,-0.58005124675161,-2.12633979111678));
#16693=CARTESIAN_POINT('Ctrl Pts',(91.7220308361001,-0.567672868549915,
-2.12967788178312));
#16694=CARTESIAN_POINT('Ctrl Pts',(91.7234752066212,-0.541652686219961,
-2.13645178890026));
#16695=CARTESIAN_POINT('Ctrl Pts',(91.7242266415553,-0.528005664285126,
-2.13986539526126));
#16696=CARTESIAN_POINT('Ctrl Pts',(91.7262019539813,-0.49184833557254,-2.14854266681873));
#16697=CARTESIAN_POINT('Ctrl Pts',(91.7274186551605,-0.46928598861023,-2.15358331408037));
#16698=CARTESIAN_POINT('Ctrl Pts',(91.7336079355327,-0.353107999423411,
-2.17762604359026));
#16699=CARTESIAN_POINT('Ctrl Pts',(91.7383959974413,-0.258403858195734,
-2.19088350613045));
#16700=CARTESIAN_POINT('Ctrl Pts',(91.749536065119,-0.0320016969515925,
-2.20768685813454));
#16701=CARTESIAN_POINT('Ctrl Pts',(91.7557689060371,0.0997292633399901,
-2.20566491624735));
#16702=CARTESIAN_POINT('Ctrl Pts',(91.7636759866867,0.259382152033342,-2.18887661580208));
#16703=CARTESIAN_POINT('Ctrl Pts',(91.7651187476883,0.288209889429562,-2.18526769820067));
#16704=CARTESIAN_POINT('Ctrl Pts',(91.7689830054256,0.364256708917513,-2.17421653728006));
#16705=CARTESIAN_POINT('Ctrl Pts',(91.7714341207368,0.411317136494377,-2.16580657081204));
#16706=CARTESIAN_POINT('Ctrl Pts',(91.7746624002179,0.471029246601015,-2.15311939853649));
#16707=CARTESIAN_POINT('Ctrl Pts',(91.7753691712496,0.483969399437671,-2.15024772959854));
#16708=CARTESIAN_POINT('Ctrl Pts',(91.7765081951137,0.504592834162175,-2.14547540271095));
#16709=CARTESIAN_POINT('Ctrl Pts',(91.7769363102217,0.512293337088345,-2.14364972994317));
#16710=CARTESIAN_POINT('Ctrl Pts',(91.7777651821034,0.527099293794177,-2.1400551278568));
#16711=CARTESIAN_POINT('Ctrl Pts',(91.778165604664,0.534205988368107,-2.1382922092265));
#16712=CARTESIAN_POINT('Ctrl Pts',(91.7791419003741,0.551425687302881,-2.13392941414762));
#16713=CARTESIAN_POINT('Ctrl Pts',(91.7797198114331,0.561529200579008,-2.13129303033152));
#16714=CARTESIAN_POINT('Ctrl Pts',(91.7817996136798,0.597588802205233,-2.12160953119154));
#16715=CARTESIAN_POINT('Ctrl Pts',(91.783322248456,0.623433194688759,-2.11415947806979));
#16716=CARTESIAN_POINT('Ctrl Pts',(91.7872305614863,0.688578467176918,-2.09408199020002));
#16717=CARTESIAN_POINT('Ctrl Pts',(91.7896415002397,0.727672216614691,-2.08082014959478));
#16718=CARTESIAN_POINT('Ctrl Pts',(91.802606518549,0.933483177393505,-2.00449332548636));
#16719=CARTESIAN_POINT('Ctrl Pts',(91.8135193958348,1.09248855624563,-1.92246315836466));
#16720=CARTESIAN_POINT('Ctrl Pts',(91.8277320271604,1.2950213652082,-1.78465261417891));
#16721=CARTESIAN_POINT('Ctrl Pts',(91.8315240056046,1.34844031435482,-1.74464188907611));
#16722=CARTESIAN_POINT('Ctrl Pts',(91.8364127922964,1.41653783805181,-1.68863759162108));
#16723=CARTESIAN_POINT('Ctrl Pts',(91.8375927672744,1.43290998738678,-1.67476726040434));
#16724=CARTESIAN_POINT('Ctrl Pts',(91.8395107369848,1.45940843057469,-1.65164494633508));
#16725=CARTESIAN_POINT('Ctrl Pts',(91.8402544735503,1.46965526582547,-1.64253383756608));
#16726=CARTESIAN_POINT('Ctrl Pts',(91.8416927119705,1.48941131819245,-1.62463459027004));
#16727=CARTESIAN_POINT('Ctrl Pts',(91.8423876183539,1.49892941153607,-1.61585712728249));
#16728=CARTESIAN_POINT('Ctrl Pts',(91.8440169256429,1.52117671096957,-1.59497521473353));
#16729=CARTESIAN_POINT('Ctrl Pts',(91.8449482945539,1.53383975000811,-1.58280136685571));
#16730=CARTESIAN_POINT('Ctrl Pts',(91.8480555567873,1.5758834056257,-1.54140346188619));
#16731=CARTESIAN_POINT('Ctrl Pts',(91.8502016896559,1.60458593802326,-1.51150170165982));
#16732=CARTESIAN_POINT('Ctrl Pts',(91.8553554381694,1.67243024209419,-1.43671069857977));
#16733=CARTESIAN_POINT('Ctrl Pts',(91.8583273949453,1.71062931436566,-1.39100989155555));
#16734=CARTESIAN_POINT('Ctrl Pts',(91.8659189541454,1.80467201948883,-1.26875636994954));
#16735=CARTESIAN_POINT('Ctrl Pts',(91.8704642064856,1.857514646127,-1.19005191723368));
#16736=CARTESIAN_POINT('Ctrl Pts',(91.8765366517972,1.92054919879009,-1.08168713051415));
#16737=CARTESIAN_POINT('Ctrl Pts',(91.8780261522123,1.93541228142226,-1.05486280081008));
#16738=CARTESIAN_POINT('Ctrl Pts',(91.883733348176,1.98980363117531,-0.951677504658571));
#16739=CARTESIAN_POINT('Ctrl Pts',(91.8880186790286,2.02540778144843,-0.873343588386556));
#16740=CARTESIAN_POINT('Ctrl Pts',(91.8933376123173,2.06176373595543,-0.779084854719754));
#16741=CARTESIAN_POINT('Ctrl Pts',(91.894137974545,2.06704022049623,-0.764975565514932));
#16742=CARTESIAN_POINT('Ctrl Pts',(91.8953972268463,2.07503180512173,-0.742919582378854));
#16743=CARTESIAN_POINT('Ctrl Pts',(91.8958504619992,2.07784690980209,-0.735009328402896));
#16744=CARTESIAN_POINT('Ctrl Pts',(91.8966927851086,2.08296410203773,-0.720366005703706));
#16745=CARTESIAN_POINT('Ctrl Pts',(91.8970811282799,2.08527886270637,-0.713637648015302));
#16746=CARTESIAN_POINT('Ctrl Pts',(91.8979890650241,2.09058822154249,-0.697958431430296));
#16747=CARTESIAN_POINT('Ctrl Pts',(91.8985100702102,2.09355793715396,-0.688999449306322));
#16748=CARTESIAN_POINT('Ctrl Pts',(91.9001893186055,2.10288820661926,-0.660234741274431));
#16749=CARTESIAN_POINT('Ctrl Pts',(91.9013594253114,2.10902576190551,-0.640358489123532));
#16750=CARTESIAN_POINT('Ctrl Pts',(91.9079172659481,2.14149294730569,-0.529680978739443));
#16751=CARTESIAN_POINT('Ctrl Pts',(91.9135409171221,2.16223834853384,-0.437351568571615));
#16752=CARTESIAN_POINT('Ctrl Pts',(91.9296044761519,2.20404566552599,-0.17276353793493));
#16753=CARTESIAN_POINT('Ctrl Pts',(91.9400431913294,2.21080998527135,0.00108088287678498));
#16754=CARTESIAN_POINT('Ctrl Pts',(91.9519407566671,2.19420681588039,0.210809556561447));
#16755=CARTESIAN_POINT('Ctrl Pts',(91.9540050115326,2.19035975198268,0.247605755228386));
#16756=CARTESIAN_POINT('Ctrl Pts',(91.956970004875,2.18340907772031,0.301041848292649));
#16757=CARTESIAN_POINT('Ctrl Pts',(91.9578934654244,2.1810374218173,0.317769070498981));
#16758=CARTESIAN_POINT('Ctrl Pts',(91.9595106911321,2.17651784310179,0.34720624128054));
#16759=CARTESIAN_POINT('Ctrl Pts',(91.9602069624109,2.17445033473915,0.359927557905491));
#16760=CARTESIAN_POINT('Ctrl Pts',(91.961644278822,2.16992933580395,0.386283007250181));
#16761=CARTESIAN_POINT('Ctrl Pts',(91.9623847440086,2.1674586451363,0.399913637824268));
#16762=CARTESIAN_POINT('Ctrl Pts',(91.9642970407964,2.16070976558687,0.435245342066936));
#16763=CARTESIAN_POINT('Ctrl Pts',(91.9654625242916,2.15623307281403,0.456907191456433));
#16764=CARTESIAN_POINT('Ctrl Pts',(91.970854196108,2.13382902221312,0.557640559977619));
#16765=CARTESIAN_POINT('Ctrl Pts',(91.974950808638,2.11187274300309,0.635755125075461));
#16766=CARTESIAN_POINT('Ctrl Pts',(91.9891047253716,2.01936727305806,0.906545543536755));
#16767=CARTESIAN_POINT('Ctrl Pts',(91.99854707361,1.92632764621014,1.09037139324226));
#16768=CARTESIAN_POINT('Ctrl Pts',(92.0104608247405,1.79462730077302,1.27968124931439));
#16769=CARTESIAN_POINT('Ctrl Pts',(92.0118015169946,1.77964444597949,1.30043715122988));
#16770=CARTESIAN_POINT('Ctrl Pts',(92.0137257325496,1.75799438274974,1.32935420012301));
#16771=CARTESIAN_POINT('Ctrl Pts',(92.0142903517085,1.75162443324855,1.33773639968258));
#16772=CARTESIAN_POINT('Ctrl Pts',(92.0152515795808,1.74075785871653,1.35182500920623));
#16773=CARTESIAN_POINT('Ctrl Pts',(92.015646025913,1.73629253518679,1.35755552725237));
#16774=CARTESIAN_POINT('Ctrl Pts',(92.0164714375588,1.72693819155161,1.36943865788802));
#16775=CARTESIAN_POINT('Ctrl Pts',(92.0169027144122,1.72204451074607,1.37558731245748));
#16776=CARTESIAN_POINT('Ctrl Pts',(92.0180535727462,1.70896633641264,1.39184020007513));
#16777=CARTESIAN_POINT('Ctrl Pts',(92.0187770201623,1.70072524786362,1.40189824739245));
#16778=CARTESIAN_POINT('Ctrl Pts',(92.0223214531359,1.66022444146323,1.45044576832971));
#16779=CARTESIAN_POINT('Ctrl Pts',(92.0252177974617,1.62674658586073,1.4878954729299));
#16780=CARTESIAN_POINT('Ctrl Pts',(92.0346999724233,1.51490764521916,1.60471344520302));
#16781=CARTESIAN_POINT('Ctrl Pts',(92.0414524162853,1.43179417154656,1.67928997591744));
#16782=CARTESIAN_POINT('Ctrl Pts',(92.0557939701127,1.24195948820453,1.82524650235054));
#16783=CARTESIAN_POINT('Ctrl Pts',(92.063325517908,1.13391187701719,1.89426502704868));
#16784=CARTESIAN_POINT('Ctrl Pts',(92.072270166758,0.992819653283209,1.96796810016855));
#16785=CARTESIAN_POINT('Ctrl Pts',(92.0740032226068,0.964862797213367,1.98182472242866));
#16786=CARTESIAN_POINT('Ctrl Pts',(92.0765909358015,0.922186271688614,2.00185981846796));
#16787=CARTESIAN_POINT('Ctrl Pts',(92.0774607104127,0.90767905635058,2.00847927596927));
#16788=CARTESIAN_POINT('Ctrl Pts',(92.0790154608451,0.881457341838468,2.02010177086763));
#16789=CARTESIAN_POINT('Ctrl Pts',(92.0797023651437,0.869768995323809,2.02516175018502));
#16790=CARTESIAN_POINT('Ctrl Pts',(92.081164233774,0.844676062666869,2.03576736427398));
#16791=CARTESIAN_POINT('Ctrl Pts',(92.0819381399571,0.831259220410901,2.04128257096149));
#16792=CARTESIAN_POINT('Ctrl Pts',(92.0840427234432,0.794418110215777,2.05600322277211));
#16793=CARTESIAN_POINT('Ctrl Pts',(92.0853643974157,0.770888713594534,2.06494068814135));
#16794=CARTESIAN_POINT('Ctrl Pts',(92.0945362357198,0.605001546982336,2.12472089565496));
#16795=CARTESIAN_POINT('Ctrl Pts',(92.1018839744866,0.457895477860774,2.16120416521849));
#16796=CARTESIAN_POINT('Ctrl Pts',(92.1141757669867,0.206092714154166,2.19676480157138));
#16797=CARTESIAN_POINT('Ctrl Pts',(92.1191372854593,0.103106355978515,2.20399999999999));
#16798=CARTESIAN_POINT('Ctrl Pts',(92.1243308360554,1.24855421140824E-11,
2.20399999999999));
#16799=CARTESIAN_POINT('Origin',(66.9212607628943,0.,0.));
#16800=CARTESIAN_POINT('',(92.9850149380438,-5.17304578464428E-12,2.204));
#16801=CARTESIAN_POINT('',(92.8757411398941,1.22339489286472E-10,2.204));
#16802=CARTESIAN_POINT('',(66.9212607628943,-2.69912154532077E-16,2.204));
#16803=CARTESIAN_POINT('',(92.2357264933075,-0.00128844900583903,2.20399983654467));
#16804=CARTESIAN_POINT('Ctrl Pts',(92.9850149380438,-5.17304578464428E-12,
2.204));
#16805=CARTESIAN_POINT('Ctrl Pts',(92.9849839122787,0.000639203858989945,
2.204));
#16806=CARTESIAN_POINT('Ctrl Pts',(92.9849528833965,0.00127841658233731,
2.20399972192954));
#16807=CARTESIAN_POINT('Ctrl Pts',(92.9797323214733,0.108815440439529,2.20390615691735));
#16808=CARTESIAN_POINT('Ctrl Pts',(92.974478251419,0.215553806951163,2.19603613966628));
#16809=CARTESIAN_POINT('Ctrl Pts',(92.9680527442138,0.336335811111836,2.17823910869595));
#16810=CARTESIAN_POINT('Ctrl Pts',(92.9672447349579,0.351361136673496,2.17586596982931));
#16811=CARTESIAN_POINT('Ctrl Pts',(92.9659786535206,0.374623324503134,2.17194465465864));
#16812=CARTESIAN_POINT('Ctrl Pts',(92.9655264029516,0.382878224169359,2.17050465996205));
#16813=CARTESIAN_POINT('Ctrl Pts',(92.9646859458543,0.398112959507861,2.16775748114263));
#16814=CARTESIAN_POINT('Ctrl Pts',(92.9642984812101,0.405094919564516,2.16646359935022));
#16815=CARTESIAN_POINT('Ctrl Pts',(92.9634006733272,0.421178842820127,2.16340249362275));
#16816=CARTESIAN_POINT('Ctrl Pts',(92.9628890277217,0.430275993989048,2.16161155846629));
#16817=CARTESIAN_POINT('Ctrl Pts',(92.9612537321165,0.4591452608254,2.15573867343655));
#16818=CARTESIAN_POINT('Ctrl Pts',(92.960118947242,0.478872181017981,2.15144253327758));
#16819=CARTESIAN_POINT('Ctrl Pts',(92.9539006013826,0.585509899658901,2.12667966949229));
#16820=CARTESIAN_POINT('Ctrl Pts',(92.9486045419589,0.671168781968484,2.10121824082946));
#16821=CARTESIAN_POINT('Ctrl Pts',(92.933819310583,0.903071985138849,2.01665670528945));
#16822=CARTESIAN_POINT('Ctrl Pts',(92.9242974386048,1.04490898995667,1.94695132625936));
#16823=CARTESIAN_POINT('Ctrl Pts',(92.9122357445336,1.22253376590112,1.8346091148031));
#16824=CARTESIAN_POINT('Ctrl Pts',(92.9092709747304,1.26594452711196,1.80492784435747));
#16825=CARTESIAN_POINT('Ctrl Pts',(92.9052768022982,1.32407975285801,1.76204865563998));
#16826=CARTESIAN_POINT('Ctrl Pts',(92.904197761914,1.33974792228667,1.75016519132171));
#16827=CARTESIAN_POINT('Ctrl Pts',(92.9024777542054,1.36465654354071,1.73074279950544));
#16828=CARTESIAN_POINT('Ctrl Pts',(92.90183161925,1.37399825171393,1.72333598929291));
#16829=CARTESIAN_POINT('Ctrl Pts',(92.9004964246188,1.393267479012,1.70780160623859));
#16830=CARTESIAN_POINT('Ctrl Pts',(92.8998078689158,1.40318506811633,1.69966239841522));
#16831=CARTESIAN_POINT('Ctrl Pts',(92.8981903778024,1.4264317070319,1.68024209092026));
#16832=CARTESIAN_POINT('Ctrl Pts',(92.8972644608044,1.43969897980819,1.66888818381006));
#16833=CARTESIAN_POINT('Ctrl Pts',(92.8941624146894,1.48399128840569,1.63006226772277));
#16834=CARTESIAN_POINT('Ctrl Pts',(92.8920161254101,1.51437700350201,1.60187256617595));
#16835=CARTESIAN_POINT('Ctrl Pts',(92.8868545313899,1.58654273916021,1.53103239358963));
#16836=CARTESIAN_POINT('Ctrl Pts',(92.8838752364433,1.62742016329827,1.48750875411669));
#16837=CARTESIAN_POINT('Ctrl Pts',(92.8762792536898,1.72842160532998,1.37081453465306));
#16838=CARTESIAN_POINT('Ctrl Pts',(92.8717365304916,1.785687956913,1.29533495886259));
#16839=CARTESIAN_POINT('Ctrl Pts',(92.8656308010742,1.85525689813687,1.19022016947047));
#16840=CARTESIAN_POINT('Ctrl Pts',(92.86410524841,1.87202714204781,1.16366513212299));
#16841=CARTESIAN_POINT('Ctrl Pts',(92.8583877438188,1.93227596821877,1.06358845770907));
#16842=CARTESIAN_POINT('Ctrl Pts',(92.8541286082913,1.97203320318755,0.98792360780754));
#16843=CARTESIAN_POINT('Ctrl Pts',(92.8488443193015,2.01347217265633,0.896531896249151));
#16844=CARTESIAN_POINT('Ctrl Pts',(92.8480496416932,2.01950867408486,0.882850113037087));
#16845=CARTESIAN_POINT('Ctrl Pts',(92.8468001193165,2.02868709726872,0.861460343411248));
#16846=CARTESIAN_POINT('Ctrl Pts',(92.8463508577373,2.0319254780675,0.853793949886412));
#16847=CARTESIAN_POINT('Ctrl Pts',(92.845516610347,2.0378233577995,0.839607967547692));
#16848=CARTESIAN_POINT('Ctrl Pts',(92.8451323630115,2.04049512523086,0.833093761964362));
#16849=CARTESIAN_POINT('Ctrl Pts',(92.8442353798318,2.04662909675851,0.817931606398258));
#16850=CARTESIAN_POINT('Ctrl Pts',(92.8437212781954,2.0500677244246,0.80927442272493));
#16851=CARTESIAN_POINT('Ctrl Pts',(92.8420701584996,2.06087114413694,0.781564691370285));
#16852=CARTESIAN_POINT('Ctrl Pts',(92.840921711227,2.06802578976791,0.762431971692556));
#16853=CARTESIAN_POINT('Ctrl Pts',(92.8345558829956,2.10580332263445,0.656962710964858));
#16854=CARTESIAN_POINT('Ctrl Pts',(92.8291155984555,2.13128426196491,0.568886872142082));
#16855=CARTESIAN_POINT('Ctrl Pts',(92.8137824224623,2.18694565302358,0.319164456967255));
#16856=CARTESIAN_POINT('Ctrl Pts',(92.8038694073796,2.20465093358873,0.155322261893016));
#16857=CARTESIAN_POINT('Ctrl Pts',(92.7918959682104,2.20379594361052,-0.0545865236937455));
#16858=CARTESIAN_POINT('Ctrl Pts',(92.789334834381,2.20219444976358,-0.100181273902928));
#16859=CARTESIAN_POINT('Ctrl Pts',(92.7857903024108,2.19794896114756,-0.164263953771485));
#16860=CARTESIAN_POINT('Ctrl Pts',(92.7847706303255,2.19648369726788,-0.182815972943825));
#16861=CARTESIAN_POINT('Ctrl Pts',(92.7830562586421,2.1936045862794,-0.214199634368179));
#16862=CARTESIAN_POINT('Ctrl Pts',(92.7823577716966,2.19231267284516,-0.227041226913029));
#16863=CARTESIAN_POINT('Ctrl Pts',(92.7809522101568,2.18947170944573,-0.252989721766818));
#16864=CARTESIAN_POINT('Ctrl Pts',(92.7802453260336,2.18791758036183,-0.266095542551742));
#16865=CARTESIAN_POINT('Ctrl Pts',(92.7785068998949,2.18378482410443,-0.29845817780594));
#16866=CARTESIAN_POINT('Ctrl Pts',(92.7774797131055,2.18106909012312,-0.317696550519678));
#16867=CARTESIAN_POINT('Ctrl Pts',(92.7735562992069,2.1696402348826,-0.391586157752993));
#16868=CARTESIAN_POINT('Ctrl Pts',(92.7707167938676,2.15912407540004,-0.445939836186519));
#16869=CARTESIAN_POINT('Ctrl Pts',(92.7633257056357,2.12586248930158,-0.588781454512491));
#16870=CARTESIAN_POINT('Ctrl Pts',(92.7588713118499,2.09964441200728,-0.676350266198253));
#16871=CARTESIAN_POINT('Ctrl Pts',(92.7475505550456,2.0187950360889,-0.895763048813044));
#16872=CARTESIAN_POINT('Ctrl Pts',(92.7407675123292,1.95667374291665,-1.02437526572849));
#16873=CARTESIAN_POINT('Ctrl Pts',(92.7320167468765,1.868370468802,-1.16942503150712));
#16874=CARTESIAN_POINT('Ctrl Pts',(92.7305878127241,1.85372467846659,-1.19250484156476));
#16875=CARTESIAN_POINT('Ctrl Pts',(92.728560972024,1.83272739442273,-1.22427195733206));
#16876=CARTESIAN_POINT('Ctrl Pts',(92.7279849069519,1.82673524765478,-1.23319497778753));
#16877=CARTESIAN_POINT('Ctrl Pts',(92.7270129250864,1.8165909122042,-1.24806492590057));
#16878=CARTESIAN_POINT('Ctrl Pts',(92.7266193482799,1.81247411146441,-1.25403596259071));
#16879=CARTESIAN_POINT('Ctrl Pts',(92.7258055638006,1.80394563154433,-1.26627600479977));
#16880=CARTESIAN_POINT('Ctrl Pts',(92.7253851438225,1.79953061608079,-1.27254246294123));
#16881=CARTESIAN_POINT('Ctrl Pts',(92.724281735946,1.78791692147766,-1.28884507500649));
#16882=CARTESIAN_POINT('Ctrl Pts',(92.7235953543537,1.78066650987759,-1.2988438364977));
#16883=CARTESIAN_POINT('Ctrl Pts',(92.7204644421927,1.74745581902342,-1.34384266082031));
#16884=CARTESIAN_POINT('Ctrl Pts',(92.7179632571069,1.72054650049254,-1.37812705347092));
#16885=CARTESIAN_POINT('Ctrl Pts',(92.7103854021319,1.63732690310113,-1.47791592766632));
#16886=CARTESIAN_POINT('Ctrl Pts',(92.7052007251412,1.57816478303736,-1.54093136455266));
#16887=CARTESIAN_POINT('Ctrl Pts',(92.690229040135,1.39722180558688,-1.71228071231178));
#16888=CARTESIAN_POINT('Ctrl Pts',(92.6805196466665,1.26691824372134,-1.81081969578041));
#16889=CARTESIAN_POINT('Ctrl Pts',(92.6698386065759,1.10334374869042,-1.9081409224567));
#16890=CARTESIAN_POINT('Ctrl Pts',(92.6683140058262,1.0794972000625,-1.92173231708979));
#16891=CARTESIAN_POINT('Ctrl Pts',(92.6659058619808,1.0410380108242,-1.94271036965767));
#16892=CARTESIAN_POINT('Ctrl Pts',(92.6650121476636,1.02658672266771,-1.95038545974326));
#16893=CARTESIAN_POINT('Ctrl Pts',(92.6634346381087,1.00076506810022,-1.96373284443257));
#16894=CARTESIAN_POINT('Ctrl Pts',(92.6627486111315,0.98942872237785,-1.96946901945875));
#16895=CARTESIAN_POINT('Ctrl Pts',(92.6613205586691,0.965609596319418,-1.98126389235353));
#16896=CARTESIAN_POINT('Ctrl Pts',(92.6605792255044,0.953117900533176,-1.98730339490451));
#16897=CARTESIAN_POINT('Ctrl Pts',(92.6586387337385,0.920092964202268,-2.0028873172942));
#16898=CARTESIAN_POINT('Ctrl Pts',(92.6574464053749,0.899467963614082,-2.01223410698139));
#16899=CARTESIAN_POINT('Ctrl Pts',(92.651553422794,0.79594274369162,-2.05723957426045));
#16900=CARTESIAN_POINT('Ctrl Pts',(92.647016204674,0.711047714751651,-2.08810272223797));
#16901=CARTESIAN_POINT('Ctrl Pts',(92.637963299853,0.534615917547711,-2.14023005865897));
#16902=CARTESIAN_POINT('Ctrl Pts',(92.6334642792863,0.443135930912989,-2.16102517955939));
#16903=CARTESIAN_POINT('Ctrl Pts',(92.6275891962034,0.323378896705407,-2.1803217392013));
#16904=CARTESIAN_POINT('Ctrl Pts',(92.6262499391514,0.296067885881175,-2.18419792439964));
#16905=CARTESIAN_POINT('Ctrl Pts',(92.6205270009926,0.179788234100803,-2.19848021273297));
#16906=CARTESIAN_POINT('Ctrl Pts',(92.6160731731659,0.0903101869764456,
-2.20396913466076));
#16907=CARTESIAN_POINT('Ctrl Pts',(92.6105656608284,-0.0142990247707454,
-2.20400503734064));
#16908=CARTESIAN_POINT('Ctrl Pts',(92.609765741015,-0.0293537274748027,
-2.2038559391864));
#16909=CARTESIAN_POINT('Ctrl Pts',(92.6085097060718,-0.0527485348309028,
-2.20338449432119));
#16910=CARTESIAN_POINT('Ctrl Pts',(92.6080592673582,-0.0610906027192511,
-2.20316898383981));
#16911=CARTESIAN_POINT('Ctrl Pts',(92.6072203564332,-0.0765331441649997,
-2.20268226644223));
#16912=CARTESIAN_POINT('Ctrl Pts',(92.6068326016046,-0.0836337601653857,
-2.20242409146915));
#16913=CARTESIAN_POINT('Ctrl Pts',(92.6059316997565,-0.100046966832361,
-2.20174782888358));
#16914=CARTESIAN_POINT('Ctrl Pts',(92.60541721759,-0.109358250564828,-2.20130499116922));
#16915=CARTESIAN_POINT('Ctrl Pts',(92.6037636372896,-0.13909996275363,-2.19970133201543));
#16916=CARTESIAN_POINT('Ctrl Pts',(92.6026130638315,-0.159516586107941,
-2.19831507005317));
#16917=CARTESIAN_POINT('Ctrl Pts',(92.5962240395545,-0.271574097740623,
-2.18913730628015));
#16918=CARTESIAN_POINT('Ctrl Pts',(92.5907610287505,-0.362671080610185,
-2.17590016885438));
#16919=CARTESIAN_POINT('Ctrl Pts',(92.5753404797683,-0.614474109666137,
-2.12305730906649));
#16920=CARTESIAN_POINT('Ctrl Pts',(92.5653650708357,-0.771971921337889,
-2.07099590966598));
#16921=CARTESIAN_POINT('Ctrl Pts',(92.5534020200614,-0.962649651465769,
-1.98315595359836));
#16922=CARTESIAN_POINT('Ctrl Pts',(92.550901449755,-1.00255169015041,-1.96328612289777));
#16923=CARTESIAN_POINT('Ctrl Pts',(92.5474262739442,-1.05805817806878,-1.93351188016115));
#16924=CARTESIAN_POINT('Ctrl Pts',(92.5464172104109,-1.07418093427552,-1.92460142586598));
#16925=CARTESIAN_POINT('Ctrl Pts',(92.5447153555933,-1.10137638250148,-1.9091232858247));
#16926=CARTESIAN_POINT('Ctrl Pts',(92.5440189054631,-1.11250649825665,-1.90265891782784));
#16927=CARTESIAN_POINT('Ctrl Pts',(92.5426131217319,-1.13497079642317,-1.88934714054745));
#16928=CARTESIAN_POINT('Ctrl Pts',(92.5419040227218,-1.14630117937367,-1.88249434074438));
#16929=CARTESIAN_POINT('Ctrl Pts',(92.5401520797203,-1.17428619620329,-1.86522219484113));
#16930=CARTESIAN_POINT('Ctrl Pts',(92.5391137458381,-1.19086475364906,-1.85468139541838));
#16931=CARTESIAN_POINT('Ctrl Pts',(92.5350873372309,-1.25508385264487,-1.81263415497283));
#16932=CARTESIAN_POINT('Ctrl Pts',(92.53216003712,-1.30163517357271,-1.77950123145934));
#16933=CARTESIAN_POINT('Ctrl Pts',(92.5244525251043,-1.42287635247538,-1.68590151859254));
#16934=CARTESIAN_POINT('Ctrl Pts',(92.519781355041,-1.49498825884334,-1.6222985684472));
#16935=CARTESIAN_POINT('Ctrl Pts',(92.5079801141876,-1.6670423277798,-1.44930005805614));
#16936=CARTESIAN_POINT('Ctrl Pts',(92.5009237560612,-1.76052346655767,-1.33418420393547));
#16937=CARTESIAN_POINT('Ctrl Pts',(92.492196633563,-1.85226066807786,-1.19461787178206));
#16938=CARTESIAN_POINT('Ctrl Pts',(92.4911865964675,-1.86255219363709,-1.17850783590741));
#16939=CARTESIAN_POINT('Ctrl Pts',(92.4896780473303,-1.87741656921542,-1.15455849845753));
#16940=CARTESIAN_POINT('Ctrl Pts',(92.4891896147057,-1.88215290009038,-1.14682115237109));
#16941=CARTESIAN_POINT('Ctrl Pts',(92.4883140808716,-1.89050377867012,-1.13298794576134));
#16942=CARTESIAN_POINT('Ctrl Pts',(92.4879281877325,-1.89413687342042,-1.12690360061047));
#16943=CARTESIAN_POINT('Ctrl Pts',(92.4870734863541,-1.90207869110663,-1.1134565205666));
#16944=CARTESIAN_POINT('Ctrl Pts',(92.4866038715698,-1.90637398503866,-1.10608634134698));
#16945=CARTESIAN_POINT('Ctrl Pts',(92.4852251319747,-1.91879012427482,-1.08449465576655));
#16946=CARTESIAN_POINT('Ctrl Pts',(92.4843091163201,-1.92679520605582,-1.07020764380351));
#16947=CARTESIAN_POINT('Ctrl Pts',(92.4771869694501,-1.98724411408087,-0.959444995656458));
#16948=CARTESIAN_POINT('Ctrl Pts',(92.470633533886,-2.03256660451294,-0.859268598926655));
#16949=CARTESIAN_POINT('Ctrl Pts',(92.4533310409448,-2.1314452370969,-0.588550426358175));
#16950=CARTESIAN_POINT('Ctrl Pts',(92.4426379332962,-2.1720914820329,-0.41411318277556));
#16951=CARTESIAN_POINT('Ctrl Pts',(92.4311841865796,-2.19404988115412,-0.210802711160837));
#16952=CARTESIAN_POINT('Ctrl Pts',(92.4297411883603,-2.19638512628893,-0.184892192079739));
#16953=CARTESIAN_POINT('Ctrl Pts',(92.4274268192586,-2.19942416530005,-0.142861447894437));
#16954=CARTESIAN_POINT('Ctrl Pts',(92.4265467168451,-2.2004105921066,-0.126764734242479));
#16955=CARTESIAN_POINT('Ctrl Pts',(92.4249865997517,-2.20185496766462,-0.0980331544618974));
#16956=CARTESIAN_POINT('Ctrl Pts',(92.4243044815661,-2.20238103161062,-0.0854025696111373));
#16957=CARTESIAN_POINT('Ctrl Pts',(92.4228663666374,-2.20326537717916,-0.0586320688867149));
#16958=CARTESIAN_POINT('Ctrl Pts',(92.4221112573544,-2.20359627333529,-0.0444917821840294));
#16959=CARTESIAN_POINT('Ctrl Pts',(92.4200917293518,-2.20412006431658,-0.00645680217045421));
#16960=CARTESIAN_POINT('Ctrl Pts',(92.4188352133837,-2.20406053916097,0.0174398040700708));
#16961=CARTESIAN_POINT('Ctrl Pts',(92.4116469659395,-2.20147357934064,0.155365518987877));
#16962=CARTESIAN_POINT('Ctrl Pts',(92.4059864301294,-2.1904865573394,0.269066775171342));
#16963=CARTESIAN_POINT('Ctrl Pts',(92.3963620201088,-2.1562810457452,0.46373941959347));
#16964=CARTESIAN_POINT('Ctrl Pts',(92.3923533820206,-2.13714530301353,0.545171569715213));
#16965=CARTESIAN_POINT('Ctrl Pts',(92.3833756488157,-2.08477275793679,0.722178251423084));
#16966=CARTESIAN_POINT('Ctrl Pts',(92.3783911481762,-2.0494925529869,0.816942369086879));
#16967=CARTESIAN_POINT('Ctrl Pts',(92.3722790322138,-2.00160837423168,0.922718036375735));
#16968=CARTESIAN_POINT('Ctrl Pts',(92.3714756925602,-1.99523076279892,0.936428767494364));
#16969=CARTESIAN_POINT('Ctrl Pts',(92.3702154099764,-1.9851091998815,0.95761544869857));
#16970=CARTESIAN_POINT('Ctrl Pts',(92.3697642046487,-1.98146282015777,0.965137798815417));
#16971=CARTESIAN_POINT('Ctrl Pts',(92.3689246429268,-1.97463892634774,0.979013570835433));
#16972=CARTESIAN_POINT('Ctrl Pts',(92.3685370143041,-1.97147339022142,0.985372583592353));
#16973=CARTESIAN_POINT('Ctrl Pts',(92.3676374366787,-1.96409230358272,1.0000219609404));
#16974=CARTESIAN_POINT('Ctrl Pts',(92.3671241665289,-1.95985497638065,1.00830102871188));
#16975=CARTESIAN_POINT('Ctrl Pts',(92.3654784150002,-1.94618130364127,1.03460537817979));
#16976=CARTESIAN_POINT('Ctrl Pts',(92.3643346046839,-1.93654796299813,1.05252642815279));
#16977=CARTESIAN_POINT('Ctrl Pts',(92.3580191343098,-1.88256706276936,1.14969753039784));
#16978=CARTESIAN_POINT('Ctrl Pts',(92.3526281480761,-1.8336048428453,1.22627636476325));
#16979=CARTESIAN_POINT('Ctrl Pts',(92.3374834448696,-1.68456818431785,1.43041052232648));
#16980=CARTESIAN_POINT('Ctrl Pts',(92.3277049785731,-1.57493166587011,1.55030547930311));
#16981=CARTESIAN_POINT('Ctrl Pts',(92.3157044236337,-1.41708671611664,1.6887214811619));
#16982=CARTESIAN_POINT('Ctrl Pts',(92.3130078931126,-1.38001264771135,1.71915112631692));
#16983=CARTESIAN_POINT('Ctrl Pts',(92.3093108689137,-1.32691074219027,1.75991034702617));
#16984=CARTESIAN_POINT('Ctrl Pts',(92.3082698497897,-1.31169912552376,1.77127693579941));
#16985=CARTESIAN_POINT('Ctrl Pts',(92.3065943744804,-1.28679956838745,1.78938595558961));
#16986=CARTESIAN_POINT('Ctrl Pts',(92.3059552414593,-1.2772012594229,1.79624947537518));
#16987=CARTESIAN_POINT('Ctrl Pts',(92.3046222458572,-1.25697483961603,1.81046880644041));
#16988=CARTESIAN_POINT('Ctrl Pts',(92.3039290011311,-1.24633618807167,1.81780889057594));
#16989=CARTESIAN_POINT('Ctrl Pts',(92.3022782017456,-1.22072012287885,1.83515196518747));
#16990=CARTESIAN_POINT('Ctrl Pts',(92.3013240267401,-1.20568333809347,1.84506587085693));
#16991=CARTESIAN_POINT('Ctrl Pts',(92.2980108198246,-1.1526844936187,1.87908393729929));
#16992=CARTESIAN_POINT('Ctrl Pts',(92.2956876417274,-1.11410661619497,1.90221050190376));
#16993=CARTESIAN_POINT('Ctrl Pts',(92.2899944942639,-1.01639330839061,1.95679421183827));
#16994=CARTESIAN_POINT('Ctrl Pts',(92.2866718568686,-0.956480355202978,
1.98676749736706));
#16995=CARTESIAN_POINT('Ctrl Pts',(92.277790410745,-0.79069248943156,2.06046713781154));
#16996=CARTESIAN_POINT('Ctrl Pts',(92.2723379247909,-0.682631086942057,
2.09874570079143));
#16997=CARTESIAN_POINT('Ctrl Pts',(92.2635807017027,-0.509891923156279,
2.14517457413493));
#16998=CARTESIAN_POINT('Ctrl Pts',(92.2603814935311,-0.446997420984935,
2.15915631174931));
#16999=CARTESIAN_POINT('Ctrl Pts',(92.2556018353007,-0.355505543634313,
2.17532639451038));
#17000=CARTESIAN_POINT('Ctrl Pts',(92.2541130197628,-0.32733317341784,2.17974355348617));
#17001=CARTESIAN_POINT('Ctrl Pts',(92.2520145308062,-0.288251538248025,
2.18509647440409));
#17002=CARTESIAN_POINT('Ctrl Pts',(92.2514287732939,-0.277408041027634,
2.18649955877926));
#17003=CARTESIAN_POINT('Ctrl Pts',(92.2504806093252,-0.259971924181495,
2.18862390005417));
#17004=CARTESIAN_POINT('Ctrl Pts',(92.2501210116239,-0.253385570763207,
2.1893962015553));
#17005=CARTESIAN_POINT('Ctrl Pts',(92.2493988040727,-0.240213485565602,
2.1908804987964));
#17006=CARTESIAN_POINT('Ctrl Pts',(92.2490361988305,-0.233627846944208,
2.1915925499295));
#17007=CARTESIAN_POINT('Ctrl Pts',(92.2482646760888,-0.219671376636344,
2.19303792794988));
#17008=CARTESIAN_POINT('Ctrl Pts',(92.2478553565435,-0.212299854477745,
2.19376380581684));
#17009=CARTESIAN_POINT('Ctrl Pts',(92.2468683636488,-0.194599233684011,
2.19541674582902));
#17010=CARTESIAN_POINT('Ctrl Pts',(92.2462888684194,-0.18426706517281,2.19630808176313));
#17011=CARTESIAN_POINT('Ctrl Pts',(92.2424670889475,-0.116489477121162,
2.20167349948885));
#17012=CARTESIAN_POINT('Ctrl Pts',(92.2391242511364,-0.058897880036256,
2.20396596668738));
#17013=CARTESIAN_POINT('Ctrl Pts',(92.2357268140388,-0.00128762525293467,
2.20399962387048));
#17014=CARTESIAN_POINT('Ctrl Pts',(92.2357268613305,-0.00128842717656291,
2.20399962340183));
#17015=CARTESIAN_POINT('Ctrl Pts',(92.2357015338201,-0.000858949161186015,
2.20399987446864));
#17016=CARTESIAN_POINT('Ctrl Pts',(92.2356762034427,-0.000429473425876918,
2.204));
#17017=CARTESIAN_POINT('Ctrl Pts',(92.2356508702176,-2.51612300885953E-11,
2.204));
#17018=CARTESIAN_POINT('',(92.1243948225064,-0.00126182935173377,2.20399987870527));
#17019=CARTESIAN_POINT('Ctrl Pts',(92.1243308360554,1.24847509279933E-11,
2.204));
#17020=CARTESIAN_POINT('Ctrl Pts',(92.1243520093957,-0.000420349403778188,
2.204));
#17021=CARTESIAN_POINT('Ctrl Pts',(92.1243731866753,-0.000840700810317714,
2.20399987974572));
#17022=CARTESIAN_POINT('Ctrl Pts',(92.1243943679136,-0.00126105415559237,
2.20399963923373));
#17023=CARTESIAN_POINT('Ctrl Pts',(92.1243944080205,-0.00126185009846303,
2.20399963877818));
#17024=CARTESIAN_POINT('Ctrl Pts',(92.1259360221631,-0.0318560252145767,
2.20398212277581));
#17025=CARTESIAN_POINT('Ctrl Pts',(92.1274978250993,-0.0624453826648012,
2.20332758254774));
#17026=CARTESIAN_POINT('Ctrl Pts',(92.1300489761317,-0.111503091054167,
2.20125547486973));
#17027=CARTESIAN_POINT('Ctrl Pts',(92.1310206936636,-0.129985052916093,
2.20024145237313));
#17028=CARTESIAN_POINT('Ctrl Pts',(92.1324632420578,-0.157072999238677,
2.19841277798702));
#17029=CARTESIAN_POINT('Ctrl Pts',(92.1329249119006,-0.165690890354302,
2.19778006031472));
#17030=CARTESIAN_POINT('Ctrl Pts',(92.1337572455189,-0.181129958988984,
2.19655521563871));
#17031=CARTESIAN_POINT('Ctrl Pts',(92.1341268966739,-0.187952566928249,
2.195981946057));
#17032=CARTESIAN_POINT('Ctrl Pts',(92.1348865159491,-0.201899683140805,
2.19474456768884));
#17033=CARTESIAN_POINT('Ctrl Pts',(92.1352766593163,-0.209023631101947,
2.19407755500457));
#17034=CARTESIAN_POINT('Ctrl Pts',(92.1361663608094,-0.225180764304435,
2.19248536478043));
#17035=CARTESIAN_POINT('Ctrl Pts',(92.1366670565733,-0.234211516058069,
2.19153905079146));
#17036=CARTESIAN_POINT('Ctrl Pts',(92.1382176937927,-0.261999662312857,
2.18845347062796));
#17037=CARTESIAN_POINT('Ctrl Pts',(92.1392771739789,-0.280735152572016,
2.18612903131721));
#17038=CARTESIAN_POINT('Ctrl Pts',(92.1438518035719,-0.360689571814189,
2.17516467516825));
#17039=CARTESIAN_POINT('Ctrl Pts',(92.1474675623071,-0.421556483211142,
2.16419207368789));
#17040=CARTESIAN_POINT('Ctrl Pts',(92.1588422795101,-0.608655046215802,
2.12227110613759));
#17041=CARTESIAN_POINT('Ctrl Pts',(92.1667394077557,-0.73267452599131,2.08271112846419));
#17042=CARTESIAN_POINT('Ctrl Pts',(92.1784325303129,-0.91494340669467,2.00626046433122));
#17043=CARTESIAN_POINT('Ctrl Pts',(92.1823797112768,-0.976158938583549,
1.97719938401971));
#17044=CARTESIAN_POINT('Ctrl Pts',(92.1880017006623,-1.06323302823782,1.93083077051992));
#17045=CARTESIAN_POINT('Ctrl Pts',(92.1897451893135,-1.09021510586326,1.91572521335551));
#17046=CARTESIAN_POINT('Ctrl Pts',(92.1928756481769,-1.13862301878099,1.88727057703892));
#17047=CARTESIAN_POINT('Ctrl Pts',(92.1942689731587,-1.16015407832838,1.87411184274326));
#17048=CARTESIAN_POINT('Ctrl Pts',(92.1964427904054,-1.1937119560621,1.852802896066));
#17049=CARTESIAN_POINT('Ctrl Pts',(92.1972322556332,-1.20589181141834,1.84489884792334));
#17050=CARTESIAN_POINT('Ctrl Pts',(92.1987057086537,-1.22860611343567,1.8298374747043));
#17051=CARTESIAN_POINT('Ctrl Pts',(92.1993907028663,-1.23915830324513,1.82270811562217));
#17052=CARTESIAN_POINT('Ctrl Pts',(92.2009245850578,-1.26276616081912,1.80645820106223));
#17053=CARTESIAN_POINT('Ctrl Pts',(92.2017714931534,-1.27578602985604,1.79728674205346));
#17054=CARTESIAN_POINT('Ctrl Pts',(92.2042567544561,-1.31393514562192,1.76979028153189));
#17055=CARTESIAN_POINT('Ctrl Pts',(92.2058799901889,-1.33877773858901,1.75107324232102));
#17056=CARTESIAN_POINT('Ctrl Pts',(92.2145873774472,-1.47138554872632,1.64669085357318));
#17057=CARTESIAN_POINT('Ctrl Pts',(92.2212827303238,-1.5713460582974,1.55159348236101));
#17058=CARTESIAN_POINT('Ctrl Pts',(92.2329681421634,-1.7301303783204,1.36933931830502));
#17059=CARTESIAN_POINT('Ctrl Pts',(92.2379688032933,-1.79283173979382,1.28615442069662));
#17060=CARTESIAN_POINT('Ctrl Pts',(92.2448386934838,-1.86713670133269,1.17152779623565));
#17061=CARTESIAN_POINT('Ctrl Pts',(92.2464989613227,-1.88424458565701,1.14380898826709));
#17062=CARTESIAN_POINT('Ctrl Pts',(92.2493660199057,-1.91218864747155,1.09620382574241));
#17063=CARTESIAN_POINT('Ctrl Pts',(92.2505564758016,-1.92334427413485,1.07651055534892));
#17064=CARTESIAN_POINT('Ctrl Pts',(92.2522860967265,-1.93887346540725,1.0480844171766));
#17065=CARTESIAN_POINT('Ctrl Pts',(92.2528105921555,-1.94349567256291,1.03948825095711));
#17066=CARTESIAN_POINT('Ctrl Pts',(92.2537291095489,-1.95143575171012,1.02448356806266));
#17067=CARTESIAN_POINT('Ctrl Pts',(92.254121508006,-1.95477948130486,1.01808902008186));
#17068=CARTESIAN_POINT('Ctrl Pts',(92.2549656211302,-1.96186814439548,1.00436898877901));
#17069=CARTESIAN_POINT('Ctrl Pts',(92.2554178774834,-1.96560342491157,0.997039042900629));
#17070=CARTESIAN_POINT('Ctrl Pts',(92.2566634879079,-1.97572350604232,0.976901948201957));
#17071=CARTESIAN_POINT('Ctrl Pts',(92.2574617242342,-1.9820246380984,0.964053473970097));
#17072=CARTESIAN_POINT('Ctrl Pts',(92.2619328683899,-2.01633511436113,0.89233349753733));
#17073=CARTESIAN_POINT('Ctrl Pts',(92.2657315141812,-2.04184463156987,0.832307306234299));
#17074=CARTESIAN_POINT('Ctrl Pts',(92.2776291130239,-2.11215097181134,0.64409423739175));
#17075=CARTESIAN_POINT('Ctrl Pts',(92.2858890129141,-2.14780109517018,0.51282732590043));
#17076=CARTESIAN_POINT('Ctrl Pts',(92.2998360268757,-2.18838459773861,0.280407187679906));
#17077=CARTESIAN_POINT('Ctrl Pts',(92.3056197596986,-2.19887030664066,0.180634844817134));
#17078=CARTESIAN_POINT('Ctrl Pts',(92.3124929664486,-2.20338392659665,0.0571149444333545));
#17079=CARTESIAN_POINT('Ctrl Pts',(92.3137818374172,-2.20386591726108,0.0337331161833779));
#17080=CARTESIAN_POINT('Ctrl Pts',(92.3158305365386,-2.20404202072537,-0.00377662077893416));
#17081=CARTESIAN_POINT('Ctrl Pts',(92.3165976868249,-2.20397256185814,-0.0179011626142755));
#17082=CARTESIAN_POINT('Ctrl Pts',(92.3180522176951,-2.20358127573999,-0.0448277041222772));
#17083=CARTESIAN_POINT('Ctrl Pts',(92.3187403257175,-2.20328364503262,-0.0576294280264321));
#17084=CARTESIAN_POINT('Ctrl Pts',(92.3202974585982,-2.20235301657398,-0.0867379788831724));
#17085=CARTESIAN_POINT('Ctrl Pts',(92.3211642726723,-2.20165044171183,-0.103041925719591));
#17086=CARTESIAN_POINT('Ctrl Pts',(92.323450364999,-2.19930521628583,-0.146291714071161));
#17087=CARTESIAN_POINT('Ctrl Pts',(92.3248598702747,-2.19734846081747,-0.173218140589351));
#17088=CARTESIAN_POINT('Ctrl Pts',(92.3366407252715,-2.17665637532275,-0.400186715694862));
#17089=CARTESIAN_POINT('Ctrl Pts',(92.346077812492,-2.13114630735586,-0.596823283658799));
#17090=CARTESIAN_POINT('Ctrl Pts',(92.3598546797665,-2.0308419927588,-0.860136345621305));
#17091=CARTESIAN_POINT('Ctrl Pts',(92.3638754506865,-1.99792506500616,-0.934048664990639));
#17092=CARTESIAN_POINT('Ctrl Pts',(92.3691090323471,-1.95218848187927,-1.02320624535878));
#17093=CARTESIAN_POINT('Ctrl Pts',(92.3701316843765,-1.94312466105778,-1.04031600504733));
#17094=CARTESIAN_POINT('Ctrl Pts',(92.3716584436675,-1.92943678936706,-1.06535149430467));
#17095=CARTESIAN_POINT('Ctrl Pts',(92.3721522105306,-1.92498654724541,-1.07337175173908));
#17096=CARTESIAN_POINT('Ctrl Pts',(92.3729999175782,-1.91731010568671,-1.08700500015952));
#17097=CARTESIAN_POINT('Ctrl Pts',(92.3733522627422,-1.91410904060029,-1.09263191026518));
#17098=CARTESIAN_POINT('Ctrl Pts',(92.3741613207157,-1.90673587928723,-1.10546078959782));
#17099=CARTESIAN_POINT('Ctrl Pts',(92.3746190344808,-1.90254783736073,-1.11265313219333));
#17100=CARTESIAN_POINT('Ctrl Pts',(92.3758940169671,-1.89083218626658,-1.13251348188617));
#17101=CARTESIAN_POINT('Ctrl Pts',(92.376716536809,-1.88321824754322,-1.14512975310402));
#17102=CARTESIAN_POINT('Ctrl Pts',(92.3816678300496,-1.83701300535474,-1.21998447349178));
#17103=CARTESIAN_POINT('Ctrl Pts',(92.3859548896681,-1.79546863117158,-1.28033957112359));
#17104=CARTESIAN_POINT('Ctrl Pts',(92.39789157381,-1.67352711280962,-1.43986017308734));
#17105=CARTESIAN_POINT('Ctrl Pts',(92.4056397829112,-1.58739416654353,-1.53429862117625));
#17106=CARTESIAN_POINT('Ctrl Pts',(92.4190658044793,-1.42032868681611,-1.68825467241441));
#17107=CARTESIAN_POINT('Ctrl Pts',(92.4248139314163,-1.34258318875831,-1.75071755643439));
#17108=CARTESIAN_POINT('Ctrl Pts',(92.4316521798041,-1.241715934637,-1.82107189948996));
#17109=CARTESIAN_POINT('Ctrl Pts',(92.4329392134088,-1.22235094164076,-1.83412637519782));
#17110=CARTESIAN_POINT('Ctrl Pts',(92.4349857090026,-1.19095189540914,-1.85457512064807));
#17111=CARTESIAN_POINT('Ctrl Pts',(92.4357524652561,-1.1790482674256,-1.86216553813707));
#17112=CARTESIAN_POINT('Ctrl Pts',(92.4372066884223,-1.15620864164595,-1.87642254933051));
#17113=CARTESIAN_POINT('Ctrl Pts',(92.437894877631,-1.14528589758854,-1.88310919201072));
#17114=CARTESIAN_POINT('Ctrl Pts',(92.4394527825923,-1.12030273312725,-1.89810550430086));
#17115=CARTESIAN_POINT('Ctrl Pts',(92.4403202793104,-1.10620690207326,-1.90635490623168));
#17116=CARTESIAN_POINT('Ctrl Pts',(92.4430440524502,-1.06137952753207,-1.93192490511823));
#17117=CARTESIAN_POINT('Ctrl Pts',(92.4448796432446,-1.03032244091916,-1.94866523271354));
#17118=CARTESIAN_POINT('Ctrl Pts',(92.4557216018491,-0.842192626441297,
-2.04431482303175));
#17119=CARTESIAN_POINT('Ctrl Pts',(92.4640675978479,-0.676548511763246,
-2.10494572099715));
#17120=CARTESIAN_POINT('Ctrl Pts',(92.4772388693823,-0.412688936544367,
-2.16711488874979));
#17121=CARTESIAN_POINT('Ctrl Pts',(92.481927782874,-0.318611853834009,-2.18292973534898));
#17122=CARTESIAN_POINT('Ctrl Pts',(92.4879789158816,-0.203047280456454,
-2.19472633107972));
#17123=CARTESIAN_POINT('Ctrl Pts',(92.4890794242496,-0.182249458261284,
-2.19655114642823));
#17124=CARTESIAN_POINT('Ctrl Pts',(92.4907005858738,-0.152002880936595,
-2.19877249090341));
#17125=CARTESIAN_POINT('Ctrl Pts',(92.4912089806292,-0.142571967361765,
-2.19940413977913));
#17126=CARTESIAN_POINT('Ctrl Pts',(92.4921060840201,-0.126033420959466,
-2.20040501475885));
#17127=CARTESIAN_POINT('Ctrl Pts',(92.4924933360493,-0.118927639343395,
-2.20080050604638));
#17128=CARTESIAN_POINT('Ctrl Pts',(92.4933412698498,-0.103443247750162,
-2.20158711917442));
#17129=CARTESIAN_POINT('Ctrl Pts',(92.4938026491174,-0.0950644096843052,
-2.20196482761502));
#17130=CARTESIAN_POINT('Ctrl Pts',(92.4950974853735,-0.0716717406611916,
-2.20288557840956));
#17131=CARTESIAN_POINT('Ctrl Pts',(92.4959364494406,-0.056654484276065,
-2.20332293458561));
#17132=CARTESIAN_POINT('Ctrl Pts',(92.5015412717844,0.0428487503805245,
-2.20520292228096));
#17133=CARTESIAN_POINT('Ctrl Pts',(92.5065177207575,0.127346452643196,-2.20193919230552));
#17134=CARTESIAN_POINT('Ctrl Pts',(92.5134635695193,0.243156214577335,-2.19077756755995));
#17135=CARTESIAN_POINT('Ctrl Pts',(92.5153749179594,0.274802606981332,-2.18703332863539));
#17136=CARTESIAN_POINT('Ctrl Pts',(92.5228252200121,0.397649971600758,-2.16979013569201));
#17137=CARTESIAN_POINT('Ctrl Pts',(92.5283692401964,0.488053878794831,-2.15126000416897));
#17138=CARTESIAN_POINT('Ctrl Pts',(92.5392243809405,0.665981258996695,-2.10299279767138));
#17139=CARTESIAN_POINT('Ctrl Pts',(92.5445247469296,0.753334519271191,-2.07330658230774));
#17140=CARTESIAN_POINT('Ctrl Pts',(92.5509200340969,0.859765848346851,-2.02951803232778));
#17141=CARTESIAN_POINT('Ctrl Pts',(92.5521819456515,0.880813883539689,-2.02047215176543));
#17142=CARTESIAN_POINT('Ctrl Pts',(92.554198290323,0.914512121573808,-2.00536285679522));
#17143=CARTESIAN_POINT('Ctrl Pts',(92.5549596411075,0.927251761732526,-1.99950413629387));
#17144=CARTESIAN_POINT('Ctrl Pts',(92.5564097235289,0.951541478150501,-1.98805167874642));
#17145=CARTESIAN_POINT('Ctrl Pts',(92.55709910629,0.963100271670365,-1.98247787840536));
#17146=CARTESIAN_POINT('Ctrl Pts',(92.5586680173806,0.989426766877393,-1.96949830576375));
#17147=CARTESIAN_POINT('Ctrl Pts',(92.559545209038,1.00416129508404,-1.96202676254249));
#17148=CARTESIAN_POINT('Ctrl Pts',(92.5618784290095,1.04337853530288,-1.94158307338858));
#17149=CARTESIAN_POINT('Ctrl Pts',(92.563324009837,1.06770335515914,-1.92831357229155));
#17150=CARTESIAN_POINT('Ctrl Pts',(92.5730185367437,1.2307808021807,-1.83532052139995));
#17151=CARTESIAN_POINT('Ctrl Pts',(92.5807141111319,1.3607433410048,-1.74115056363579));
#17152=CARTESIAN_POINT('Ctrl Pts',(92.5945655181774,1.57304189210383,-1.54891050962903));
#17153=CARTESIAN_POINT('Ctrl Pts',(92.6006958734549,1.65923325915252,-1.45620122665279));
#17154=CARTESIAN_POINT('Ctrl Pts',(92.6081644098687,1.74662289606223,-1.34430985196332));
#17155=CARTESIAN_POINT('Ctrl Pts',(92.6089948028617,1.7561163470124,-1.33188432954069));
#17156=CARTESIAN_POINT('Ctrl Pts',(92.6102863273112,1.77052140091805,-1.31260846873266));
#17157=CARTESIAN_POINT('Ctrl Pts',(92.6107411911895,1.77552744689428,-1.30582897189404));
#17158=CARTESIAN_POINT('Ctrl Pts',(92.6115885916867,1.78472598476277,-1.29322105823049));
#17159=CARTESIAN_POINT('Ctrl Pts',(92.6119803990189,1.78892902163402,-1.28740067461467));
#17160=CARTESIAN_POINT('Ctrl Pts',(92.6128828482631,1.79849649270917,-1.27401428005548));
#17161=CARTESIAN_POINT('Ctrl Pts',(92.6133947519263,1.80384167105459,-1.2664348540236));
#17162=CARTESIAN_POINT('Ctrl Pts',(92.6150448966668,1.82081775272028,-1.24203737307254));
#17163=CARTESIAN_POINT('Ctrl Pts',(92.6161946205806,1.8322621829349,-1.22509157070617));
#17164=CARTESIAN_POINT('Ctrl Pts',(92.6246065749992,1.91339688550704,-1.10127487111994));
#17165=CARTESIAN_POINT('Ctrl Pts',(92.6323010488496,1.97392167387891,-0.988697418926266));
#17166=CARTESIAN_POINT('Ctrl Pts',(92.6464846523659,2.06730213973287,-0.771795272521114));
#17167=CARTESIAN_POINT('Ctrl Pts',(92.652965112083,2.10281332490698,-0.669018632201595));
#17168=CARTESIAN_POINT('Ctrl Pts',(92.6627936131404,2.14636212546737,-0.504516092641967));
#17169=CARTESIAN_POINT('Ctrl Pts',(92.6662809413301,2.15961876363449,-0.444358752015239));
#17170=CARTESIAN_POINT('Ctrl Pts',(92.6708113377272,2.17387050670267,-0.363750332766872));
#17171=CARTESIAN_POINT('Ctrl Pts',(92.6719250188061,2.17712559513296,-0.343731677864219));
#17172=CARTESIAN_POINT('Ctrl Pts',(92.6737635189982,2.18208129385619,-0.310352238161295));
#17173=CARTESIAN_POINT('Ctrl Pts',(92.6744931859176,2.18393653878344,-0.297015976982417));
#17174=CARTESIAN_POINT('Ctrl Pts',(92.6759164668106,2.18733474312018,-0.270832292048455));
#17175=CARTESIAN_POINT('Ctrl Pts',(92.6766103474876,2.1888870024233,-0.257986645701906));
#17176=CARTESIAN_POINT('Ctrl Pts',(92.6782752408913,2.19235753304524,-0.226975919143379));
#17177=CARTESIAN_POINT('Ctrl Pts',(92.6792426845291,2.19416330339933,-0.208799055321895));
#17178=CARTESIAN_POINT('Ctrl Pts',(92.6824448665742,2.19942898908688,-0.148137968185167));
#17179=CARTESIAN_POINT('Ctrl Pts',(92.6846483395663,2.2018826010158,-0.105574880363342));
#17180=CARTESIAN_POINT('Ctrl Pts',(92.6953295990619,2.20787385170795,0.104053105674433));
#17181=CARTESIAN_POINT('Ctrl Pts',(92.7032559255081,2.19364040370517,0.271067532739719));
#17182=CARTESIAN_POINT('Ctrl Pts',(92.7158806168465,2.14242445694557,0.525533394984517));
#17183=CARTESIAN_POINT('Ctrl Pts',(92.7204396682846,2.11849156300855,0.614945750728927));
#17184=CARTESIAN_POINT('Ctrl Pts',(92.726331656623,2.08245227150757,0.722102984280509));
#17185=CARTESIAN_POINT('Ctrl Pts',(92.7274177064101,2.07561378465311,0.741530538680626));
#17186=CARTESIAN_POINT('Ctrl Pts',(92.7290213738526,2.0652588807805,0.769681840633855));
#17187=CARTESIAN_POINT('Ctrl Pts',(92.7295271010154,2.06195710450873,0.778483958151378));
#17188=CARTESIAN_POINT('Ctrl Pts',(92.7304212743774,2.05605879659927,0.793907302540494));
#17189=CARTESIAN_POINT('Ctrl Pts',(92.7308082972785,2.05348638546817,0.800537471534418));
#17190=CARTESIAN_POINT('Ctrl Pts',(92.7316579192573,2.04779767194742,0.814991790290467));
#17191=CARTESIAN_POINT('Ctrl Pts',(92.73212124037,2.04466864826521,0.82281045049415));
#17192=CARTESIAN_POINT('Ctrl Pts',(92.7334266378054,2.03577530029283,0.844668730947752));
#17193=CARTESIAN_POINT('Ctrl Pts',(92.7342743595535,2.02991076175273,0.858666763991459));
#17194=CARTESIAN_POINT('Ctrl Pts',(92.7402484158178,1.98792546895196,0.956046854019381));
#17195=CARTESIAN_POINT('Ctrl Pts',(92.7456178323101,1.94682567532868,1.0371788550614));
#17196=CARTESIAN_POINT('Ctrl Pts',(92.7524115566793,1.88933611209746,1.13513954124702));
#17197=CARTESIAN_POINT('Ctrl Pts',(92.7537750576747,1.87752821808702,1.15456506907185));
#17198=CARTESIAN_POINT('Ctrl Pts',(92.7604333567593,1.81847249629876,1.24841703644602));
#17199=CARTESIAN_POINT('Ctrl Pts',(92.7657382384729,1.76708684015812,1.32014868740261));
#17200=CARTESIAN_POINT('Ctrl Pts',(92.7747892184596,1.67052047249218,1.43917213770966));
#17201=CARTESIAN_POINT('Ctrl Pts',(92.7785769157666,1.62727698152837,1.48789307032024));
#17202=CARTESIAN_POINT('Ctrl Pts',(92.7847978182065,1.55118258533804,1.56633311745049));
#17203=CARTESIAN_POINT('Ctrl Pts',(92.7872737206403,1.51948099481991,1.59710511500307));
#17204=CARTESIAN_POINT('Ctrl Pts',(92.7907005704363,1.47359114764053,1.63904513347379));
#17205=CARTESIAN_POINT('Ctrl Pts',(92.7916856117272,1.46015950912441,1.6510221243255));
#17206=CARTESIAN_POINT('Ctrl Pts',(92.7933714842882,1.43675916087808,1.67137926254787));
#17207=CARTESIAN_POINT('Ctrl Pts',(92.7940755631496,1.42686024185909,1.67983790468767));
#17208=CARTESIAN_POINT('Ctrl Pts',(92.7955061254174,1.40649193239773,1.6969327063139));
#17209=CARTESIAN_POINT('Ctrl Pts',(92.796232266774,1.39601655870108,1.7055608886279));
#17210=CARTESIAN_POINT('Ctrl Pts',(92.7980611003176,1.36929206435639,1.72716169733097));
#17211=CARTESIAN_POINT('Ctrl Pts',(92.7991584857871,1.35293765204394,1.74000230895858));
#17212=CARTESIAN_POINT('Ctrl Pts',(92.8034198971075,1.28821659860586,1.78935353665396));
#17213=CARTESIAN_POINT('Ctrl Pts',(92.8065156126625,1.23853250913716,1.82409597482429));
#17214=CARTESIAN_POINT('Ctrl Pts',(92.8170834000714,1.0609482574718,1.93766931496357));
#17215=CARTESIAN_POINT('Ctrl Pts',(92.8242035545896,0.92648391386854,2.00544295858634));
#17216=CARTESIAN_POINT('Ctrl Pts',(92.8361302074394,0.697959112408725,2.09269797525605));
#17217=CARTESIAN_POINT('Ctrl Pts',(92.8408111338332,0.607682531550858,2.12067207029121));
#17218=CARTESIAN_POINT('Ctrl Pts',(92.8465790745721,0.50119742658519,2.14630982798855));
#17219=CARTESIAN_POINT('Ctrl Pts',(92.8473828885217,0.486457857147284,2.14969845937399));
#17220=CARTESIAN_POINT('Ctrl Pts',(92.8486416764787,0.463558845433109,2.15471538740191));
#17221=CARTESIAN_POINT('Ctrl Pts',(92.8490908725455,0.45542282106395,2.15644968717707));
#17222=CARTESIAN_POINT('Ctrl Pts',(92.849933637424,0.440229947525869,2.15959843301897));
#17223=CARTESIAN_POINT('Ctrl Pts',(92.8503265557052,0.433175763365217,2.1610244217896));
#17224=CARTESIAN_POINT('Ctrl Pts',(92.8512392542547,0.416855141835998,2.16424048130748));
#17225=CARTESIAN_POINT('Ctrl Pts',(92.8517604018492,0.407584055186156,2.16600560975387));
#17226=CARTESIAN_POINT('Ctrl Pts',(92.8534268139649,0.378079127532255,2.17142693846586));
#17227=CARTESIAN_POINT('Ctrl Pts',(92.8545835735802,0.357805879830048,2.17485945896453));
#17228=CARTESIAN_POINT('Ctrl Pts',(92.86214101456,0.2264544342756,2.19521273006672));
#17229=CARTESIAN_POINT('Ctrl Pts',(92.8688761504706,0.11427588574401,2.20390054763915));
#17230=CARTESIAN_POINT('Ctrl Pts',(92.875663664803,0.00128964400580923,
2.20399971703118));
#17231=CARTESIAN_POINT('Ctrl Pts',(92.8757024023764,0.000644818249044074,
2.20399999999996));
#17232=CARTESIAN_POINT('Ctrl Pts',(92.8757411398941,1.22339489286472E-10,
2.204));
#17233=CARTESIAN_POINT('Origin',(66.9212607628943,0.,0.));
#17234=CARTESIAN_POINT('',(93.7322127872898,-1.52555169845894E-15,2.204));
#17235=CARTESIAN_POINT('',(93.6281258142613,1.15214847468432E-14,2.204));
#17236=CARTESIAN_POINT('',(66.9212607628943,-2.69912154532077E-16,2.204));
#17237=CARTESIAN_POINT('',(93.7322042748184,0.000170073928470324,2.20399969046683));
#17238=CARTESIAN_POINT('Ctrl Pts',(93.7322127872898,-1.52555169845894E-15,
2.204));
#17239=CARTESIAN_POINT('Ctrl Pts',(93.7322097718937,5.67412332685096E-5,
2.204));
#17240=CARTESIAN_POINT('Ctrl Pts',(93.732206756565,0.000113482473413851,
2.20399999780882));
#17241=CARTESIAN_POINT('Ctrl Pts',(93.7322037413037,0.000170223720302068,
2.20399999342647));
#17242=CARTESIAN_POINT('Ctrl Pts',(93.7322037507425,0.000170046101699417,
2.20399999344018));
#17243=CARTESIAN_POINT('Ctrl Pts',(93.7311627020912,0.019760519554234,2.20399848196847));
#17244=CARTESIAN_POINT('Ctrl Pts',(93.7301297689015,0.0393505287422103,
2.20373577308858));
#17245=CARTESIAN_POINT('Ctrl Pts',(93.7273906911225,0.0916756679353474,
2.20233610000477));
#17246=CARTESIAN_POINT('Ctrl Pts',(93.7256988646687,0.12439382954957,2.20073056969929));
#17247=CARTESIAN_POINT('Ctrl Pts',(93.7141567735045,0.349874654399729,2.18462101571674));
#17248=CARTESIAN_POINT('Ctrl Pts',(93.7051076533056,0.540019923774952,2.14554366317177));
#17249=CARTESIAN_POINT('Ctrl Pts',(93.6929682032714,0.773520450323089,2.06450571506348));
#17250=CARTESIAN_POINT('Ctrl Pts',(93.6902857141559,0.823743286802514,2.04498511298578));
#17251=CARTESIAN_POINT('Ctrl Pts',(93.6864030017052,0.893345757848016,2.01495183127093));
#17252=CARTESIAN_POINT('Ctrl Pts',(93.6852665889057,0.913362168797062,2.00595787864736));
#17253=CARTESIAN_POINT('Ctrl Pts',(93.6832358187998,0.948413873538154,1.98957474364813));
#17254=CARTESIAN_POINT('Ctrl Pts',(93.6823478957235,0.963505675530331,1.98231009576007));
#17255=CARTESIAN_POINT('Ctrl Pts',(93.6809884392729,0.986224756900104,1.97105322225954));
#17256=CARTESIAN_POINT('Ctrl Pts',(93.6805243255696,0.993914174789823,1.96718699776744));
#17257=CARTESIAN_POINT('Ctrl Pts',(93.679673151206,1.00788950253193,1.96005737457327));
#17258=CARTESIAN_POINT('Ctrl Pts',(93.6792869892997,1.01418256100026,1.95680859827848));
#17259=CARTESIAN_POINT('Ctrl Pts',(93.6784067901617,1.02842008709858,1.94937138051269));
#17260=CARTESIAN_POINT('Ctrl Pts',(93.6779116424099,1.03635464206135,1.94516469862781));
#17261=CARTESIAN_POINT('Ctrl Pts',(93.6763801141125,1.06067715312717,1.93207851481566));
#17262=CARTESIAN_POINT('Ctrl Pts',(93.6753344342274,1.07697795162622,1.92303974356451));
#17263=CARTESIAN_POINT('Ctrl Pts',(93.6656452355125,1.22546184882725,1.8382256234807));
#17264=CARTESIAN_POINT('Ctrl Pts',(93.656373714362,1.34956102328693,1.74914557214675));
#17265=CARTESIAN_POINT('Ctrl Pts',(93.6401175890809,1.55251973689422,1.56891067381643));
#17266=CARTESIAN_POINT('Ctrl Pts',(93.6330965682512,1.63501923341314,1.4827395436678));
#17267=CARTESIAN_POINT('Ctrl Pts',(93.6242513395088,1.73370478225863,1.36135116094821));
#17268=CARTESIAN_POINT('Ctrl Pts',(93.6221689880822,1.75651212768382,1.33179376797084));
#17269=CARTESIAN_POINT('Ctrl Pts',(93.6191934608053,1.78846544041769,1.28813382031447));
#17270=CARTESIAN_POINT('Ctrl Pts',(93.618276937348,1.79821746453001,1.27448473620757));
#17271=CARTESIAN_POINT('Ctrl Pts',(93.6166757904982,1.81509062968977,1.25028951781281));
#17272=CARTESIAN_POINT('Ctrl Pts',(93.6159886556115,1.8222779508952,1.23979068858649));
#17273=CARTESIAN_POINT('Ctrl Pts',(93.6145626135252,1.83707876191197,1.21776371347906));
#17274=CARTESIAN_POINT('Ctrl Pts',(93.6138243531795,1.844675599282,1.20622501410989));
#17275=CARTESIAN_POINT('Ctrl Pts',(93.6119015160732,1.86428448747864,1.17582287273593));
#17276=CARTESIAN_POINT('Ctrl Pts',(93.6107235384816,1.87611896963305,1.15684646285209));
#17277=CARTESIAN_POINT('Ctrl Pts',(93.6055521900641,1.92723226181816,1.07203915008598));
#17278=CARTESIAN_POINT('Ctrl Pts',(93.6016727659889,1.96335155688039,1.0043626424015));
#17279=CARTESIAN_POINT('Ctrl Pts',(93.5909362786264,2.05523820865861,0.808205881616465));
#17280=CARTESIAN_POINT('Ctrl Pts',(93.584305774443,2.10239637081351,0.676113590212933));
#17281=CARTESIAN_POINT('Ctrl Pts',(93.5735931051871,2.15606209240247,0.463939127097435));
#17282=CARTESIAN_POINT('Ctrl Pts',(93.569662693869,2.17128802660668,0.386457545033741));
#17283=CARTESIAN_POINT('Ctrl Pts',(93.5645432732366,2.18499300103845,0.289456487168083));
#17284=CARTESIAN_POINT('Ctrl Pts',(93.5635358915841,2.18741499916114,0.270545829009715));
#17285=CARTESIAN_POINT('Ctrl Pts',(93.5620305713203,2.19062582557879,0.242603824419862));
#17286=CARTESIAN_POINT('Ctrl Pts',(93.5615426502332,2.19160480323373,0.233594742868918));
#17287=CARTESIAN_POINT('Ctrl Pts',(93.5607044760275,2.19318099568821,0.218206704199088));
#17288=CARTESIAN_POINT('Ctrl Pts',(93.5603557754096,2.1938059986527,0.211830792826221));
#17289=CARTESIAN_POINT('Ctrl Pts',(93.559554746513,2.19517163778844,0.197244604355678));
#17290=CARTESIAN_POINT('Ctrl Pts',(93.5591014332354,2.19589400251204,0.189033008989035));
#17291=CARTESIAN_POINT('Ctrl Pts',(93.5578383982255,2.1977682051405,0.16626522721368));
#17292=CARTESIAN_POINT('Ctrl Pts',(93.5570235145801,2.19882145880143,0.151701609389933));
#17293=CARTESIAN_POINT('Ctrl Pts',(93.552132572279,2.20422920517113,0.0649542351037719));
#17294=CARTESIAN_POINT('Ctrl Pts',(93.5479018377236,2.20517322976083,-0.00739231330563989));
#17295=CARTESIAN_POINT('Ctrl Pts',(93.535693768828,2.19774872551549,-0.212708820541933));
#17296=CARTESIAN_POINT('Ctrl Pts',(93.5276005580955,2.18088843175286,-0.345069445179283));
#17297=CARTESIAN_POINT('Ctrl Pts',(93.5159931108789,2.13846789426629,-0.537233741348164));
#17298=CARTESIAN_POINT('Ctrl Pts',(93.5122957336523,2.12206607826796,-0.59875002906928));
#17299=CARTESIAN_POINT('Ctrl Pts',(93.5062086403788,2.09004364066282,-0.700867662469533));
#17300=CARTESIAN_POINT('Ctrl Pts',(93.5037783362893,2.07584349521482,-0.741870647308984));
#17301=CARTESIAN_POINT('Ctrl Pts',(93.5004084762503,2.05413388652524,-0.799040470477603));
#17302=CARTESIAN_POINT('Ctrl Pts',(93.4994360893055,2.04762545585654,-0.815574469852261));
#17303=CARTESIAN_POINT('Ctrl Pts',(93.4977703241192,2.03605470230212,-0.843956863833963));
#17304=CARTESIAN_POINT('Ctrl Pts',(93.497073793507,2.0310871902943,-0.855842727409971));
#17305=CARTESIAN_POINT('Ctrl Pts',(93.4957432895972,2.02135044406547,-0.878577718898446));
#17306=CARTESIAN_POINT('Ctrl Pts',(93.4951087968149,2.01659736757408,-0.889433241179307));
#17307=CARTESIAN_POINT('Ctrl Pts',(93.4934502120683,2.00388510223251,-0.91784089035594));
#17308=CARTESIAN_POINT('Ctrl Pts',(93.4924310556804,1.99578275706997,-0.935328082015062));
#17309=CARTESIAN_POINT('Ctrl Pts',(93.4888037306351,1.96591043233258,-0.997645038404249));
#17310=CARTESIAN_POINT('Ctrl Pts',(93.4862400619051,1.94285013870369,-1.04184128696349));
#17311=CARTESIAN_POINT('Ctrl Pts',(93.4756156453453,1.83944885091134,-1.22462056636108));
#17312=CARTESIAN_POINT('Ctrl Pts',(93.4680215633989,1.74563093271669,-1.35500604578568));
#17313=CARTESIAN_POINT('Ctrl Pts',(93.4558335291167,1.57819061843789,-1.54112432022936));
#17314=CARTESIAN_POINT('Ctrl Pts',(93.4513794049857,1.51381811716872,-1.60440068541811));
#17315=CARTESIAN_POINT('Ctrl Pts',(93.4456197649533,1.43044968978261,-1.67685450544111));
#17316=CARTESIAN_POINT('Ctrl Pts',(93.4445498100754,1.41495894746829,-1.68994629108733));
#17317=CARTESIAN_POINT('Ctrl Pts',(93.4429685609006,1.39211372736261,-1.70871930162054));
#17318=CARTESIAN_POINT('Ctrl Pts',(93.4424687908163,1.38490007930343,-1.7145710967179));
#17319=CARTESIAN_POINT('Ctrl Pts',(93.4415811297548,1.37210578412407,-1.72481655915851));
#17320=CARTESIAN_POINT('Ctrl Pts',(93.4411945882044,1.36654058716386,-1.72922909635091));
#17321=CARTESIAN_POINT('Ctrl Pts',(93.4403483645369,1.35437213683413,-1.73878179600393));
#17322=CARTESIAN_POINT('Ctrl Pts',(93.4398879893912,1.34776100335565,-1.74391120537744));
#17323=CARTESIAN_POINT('Ctrl Pts',(93.4385866098392,1.32909212030213,-1.75822635141928));
#17324=CARTESIAN_POINT('Ctrl Pts',(93.4377399480984,1.31696880891075,-1.76732535133342));
#17325=CARTESIAN_POINT('Ctrl Pts',(93.4313594392685,1.2256856373801,-1.8343760190016));
#17326=CARTESIAN_POINT('Ctrl Pts',(93.4255421403649,1.14283576217411,-1.8871045203934));
#17327=CARTESIAN_POINT('Ctrl Pts',(93.4187993255949,1.04407012779767,-1.94106739643301));
#17328=CARTESIAN_POINT('Ctrl Pts',(93.417931811131,1.03131346971472,-1.94787514827089));
#17329=CARTESIAN_POINT('Ctrl Pts',(93.4118035554381,0.940796389506141,-1.99504226607016));
#17330=CARTESIAN_POINT('Ctrl Pts',(93.4065302328044,0.860754130648719,-2.0308606299483));
#17331=CARTESIAN_POINT('Ctrl Pts',(93.3974401910949,0.716851736606003,-2.08521540943635));
#17332=CARTESIAN_POINT('Ctrl Pts',(93.3935858656735,0.653887000898354,-2.10580925731379));
#17333=CARTESIAN_POINT('Ctrl Pts',(93.3880844748785,0.560802004611938,-2.13167560901881));
#17334=CARTESIAN_POINT('Ctrl Pts',(93.3863717034813,0.5313515489001,-2.13920673355858));
#17335=CARTESIAN_POINT('Ctrl Pts',(93.3832932872548,0.477556646441944,-2.15178371348094));
#17336=CARTESIAN_POINT('Ctrl Pts',(93.3819215387299,0.453265002794533,-2.15703138799492));
#17337=CARTESIAN_POINT('Ctrl Pts',(93.3797784423691,0.414815566812925,-2.16465930452163));
#17338=CARTESIAN_POINT('Ctrl Pts',(93.3789984184152,0.400714900514885,-2.16731387697486));
#17339=CARTESIAN_POINT('Ctrl Pts',(93.3775411243086,0.374175172314,-2.17204234241065));
#17340=CARTESIAN_POINT('Ctrl Pts',(93.3768628847,0.361742341462967,-2.17414753049789));
#17341=CARTESIAN_POINT('Ctrl Pts',(93.3753424389276,0.333692710915717,-2.17864976073448));
#17342=CARTESIAN_POINT('Ctrl Pts',(93.374502193898,0.318066740350762,-2.18098582562306));
#17343=CARTESIAN_POINT('Ctrl Pts',(93.3720319982808,0.271773201860081,-2.18739853947103));
#17344=CARTESIAN_POINT('Ctrl Pts',(93.3704170353733,0.241042795640048,-2.1909978407837));
#17345=CARTESIAN_POINT('Ctrl Pts',(93.3615010376657,0.0690644453104937,
-2.20747849572024));
#17346=CARTESIAN_POINT('Ctrl Pts',(93.3546168788456,-0.0730955019596106,
-2.20734976347764));
#17347=CARTESIAN_POINT('Ctrl Pts',(93.3428687953956,-0.315007155167834,
-2.18371967773079));
#17348=CARTESIAN_POINT('Ctrl Pts',(93.3379961410825,-0.414942724344834,
-2.1669520831745));
#17349=CARTESIAN_POINT('Ctrl Pts',(93.3312896607526,-0.544514657835592,
-2.13591800035786));
#17350=CARTESIAN_POINT('Ctrl Pts',(93.3296556287795,-0.575495998444965,
-2.1277796176765));
#17351=CARTESIAN_POINT('Ctrl Pts',(93.3268317334739,-0.627738776872336,
-2.11283171363186));
#17352=CARTESIAN_POINT('Ctrl Pts',(93.3256576586665,-0.64909466298474,-2.10636888155922));
#17353=CARTESIAN_POINT('Ctrl Pts',(93.323950770794,-0.679538917234773,-2.09664874151746));
#17354=CARTESIAN_POINT('Ctrl Pts',(93.323432213196,-0.688710363921782,-2.09365400985207));
#17355=CARTESIAN_POINT('Ctrl Pts',(93.3225237070262,-0.704636047269229,
-2.08833786697613));
#17356=CARTESIAN_POINT('Ctrl Pts',(93.3221353410121,-0.711399117455989,
-2.08604369573591));
#17357=CARTESIAN_POINT('Ctrl Pts',(93.3212998403101,-0.725850661122635,
-2.08106298377712));
#17358=CARTESIAN_POINT('Ctrl Pts',(93.3208521734447,-0.733535305931576,
-2.07836673262028));
#17359=CARTESIAN_POINT('Ctrl Pts',(93.3196195223198,-0.754541459795169,
-2.07086545587906));
#17360=CARTESIAN_POINT('Ctrl Pts',(93.3188297545146,-0.767831653917365,
-2.06597460796911));
#17361=CARTESIAN_POINT('Ctrl Pts',(93.314435656475,-0.840915228423101,-2.03827695988927));
#17362=CARTESIAN_POINT('Ctrl Pts',(93.3107099447663,-0.899736185700069,
-2.01300393242826));
#17363=CARTESIAN_POINT('Ctrl Pts',(93.2990784541018,-1.07678419263712,-1.92762240560806));
#17364=CARTESIAN_POINT('Ctrl Pts',(93.2910132719407,-1.19076032610242,-1.85937729747585));
#17365=CARTESIAN_POINT('Ctrl Pts',(93.2769668415769,-1.38244641178254,-1.71970842838357));
#17366=CARTESIAN_POINT('Ctrl Pts',(93.2709184566932,-1.46249425211976,-1.65217145255705));
#17367=CARTESIAN_POINT('Ctrl Pts',(93.2637950308372,-1.55426712177235,-1.56282453194235));
#17368=CARTESIAN_POINT('Ctrl Pts',(93.2625013423239,-1.57082098966639,-1.54618507367729));
#17369=CARTESIAN_POINT('Ctrl Pts',(93.2604517607318,-1.59685685049937,-1.51916479257714));
#17370=CARTESIAN_POINT('Ctrl Pts',(93.2596884186271,-1.60651045926708,-1.5089524926651));
#17371=CARTESIAN_POINT('Ctrl Pts',(93.2582453923524,-1.62467398921813,-1.48936586950855));
#17372=CARTESIAN_POINT('Ctrl Pts',(93.2575649442616,-1.63320206381848,-1.48000922041482));
#17373=CARTESIAN_POINT('Ctrl Pts',(93.2560167234031,-1.65251777404208,-1.45844655054329));
#17374=CARTESIAN_POINT('Ctrl Pts',(93.2551512196613,-1.66325172373511,-1.44619329865406));
#17375=CARTESIAN_POINT('Ctrl Pts',(93.2528882395337,-1.69113650233488,-1.41364050494546));
#17376=CARTESIAN_POINT('Ctrl Pts',(93.2515000856677,-1.70805800766838,-1.39314753994207));
#17377=CARTESIAN_POINT('Ctrl Pts',(93.2411677876472,-1.83244648445708,-1.23683132560324));
#17378=CARTESIAN_POINT('Ctrl Pts',(93.2328909531915,-1.92393698612088,-1.08907436591619));
#17379=CARTESIAN_POINT('Ctrl Pts',(93.2188948834625,-2.0461212632412,-0.827278599629718));
#17380=CARTESIAN_POINT('Ctrl Pts',(93.213241039844,-2.08671590481652,-0.718757789847149));
#17381=CARTESIAN_POINT('Ctrl Pts',(93.2063432391737,-2.12284413955009,-0.59277777263816));
#17382=CARTESIAN_POINT('Ctrl Pts',(93.2055258691251,-2.12693042648767,-0.577944342532827));
#17383=CARTESIAN_POINT('Ctrl Pts',(93.2042530940948,-2.13298756204755,-0.555021936602559));
#17384=CARTESIAN_POINT('Ctrl Pts',(93.2038037445118,-2.13506851688171,-0.546962259726661));
#17385=CARTESIAN_POINT('Ctrl Pts',(93.2029657499129,-2.13884179796295,-0.531998396465917));
#17386=CARTESIAN_POINT('Ctrl Pts',(93.2025778074699,-2.14054643651055,-0.525097590067583));
#17387=CARTESIAN_POINT('Ctrl Pts',(93.2016835994286,-2.14437969618979,-0.509250704921521));
#17388=CARTESIAN_POINT('Ctrl Pts',(93.2011760872183,-2.1464857375539,-0.500299444509844));
#17389=CARTESIAN_POINT('Ctrl Pts',(93.1995380337278,-2.1530639224646,-0.471534035110906));
#17390=CARTESIAN_POINT('Ctrl Pts',(93.198396141276,-2.1573180629117,-0.451671690448005));
#17391=CARTESIAN_POINT('Ctrl Pts',(93.1899264316195,-2.18652268988393,-0.305477674139943));
#17392=CARTESIAN_POINT('Ctrl Pts',(93.1821573063825,-2.20063138225343,-0.177242546286337));
#17393=CARTESIAN_POINT('Ctrl Pts',(93.167932121181,-2.20584571300854,0.0595563532546467));
#17394=CARTESIAN_POINT('Ctrl Pts',(93.1614825328575,-2.20027104367885,0.167670236967142));
#17395=CARTESIAN_POINT('Ctrl Pts',(93.1528696039071,-2.18166274314294,0.315671461516062));
#17396=CARTESIAN_POINT('Ctrl Pts',(93.1505296893733,-2.17540539313061,0.356247769589945));
#17397=CARTESIAN_POINT('Ctrl Pts',(93.1464618591503,-2.1623740217958,0.427478953036301));
#17398=CARTESIAN_POINT('Ctrl Pts',(93.1447202327652,-2.15607183920648,0.458207412149979));
#17399=CARTESIAN_POINT('Ctrl Pts',(93.1421391995641,-2.14563863696147,0.504080004448933));
#17400=CARTESIAN_POINT('Ctrl Pts',(93.1412842698145,-2.14199847635309,0.519330681283016));
#17401=CARTESIAN_POINT('Ctrl Pts',(93.1397579948813,-2.13516798153441,0.546653041571861));
#17402=CARTESIAN_POINT('Ctrl Pts',(93.1390847639393,-2.1320372449889,0.558738804945016));
#17403=CARTESIAN_POINT('Ctrl Pts',(93.1376426961688,-2.12507735132605,0.584695907567733));
#17404=CARTESIAN_POINT('Ctrl Pts',(93.1368749799027,-2.12121468308368,0.598557712449143));
#17405=CARTESIAN_POINT('Ctrl Pts',(93.1348171178863,-2.11043685429857,0.635820461420807));
#17406=CARTESIAN_POINT('Ctrl Pts',(93.1335352379196,-2.10326828908577,0.659146373501317));
#17407=CARTESIAN_POINT('Ctrl Pts',(93.1255419100495,-2.05572260372239,0.805174479322779));
#17408=CARTESIAN_POINT('Ctrl Pts',(93.1191858336827,-2.0050102952646,0.924251044399654));
#17409=CARTESIAN_POINT('Ctrl Pts',(93.1083680505205,-1.89989264625379,1.12109443119273));
#17410=CARTESIAN_POINT('Ctrl Pts',(93.1038675718405,-1.85037762538199,1.20106058578348));
#17411=CARTESIAN_POINT('Ctrl Pts',(93.0967253368166,-1.76627647760122,1.31927901568861));
#17412=CARTESIAN_POINT('Ctrl Pts',(93.0941727973656,-1.73520146269131,1.35989155913785));
#17413=CARTESIAN_POINT('Ctrl Pts',(93.0899508911615,-1.68294317982559,1.42347843327447));
#17414=CARTESIAN_POINT('Ctrl Pts',(93.0883256849407,-1.66263377066695,1.44714800522346));
#17415=CARTESIAN_POINT('Ctrl Pts',(93.0860830128931,-1.63450566642378,1.4785559713312));
#17416=CARTESIAN_POINT('Ctrl Pts',(93.0854949148979,-1.62712041512728,1.48667941349272));
#17417=CARTESIAN_POINT('Ctrl Pts',(93.0845044803561,-1.6146758384688,1.5001640812214));
#17418=CARTESIAN_POINT('Ctrl Pts',(93.0841046020389,-1.60964964325076,1.50555583029049));
#17419=CARTESIAN_POINT('Ctrl Pts',(93.083287063713,-1.59937309601679,1.5164695039171));
#17420=CARTESIAN_POINT('Ctrl Pts',(93.0828692816428,-1.59412101086154,1.52198957147081));
#17421=CARTESIAN_POINT('Ctrl Pts',(93.0817803249256,-1.58042658569946,1.53623409562788));
#17422=CARTESIAN_POINT('Ctrl Pts',(93.081105912289,-1.57194070579182,1.54491611198152));
#17423=CARTESIAN_POINT('Ctrl Pts',(93.0783226559348,-1.536879475061,1.58019978883584));
#17424=CARTESIAN_POINT('Ctrl Pts',(93.076172509658,-1.50969848706039,1.606188045857));
#17425=CARTESIAN_POINT('Ctrl Pts',(93.0662158840075,-1.38271826954793,1.72152468665409));
#17426=CARTESIAN_POINT('Ctrl Pts',(93.0580726356368,-1.27556907243249,1.80235371970612));
#17427=CARTESIAN_POINT('Ctrl Pts',(93.0421788952118,-1.04964884311135,1.94248669645377));
#17428=CARTESIAN_POINT('Ctrl Pts',(93.0344589440366,-0.931519404037495,
2.00182368578717));
#17429=CARTESIAN_POINT('Ctrl Pts',(93.0257473730472,-0.786012160526536,
2.05922308164554));
#17430=CARTESIAN_POINT('Ctrl Pts',(93.0243970585048,-0.763099991436265,
2.06782332120856));
#17431=CARTESIAN_POINT('Ctrl Pts',(93.0222796121493,-0.726610012583107,
2.08083094843863));
#17432=CARTESIAN_POINT('Ctrl Pts',(93.0215041486329,-0.713124942137394,
2.08549091983997));
#17433=CARTESIAN_POINT('Ctrl Pts',(93.0200508900681,-0.687627510470923,
2.09402571236726));
#17434=CARTESIAN_POINT('Ctrl Pts',(93.0193721807329,-0.675625319625622,
2.09792891059018));
#17435=CARTESIAN_POINT('Ctrl Pts',(93.0178448045262,-0.648406158697861,
2.10652296177654));
#17436=CARTESIAN_POINT('Ctrl Pts',(93.0169981765061,-0.633170463847152,
2.11115246177686));
#17437=CARTESIAN_POINT('Ctrl Pts',(93.0148189473012,-0.593581853252356,
2.12271468697768));
#17438=CARTESIAN_POINT('Ctrl Pts',(93.0134945532719,-0.569156929815739,
2.12939369696192));
#17439=CARTESIAN_POINT('Ctrl Pts',(93.0026658215889,-0.366637333641922,
2.18103911231749));
#17440=CARTESIAN_POINT('Ctrl Pts',(92.9939307301204,-0.183686324100655,
2.20399999999957));
#17441=CARTESIAN_POINT('Ctrl Pts',(92.9850149380438,-5.17478421224737E-12,
2.204));
#17442=CARTESIAN_POINT('',(93.628116692315,0.00015915216883437,2.20399968871531));
#17443=CARTESIAN_POINT('Ctrl Pts',(92.8757411398941,1.22336862862227E-10,
2.204));
#17444=CARTESIAN_POINT('Ctrl Pts',(92.8857120941664,-0.16597480764464,2.20400000000921));
#17445=CARTESIAN_POINT('Ctrl Pts',(92.8956194489081,-0.331447695365568,
2.18525149933953));
#17446=CARTESIAN_POINT('Ctrl Pts',(92.9064630876008,-0.519824247182944,
2.141994705664));
#17447=CARTESIAN_POINT('Ctrl Pts',(92.9079766238444,-0.546268501020775,
2.13540379919117));
#17448=CARTESIAN_POINT('Ctrl Pts',(92.9103754214465,-0.588412773391464,
2.12406569395616));
#17449=CARTESIAN_POINT('Ctrl Pts',(92.9112706107889,-0.60419324834365,2.11963091203957));
#17450=CARTESIAN_POINT('Ctrl Pts',(92.9128554496667,-0.632220121278324,
2.11141609502695));
#17451=CARTESIAN_POINT('Ctrl Pts',(92.9135472907579,-0.644485659369196,
2.10770454586058));
#17452=CARTESIAN_POINT('Ctrl Pts',(92.9149923108652,-0.670164686830281,
2.09968895652059));
#17453=CARTESIAN_POINT('Ctrl Pts',(92.9157447301723,-0.683570718555069,
2.09536285806611));
#17454=CARTESIAN_POINT('Ctrl Pts',(92.9177257893932,-0.718951746174243,
2.08356977300461));
#17455=CARTESIAN_POINT('Ctrl Pts',(92.9189471745916,-0.740852152386469,
2.07588360817131));
#17456=CARTESIAN_POINT('Ctrl Pts',(92.9252213309961,-0.853705175131841,
2.03426322008874));
#17457=CARTESIAN_POINT('Ctrl Pts',(92.9300830402856,-0.942468709037799,
1.99469166928737));
#17458=CARTESIAN_POINT('Ctrl Pts',(92.9414454245451,-1.14743133916119,1.88657001334687));
#17459=CARTESIAN_POINT('Ctrl Pts',(92.9478207661505,-1.26050877095401,1.81297007782795));
#17460=CARTESIAN_POINT('Ctrl Pts',(92.9578941885746,-1.42052702019115,1.68657020255177));
#17461=CARTESIAN_POINT('Ctrl Pts',(92.9613879837666,-1.47283449179674,1.64108896410067));
#17462=CARTESIAN_POINT('Ctrl Pts',(92.9658068764573,-1.53344195171914,1.5831563720421));
#17463=CARTESIAN_POINT('Ctrl Pts',(92.9665817098654,-1.54387472307975,1.57298414948275));
#17464=CARTESIAN_POINT('Ctrl Pts',(92.9678092227109,-1.56008051337731,1.55686654748618));
#17465=CARTESIAN_POINT('Ctrl Pts',(92.9682566946432,-1.56592234609977,1.55099060484699));
#17466=CARTESIAN_POINT('Ctrl Pts',(92.9690588178212,-1.57627368946636,1.54046072635729));
#17467=CARTESIAN_POINT('Ctrl Pts',(92.9694124590533,-1.58079599423231,1.53581965563095));
#17468=CARTESIAN_POINT('Ctrl Pts',(92.9702735160431,-1.59170787776845,1.52452194753349));
#17469=CARTESIAN_POINT('Ctrl Pts',(92.970782529509,-1.59807615177979,1.51784509865212));
#17470=CARTESIAN_POINT('Ctrl Pts',(92.9723850422269,-1.61787659038382,1.49682248847123));
#17471=CARTESIAN_POINT('Ctrl Pts',(92.9734889876174,-1.63115856856638,1.48233730753433));
#17472=CARTESIAN_POINT('Ctrl Pts',(92.979342532078,-1.69983889654991,1.40539445215957));
#17473=CARTESIAN_POINT('Ctrl Pts',(92.9842791451023,-1.75184513578168,1.34000826903958));
#17474=CARTESIAN_POINT('Ctrl Pts',(92.9977380762131,-1.88170995631609,1.15621233656285));
#17475=CARTESIAN_POINT('Ctrl Pts',(93.0063129910829,-1.95208377297054,1.03297359515815));
#17476=CARTESIAN_POINT('Ctrl Pts',(93.0186552514051,-2.03908990171498,0.839469083831763));
#17477=CARTESIAN_POINT('Ctrl Pts',(93.022675189293,-2.06492338595088,0.773749911333875));
#17478=CARTESIAN_POINT('Ctrl Pts',(93.027804626213,-2.09457535058681,0.686183949310435));
#17479=CARTESIAN_POINT('Ctrl Pts',(93.0290079742925,-2.10128137152249,0.665365281627181));
#17480=CARTESIAN_POINT('Ctrl Pts',(93.0309540023276,-2.11171153231198,0.631253378607787));
#17481=CARTESIAN_POINT('Ctrl Pts',(93.0317027514431,-2.11562251891809,0.618019249956476));
#17482=CARTESIAN_POINT('Ctrl Pts',(93.0331440623767,-2.12295097675411,0.592335869865602));
#17483=CARTESIAN_POINT('Ctrl Pts',(93.033837101633,-2.12638386242474,0.579891638035345));
#17484=CARTESIAN_POINT('Ctrl Pts',(93.0354520312484,-2.1341675652148,0.550676817690431));
#17485=CARTESIAN_POINT('Ctrl Pts',(93.0363710463525,-2.13843039218138,0.533883540504832));
#17486=CARTESIAN_POINT('Ctrl Pts',(93.0393900926016,-2.15187276131681,0.478181606696938));
#17487=CARTESIAN_POINT('Ctrl Pts',(93.0414626949808,-2.16019204570835,0.43907244732139));
#17488=CARTESIAN_POINT('Ctrl Pts',(93.0515179052008,-2.19587260884659,0.245615908689154));
#17489=CARTESIAN_POINT('Ctrl Pts',(93.0590123663761,-2.20777866280608,0.088883934548864));
#17490=CARTESIAN_POINT('Ctrl Pts',(93.0681402053485,-2.2019826996651,-0.0994572953099441));
#17491=CARTESIAN_POINT('Ctrl Pts',(93.0696793206099,-2.2003257201682,-0.131096288299875));
#17492=CARTESIAN_POINT('Ctrl Pts',(93.0753771539066,-2.19173527411179,-0.247156957431132));
#17493=CARTESIAN_POINT('Ctrl Pts',(93.0796024441038,-2.18061968012059,-0.331187458397588));
#17494=CARTESIAN_POINT('Ctrl Pts',(93.0848525857204,-2.16187321222613,-0.429122473933823));
#17495=CARTESIAN_POINT('Ctrl Pts',(93.0856511739632,-2.15889678012207,-0.443854200772686));
#17496=CARTESIAN_POINT('Ctrl Pts',(93.0869082236893,-2.1540246845498,-0.466759069331786));
#17497=CARTESIAN_POINT('Ctrl Pts',(93.0873610619256,-2.15223256758269,-0.474954040688606));
#17498=CARTESIAN_POINT('Ctrl Pts',(93.0882030613034,-2.14883364602683,-0.490082250295158));
#17499=CARTESIAN_POINT('Ctrl Pts',(93.0885914831957,-2.14723999215333,-0.497018170478371));
#17500=CARTESIAN_POINT('Ctrl Pts',(93.0895001550641,-2.14345199701084,-0.513146023942134));
#17501=CARTESIAN_POINT('Ctrl Pts',(93.0900218243079,-2.14123210605389,-0.522331663472147));
#17502=CARTESIAN_POINT('Ctrl Pts',(93.0917053729284,-2.13392121010454,-0.551753279874298));
#17503=CARTESIAN_POINT('Ctrl Pts',(93.0928791976697,-2.128602016111,-0.571930769480351));
#17504=CARTESIAN_POINT('Ctrl Pts',(93.0994784596318,-2.0974268406941,-0.683723981244553));
#17505=CARTESIAN_POINT('Ctrl Pts',(93.1051428419745,-2.06594449814274,-0.773658980374074));
#17506=CARTESIAN_POINT('Ctrl Pts',(93.1213703375746,-1.9602115676304,-1.02271678520752));
#17507=CARTESIAN_POINT('Ctrl Pts',(93.1319268447301,-1.8726323959279,-1.17543409313561));
#17508=CARTESIAN_POINT('Ctrl Pts',(93.1436393170979,-1.74870780052214,-1.34188887163963));
#17509=CARTESIAN_POINT('Ctrl Pts',(93.1454287471041,-1.72899446881725,-1.36719530218094));
#17510=CARTESIAN_POINT('Ctrl Pts',(93.1480850707039,-1.69855258364111,-1.40456221759031));
#17511=CARTESIAN_POINT('Ctrl Pts',(93.1489680547748,-1.68823311180229,-1.41694914594841));
#17512=CARTESIAN_POINT('Ctrl Pts',(93.1504944592617,-1.67004650090356,-1.43829859665395));
#17513=CARTESIAN_POINT('Ctrl Pts',(93.1511403577285,-1.66224091094551,-1.44731245076247));
#17514=CARTESIAN_POINT('Ctrl Pts',(93.1524869770361,-1.64573809871651,-1.46606019035062));
#17515=CARTESIAN_POINT('Ctrl Pts',(93.1531870710633,-1.63702676043598,-1.47578107015957));
#17516=CARTESIAN_POINT('Ctrl Pts',(93.1548535338255,-1.61597832709175,-1.49885305221158));
#17517=CARTESIAN_POINT('Ctrl Pts',(93.1558164635063,-1.60356130664935,-1.5121301491978));
#17518=CARTESIAN_POINT('Ctrl Pts',(93.1591591091192,-1.55958260866614,-1.55800405317259));
#17519=CARTESIAN_POINT('Ctrl Pts',(93.1615023337911,-1.52717894733907,-1.58977966251503));
#17520=CARTESIAN_POINT('Ctrl Pts',(93.1672486566337,-1.44407642941321,-1.66638396371345));
#17521=CARTESIAN_POINT('Ctrl Pts',(93.1706034339528,-1.39225038313005,-1.70992162082279));
#17522=CARTESIAN_POINT('Ctrl Pts',(93.1809051328467,-1.22496669804652,-1.83779618924647));
#17523=CARTESIAN_POINT('Ctrl Pts',(93.1876541138286,-1.10326762233292,-1.9133308267168));
#17524=CARTESIAN_POINT('Ctrl Pts',(93.1976269331511,-0.923886170119412,
-2.00182773612126));
#17525=CARTESIAN_POINT('Ctrl Pts',(93.2005346910079,-0.871691372103053,
-2.02510076458536));
#17526=CARTESIAN_POINT('Ctrl Pts',(93.2042894974147,-0.80565507687788,-2.05151942906736));
#17527=CARTESIAN_POINT('Ctrl Pts',(93.2050351179288,-0.792605402354965,
-2.05659639373236));
#17528=CARTESIAN_POINT('Ctrl Pts',(93.2062221063346,-0.771953443032062,
-2.0644052709607));
#17529=CARTESIAN_POINT('Ctrl Pts',(93.2066587072136,-0.764382784488698,
-2.06722040322442));
#17530=CARTESIAN_POINT('Ctrl Pts',(93.2074923943445,-0.749980234662113,
-2.07248602560038));
#17531=CARTESIAN_POINT('Ctrl Pts',(93.2078890133934,-0.74315150428437,-2.07494446063364));
#17532=CARTESIAN_POINT('Ctrl Pts',(93.2088397696507,-0.726834375344231,
-2.08072796802666));
#17533=CARTESIAN_POINT('Ctrl Pts',(93.209395688463,-0.717335192391652,-2.08402190483849));
#17534=CARTESIAN_POINT('Ctrl Pts',(93.2113128691234,-0.684703331373508,
-2.09508779563051));
#17535=CARTESIAN_POINT('Ctrl Pts',(93.2126909659544,-0.661465054762219,
-2.10254022648159));
#17536=CARTESIAN_POINT('Ctrl Pts',(93.2161473712218,-0.603573711328786,
-2.12005107776756));
#17537=CARTESIAN_POINT('Ctrl Pts',(93.2182445883708,-0.568788814842518,
-2.12964711603335));
#17538=CARTESIAN_POINT('Ctrl Pts',(93.2278740428796,-0.409835201308626,
-2.16932528321663));
#17539=CARTESIAN_POINT('Ctrl Pts',(93.2356412493696,-0.283430906475186,
-2.18943006685147));
#17540=CARTESIAN_POINT('Ctrl Pts',(93.2503756383045,-0.0367672624844075,
-2.20693260825921));
#17541=CARTESIAN_POINT('Ctrl Pts',(93.2573380813423,0.0829660686266078,
-2.20568060950862));
#17542=CARTESIAN_POINT('Ctrl Pts',(93.2653723495126,0.22658194354453,-2.19246093326515));
#17543=CARTESIAN_POINT('Ctrl Pts',(93.266733579356,0.251103262326049,-2.18978801314081));
#17544=CARTESIAN_POINT('Ctrl Pts',(93.2688690035628,0.289860627520369,-2.18490368869045));
#17545=CARTESIAN_POINT('Ctrl Pts',(93.2696516493694,0.304128222890052,-2.18296343307092));
#17546=CARTESIAN_POINT('Ctrl Pts',(93.2710501294238,0.329731242483727,-2.17922577918297));
#17547=CARTESIAN_POINT('Ctrl Pts',(93.2716675502865,0.341073486155282,-2.17747940814325));
#17548=CARTESIAN_POINT('Ctrl Pts',(93.273111674567,0.367689860460666,-2.17316820005079));
#17549=CARTESIAN_POINT('Ctrl Pts',(93.2739360472885,0.382951725101924,-2.1705307765781));
#17550=CARTESIAN_POINT('Ctrl Pts',(93.2763382617193,0.427610377305468,-2.1623275527504));
#17551=CARTESIAN_POINT('Ctrl Pts',(93.2779022030043,0.456923710815786,-2.1563237037659));
#17552=CARTESIAN_POINT('Ctrl Pts',(93.2850363591304,0.591532826864561,-2.1258852055745));
#17553=CARTESIAN_POINT('Ctrl Pts',(93.2903789607237,0.695068772461029,-2.0943212613889));
#17554=CARTESIAN_POINT('Ctrl Pts',(93.3040300853188,0.956866743701798,-1.99294407787394));
#17555=CARTESIAN_POINT('Ctrl Pts',(93.3121370744278,1.1099527124253,-1.91191264640855));
#17556=CARTESIAN_POINT('Ctrl Pts',(93.3221863635486,1.26849471930347,-1.80248135004072));
#17557=CARTESIAN_POINT('Ctrl Pts',(93.3232442162411,1.28483624019738,-1.79086952351595));
#17558=CARTESIAN_POINT('Ctrl Pts',(93.3248084498348,1.30844411100608,-1.77360499609327));
#17559=CARTESIAN_POINT('Ctrl Pts',(93.3253035782826,1.31583747567764,-1.76812680690075));
#17560=CARTESIAN_POINT('Ctrl Pts',(93.3261903484758,1.32893246731872,-1.75829631920462));
#17561=CARTESIAN_POINT('Ctrl Pts',(93.3265807397198,1.33464744900739,-1.75396226698755));
#17562=CARTESIAN_POINT('Ctrl Pts',(93.3274370442597,1.34707301772952,-1.74444323373215));
#17563=CARTESIAN_POINT('Ctrl Pts',(93.3279036828008,1.3537747774502,-1.73924746882646));
#17564=CARTESIAN_POINT('Ctrl Pts',(93.3292519455852,1.37294571020943,-1.72420662413077));
#17565=CARTESIAN_POINT('Ctrl Pts',(93.3301399516686,1.38533838603356,-1.71426542060749));
#17566=CARTESIAN_POINT('Ctrl Pts',(93.3380978143606,1.49445500458864,-1.62477793687495));
#17567=CARTESIAN_POINT('Ctrl Pts',(93.3456211912652,1.58433507152372,-1.53726254067326));
#17568=CARTESIAN_POINT('Ctrl Pts',(93.3628039862581,1.77153319192621,-1.32103731846744));
#17569=CARTESIAN_POINT('Ctrl Pts',(93.3723850219719,1.86317381736594,-1.18830466636839));
#17570=CARTESIAN_POINT('Ctrl Pts',(93.3829660220522,1.95269842699355,-1.02242355272343));
#17571=CARTESIAN_POINT('Ctrl Pts',(93.3845029364724,1.96537617711405,-0.997836483793361));
#17572=CARTESIAN_POINT('Ctrl Pts',(93.386931243176,1.9848755961537,-0.958205273341404));
#17573=CARTESIAN_POINT('Ctrl Pts',(93.3878329528898,1.9919965371105,-0.943312405903441));
#17574=CARTESIAN_POINT('Ctrl Pts',(93.3894252085864,2.00435383217488,-0.916704058621696));
#17575=CARTESIAN_POINT('Ctrl Pts',(93.3901180183246,2.009656394451,-0.90502033215498));
#17576=CARTESIAN_POINT('Ctrl Pts',(93.391560986075,2.0205423164275,-0.880466655891991));
#17577=CARTESIAN_POINT('Ctrl Pts',(93.3923104280041,2.02610544645255,-0.867588333794463));
#17578=CARTESIAN_POINT('Ctrl Pts',(93.3942743854889,2.04043971690847,-0.833515365448055));
#17579=CARTESIAN_POINT('Ctrl Pts',(93.3954818761748,2.04900372810589,-0.812235112041747));
#17580=CARTESIAN_POINT('Ctrl Pts',(93.4015121595105,2.09046864163244,-0.704369159062519));
#17581=CARTESIAN_POINT('Ctrl Pts',(93.4061622953983,2.11822193649965,-0.615900431620633));
#17582=CARTESIAN_POINT('Ctrl Pts',(93.4152255072159,2.16223272988468,-0.436797320582795));
#17583=CARTESIAN_POINT('Ctrl Pts',(93.4196320422737,2.17854750799947,-0.346371716055772));
#17584=CARTESIAN_POINT('Ctrl Pts',(93.4256251541043,2.19287200190162,-0.223488654935204));
#17585=CARTESIAN_POINT('Ctrl Pts',(93.4271760137457,2.19587853708624,-0.191708614386923));
#17586=CARTESIAN_POINT('Ctrl Pts',(93.4328686150059,2.20431113108033,-0.0757650251248282));
#17587=CARTESIAN_POINT('Ctrl Pts',(93.4370766342163,2.2055953601929,0.00861903260830226));
#17588=CARTESIAN_POINT('Ctrl Pts',(93.442307001207,2.20141010894884,0.107866189251395));
#17589=CARTESIAN_POINT('Ctrl Pts',(93.4431050707776,2.20062394606502,0.122864990971442));
#17590=CARTESIAN_POINT('Ctrl Pts',(93.4443614759056,2.19916002346551,0.146224225494058));
#17591=CARTESIAN_POINT('Ctrl Pts',(93.4448141974418,2.1985877120656,0.154591075306799));
#17592=CARTESIAN_POINT('Ctrl Pts',(93.4456561005437,2.19744145379142,0.170052087471947));
#17593=CARTESIAN_POINT('Ctrl Pts',(93.446044544474,2.19688087979474,0.177146974617733));
#17594=CARTESIAN_POINT('Ctrl Pts',(93.4469534285425,2.19549570431192,0.193659448176491));
#17595=CARTESIAN_POINT('Ctrl Pts',(93.447475290178,2.1946448666491,0.203074548105166));
#17596=CARTESIAN_POINT('Ctrl Pts',(93.4491600912566,2.19171998101012,0.233271779701937));
#17597=CARTESIAN_POINT('Ctrl Pts',(93.4503350000238,2.18941115014019,0.254029425706188));
#17598=CARTESIAN_POINT('Ctrl Pts',(93.4569463929965,2.17491710866893,0.369391188702525));
#17599=CARTESIAN_POINT('Ctrl Pts',(93.4626227131336,2.15689606184709,0.463152999278649));
#17600=CARTESIAN_POINT('Ctrl Pts',(93.4788964199204,2.08851564099992,0.725728379517686));
#17601=CARTESIAN_POINT('Ctrl Pts',(93.4894855774807,2.02392820326077,0.890119402739486));
#17602=CARTESIAN_POINT('Ctrl Pts',(93.5013926642765,1.92383579477993,1.07596546090861));
#17603=CARTESIAN_POINT('Ctrl Pts',(93.5033458877859,1.90647163138808,1.1064411219035));
#17604=CARTESIAN_POINT('Ctrl Pts',(93.5061783003804,1.87989367634389,1.15060290872919));
#17605=CARTESIAN_POINT('Ctrl Pts',(93.5070776292229,1.87124242880466,1.16461971534029));
#17606=CARTESIAN_POINT('Ctrl Pts',(93.5086650255563,1.85559564035487,1.18934620640933));
#17607=CARTESIAN_POINT('Ctrl Pts',(93.5093553538396,1.8486625397758,1.20009433081762));
#17608=CARTESIAN_POINT('Ctrl Pts',(93.5108041687347,1.83384164039406,1.22263737497164));
#17609=CARTESIAN_POINT('Ctrl Pts',(93.511561820532,1.82593268975664,1.23441773240945));
#17610=CARTESIAN_POINT('Ctrl Pts',(93.5135729192634,1.80451957298273,1.26565637216092));
#17611=CARTESIAN_POINT('Ctrl Pts',(93.5148187006686,1.79081440203544,1.28497501006123));
#17612=CARTESIAN_POINT('Ctrl Pts',(93.5215782978389,1.71408467482188,1.38951958398089));
#17613=CARTESIAN_POINT('Ctrl Pts',(93.5268610462018,1.64528390915837,1.4703384500147));
#17614=CARTESIAN_POINT('Ctrl Pts',(93.5383109204126,1.48084106912022,1.63744364233642));
#17615=CARTESIAN_POINT('Ctrl Pts',(93.5444037702861,1.38292960214896,1.72093443910016));
#17616=CARTESIAN_POINT('Ctrl Pts',(93.5540332142203,1.22450366422254,1.83373103132184));
#17617=CARTESIAN_POINT('Ctrl Pts',(93.5573723364798,1.16900667281692,1.86959906744733));
#17618=CARTESIAN_POINT('Ctrl Pts',(93.5616114805313,1.0995965095452,1.91015955004592));
#17619=CARTESIAN_POINT('Ctrl Pts',(93.5623749680103,1.08713466303404,1.91727937277578));
#17620=CARTESIAN_POINT('Ctrl Pts',(93.5635883638492,1.06741344226693,1.92829260781846));
#17621=CARTESIAN_POINT('Ctrl Pts',(93.5640332583898,1.06020004895935,1.93226801707187));
#17622=CARTESIAN_POINT('Ctrl Pts',(93.56487271353,1.04662704714868,1.93964941896304));
#17623=CARTESIAN_POINT('Ctrl Pts',(93.5652666847544,1.04027280106005,1.94306472830336));
#17624=CARTESIAN_POINT('Ctrl Pts',(93.5661973592173,1.02529740986403,1.95101925911956));
#17625=CARTESIAN_POINT('Ctrl Pts',(93.5667356392425,1.01666279892074,1.95553258067734));
#17626=CARTESIAN_POINT('Ctrl Pts',(93.5685297296344,0.987960169659007,1.97029400131007));
#17627=CARTESIAN_POINT('Ctrl Pts',(93.5697996930901,0.967765536414832,1.98029127516887));
#17628=CARTESIAN_POINT('Ctrl Pts',(93.5729295068077,0.918188893694589,2.00389456696331));
#17629=CARTESIAN_POINT('Ctrl Pts',(93.5748042468324,0.888653890759159,2.01716592224458));
#17630=CARTESIAN_POINT('Ctrl Pts',(93.5827219774557,0.764092711731034,2.06987010113438));
#17631=CARTESIAN_POINT('Ctrl Pts',(93.5889356350719,0.666659361619681,2.1032745706533));
#17632=CARTESIAN_POINT('Ctrl Pts',(93.6037015921959,0.428849775582664,2.16661446511029));
#17633=CARTESIAN_POINT('Ctrl Pts',(93.6121620417927,0.287164686339577,2.18990365014303));
#17634=CARTESIAN_POINT('Ctrl Pts',(93.6216975236506,0.117309340500798,2.20104088207681));
#17635=CARTESIAN_POINT('Ctrl Pts',(93.6231923520175,0.0903835592114097,
2.20231091106627));
#17636=CARTESIAN_POINT('Ctrl Pts',(93.6253105964606,0.0518079052208622,
2.20342174076335));
#17637=CARTESIAN_POINT('Ctrl Pts',(93.6259464657204,0.0401728052261094,
2.20366457968713));
#17638=CARTESIAN_POINT('Ctrl Pts',(93.6270939537324,0.0190777760891422,
2.20393772929777));
#17639=CARTESIAN_POINT('Ctrl Pts',(93.6276065381154,0.00961859671807106,
2.20399931092351));
#17640=CARTESIAN_POINT('Ctrl Pts',(93.628117219095,0.000159212296038848,
2.20399999424942));
#17641=CARTESIAN_POINT('Ctrl Pts',(93.6281172207996,0.000159180721964109,
2.2039999942517));
#17642=CARTESIAN_POINT('Ctrl Pts',(93.628120085347,0.000106120480998003,
2.2039999980839));
#17643=CARTESIAN_POINT('Ctrl Pts',(93.6281229498343,5.3060240237878E-5,
2.204));
#17644=CARTESIAN_POINT('Ctrl Pts',(93.6281258142613,-2.08913978507926E-13,
2.204));
#17645=CARTESIAN_POINT('Origin',(66.9212607628943,0.,0.));
#17646=CARTESIAN_POINT('',(94.4842111356677,-1.34689240618509E-10,2.204));
#17647=CARTESIAN_POINT('',(94.3756281550323,1.12638885946569E-10,2.204));
#17648=CARTESIAN_POINT('',(66.9212607628943,-2.69912154532077E-16,2.204));
#17649=CARTESIAN_POINT('Ctrl Pts',(94.4842111356677,-1.34689273623145E-10,
2.204));
#17650=CARTESIAN_POINT('Ctrl Pts',(94.4755329260027,0.144554936193152,2.20400000000883));
#17651=CARTESIAN_POINT('Ctrl Pts',(94.4669715239421,0.288779928745478,2.18977863375921));
#17652=CARTESIAN_POINT('Ctrl Pts',(94.4571165643329,0.460855615512199,2.15550003951819));
#17653=CARTESIAN_POINT('Ctrl Pts',(94.4554028323884,0.490991655142827,2.14883588239167));
#17654=CARTESIAN_POINT('Ctrl Pts',(94.4528430644687,0.536314841135943,2.13780997761415));
#17655=CARTESIAN_POINT('Ctrl Pts',(94.451982241008,0.551610507374334,2.13391447242889));
#17656=CARTESIAN_POINT('Ctrl Pts',(94.4504433200519,0.579047215088749,2.12661216165422));
#17657=CARTESIAN_POINT('Ctrl Pts',(94.4497633335038,0.591203255217717,2.12326486421961));
#17658=CARTESIAN_POINT('Ctrl Pts',(94.4483161854108,0.617140001045622,2.11588288471663));
#17659=CARTESIAN_POINT('Ctrl Pts',(94.4475500597095,0.63091139614224,2.11181746045393));
#17660=CARTESIAN_POINT('Ctrl Pts',(94.4454671786757,0.668452680218493,2.10033496996597));
#17661=CARTESIAN_POINT('Ctrl Pts',(94.4441592322409,0.692138527511339,2.09264910981138));
#17662=CARTESIAN_POINT('Ctrl Pts',(94.4412780147371,0.74451002619487,2.07466848902778));
#17663=CARTESIAN_POINT('Ctrl Pts',(94.4397111962772,0.773122826556533,2.06417676647542));
#17664=CARTESIAN_POINT('Ctrl Pts',(94.4347790450191,0.86342836540625,2.02892229545274));
#17665=CARTESIAN_POINT('Ctrl Pts',(94.4314792240034,0.924224275939539,2.00196016740092));
#17666=CARTESIAN_POINT('Ctrl Pts',(94.4218340523172,1.10048438414319,1.91404760938981));
#17667=CARTESIAN_POINT('Ctrl Pts',(94.4156477294851,1.21184926726234,1.8455523486277));
#17668=CARTESIAN_POINT('Ctrl Pts',(94.4057300303503,1.37297071605369,1.72555083613591));
#17669=CARTESIAN_POINT('Ctrl Pts',(94.4021815416241,1.42739088819563,1.68081165490115));
#17670=CARTESIAN_POINT('Ctrl Pts',(94.3977051666337,1.49033571375073,1.62379997956445));
#17671=CARTESIAN_POINT('Ctrl Pts',(94.396932858669,1.50100277890876,1.61394471674125));
#17672=CARTESIAN_POINT('Ctrl Pts',(94.3957111442336,1.51755768450098,1.59834362243017));
#17673=CARTESIAN_POINT('Ctrl Pts',(94.3952669307489,1.52351225618735,1.59266884879891));
#17674=CARTESIAN_POINT('Ctrl Pts',(94.3944719643773,1.53404996823727,1.58251312091587));
#17675=CARTESIAN_POINT('Ctrl Pts',(94.3941222185961,1.53864551403849,1.57804532941381));
#17676=CARTESIAN_POINT('Ctrl Pts',(94.3932727922954,1.54970983096841,1.5671943176669));
#17677=CARTESIAN_POINT('Ctrl Pts',(94.3927715743218,1.55615863396331,1.56079111013264));
#17678=CARTESIAN_POINT('Ctrl Pts',(94.3912023629604,1.57610854780816,1.54073570346931));
#17679=CARTESIAN_POINT('Ctrl Pts',(94.390124422563,1.58947063855862,1.52694718326401));
#17680=CARTESIAN_POINT('Ctrl Pts',(94.3844920145473,1.65764656257154,1.45473095159012));
#17681=CARTESIAN_POINT('Ctrl Pts',(94.3797641813018,1.70942119610173,1.39352478497471));
#17682=CARTESIAN_POINT('Ctrl Pts',(94.3665400319105,1.84297096431901,1.21697623227737));
#17683=CARTESIAN_POINT('Ctrl Pts',(94.3579739670952,1.91717512910132,1.09636596904523));
#17684=CARTESIAN_POINT('Ctrl Pts',(94.3454116421316,2.01193566200479,0.902899355661724));
#17685=CARTESIAN_POINT('Ctrl Pts',(94.3411803758647,2.04116884521913,0.834711854907595));
#17686=CARTESIAN_POINT('Ctrl Pts',(94.3358287098301,2.07463527678722,0.744311355294609));
#17687=CARTESIAN_POINT('Ctrl Pts',(94.3346040500425,2.08204272016849,0.723331934852169));
#17688=CARTESIAN_POINT('Ctrl Pts',(94.3326373353251,2.09352514243281,0.68917242601368));
#17689=CARTESIAN_POINT('Ctrl Pts',(94.331888854483,2.09779613561352,0.676060308202038));
#17690=CARTESIAN_POINT('Ctrl Pts',(94.3304571493909,2.10577302615682,0.650767270620612));
#17691=CARTESIAN_POINT('Ctrl Pts',(94.32977335555,2.10949697712415,0.638592664478323));
#17692=CARTESIAN_POINT('Ctrl Pts',(94.3281935396298,2.11789860509736,0.610249757478722));
#17693=CARTESIAN_POINT('Ctrl Pts',(94.3273001295572,2.12249701669685,0.594058669898781));
#17694=CARTESIAN_POINT('Ctrl Pts',(94.324426998515,2.13678082956936,0.541480740360065));
#17695=CARTESIAN_POINT('Ctrl Pts',(94.3224712676927,2.14571966857923,0.504897046662249));
#17696=CARTESIAN_POINT('Ctrl Pts',(94.3141972667103,2.18001368033813,0.347111368708467));
#17697=CARTESIAN_POINT('Ctrl Pts',(94.30816679732,2.19606968884809,0.224114518980948));
#17698=CARTESIAN_POINT('Ctrl Pts',(94.2951091691506,2.20837133692535,-0.0456128568451124));
#17699=CARTESIAN_POINT('Ctrl Pts',(94.2881297916571,2.20048622062959,-0.191923968391015));
#17700=CARTESIAN_POINT('Ctrl Pts',(94.2795866877272,2.17552760641784,-0.353550998567542));
#17701=CARTESIAN_POINT('Ctrl Pts',(94.278668668687,2.17266911864438,-0.370712205575144));
#17702=CARTESIAN_POINT('Ctrl Pts',(94.2772678624662,2.16805128817065,-0.396544900281867));
#17703=CARTESIAN_POINT('Ctrl Pts',(94.27679295198,2.16644233509168,-0.405242951132153));
#17704=CARTESIAN_POINT('Ctrl Pts',(94.2759257322284,2.16342728137486,-0.421011116281111));
#17705=CARTESIAN_POINT('Ctrl Pts',(94.2755344010851,2.16203875327917,-0.42808455960588));
#17706=CARTESIAN_POINT('Ctrl Pts',(94.2747185829523,2.15908705485425,-0.442740356607223));
#17707=CARTESIAN_POINT('Ctrl Pts',(94.2742938197746,2.15751860642754,-0.450321432894227));
#17708=CARTESIAN_POINT('Ctrl Pts',(94.2731666355447,2.15327235524986,-0.470314132517021));
#17709=CARTESIAN_POINT('Ctrl Pts',(94.2724605589959,2.15052721935581,-0.482710971779726));
#17710=CARTESIAN_POINT('Ctrl Pts',(94.2690893050089,2.13701072239248,-0.54134566475598));
#17711=CARTESIAN_POINT('Ctrl Pts',(94.2663567207286,2.1248549478544,-0.587248480012665));
#17712=CARTESIAN_POINT('Ctrl Pts',(94.2576956166837,2.08235623116248,-0.729056106455512));
#17713=CARTESIAN_POINT('Ctrl Pts',(94.251626214002,2.0469259610892,-0.823300103081853));
#17714=CARTESIAN_POINT('Ctrl Pts',(94.2370259418136,1.94596461217234,-1.04460323400846));
#17715=CARTESIAN_POINT('Ctrl Pts',(94.2285813858493,1.87426989969075,-1.1683738141596));
#17716=CARTESIAN_POINT('Ctrl Pts',(94.2188278364962,1.77308359070473,-1.30948332158075));
#17717=CARTESIAN_POINT('Ctrl Pts',(94.2171107187019,1.7545385013355,-1.33422890593055));
#17718=CARTESIAN_POINT('Ctrl Pts',(94.2145469469628,1.72574166342128,-1.37101466296442));
#17719=CARTESIAN_POINT('Ctrl Pts',(94.213685436762,1.71587155267967,-1.3833475080242));
#17720=CARTESIAN_POINT('Ctrl Pts',(94.212145768402,1.6978854444494,-1.4053327032635));
#17721=CARTESIAN_POINT('Ctrl Pts',(94.2114657135551,1.68981764606795,-1.41502343499562));
#17722=CARTESIAN_POINT('Ctrl Pts',(94.2100189252977,1.67239121909451,-1.43559379237224));
#17723=CARTESIAN_POINT('Ctrl Pts',(94.2092532221364,1.66300857003547,-1.44645236205736));
#17724=CARTESIAN_POINT('Ctrl Pts',(94.2071727768072,1.63708331464815,-1.47587000419676));
#17725=CARTESIAN_POINT('Ctrl Pts',(94.2058668079152,1.62033143840077,-1.49424233112496));
#17726=CARTESIAN_POINT('Ctrl Pts',(94.1965103074908,1.4969528290348,-1.6250403293642));
#17727=CARTESIAN_POINT('Ctrl Pts',(94.1889918462647,1.37904397359871,-1.7262293223493));
#17728=CARTESIAN_POINT('Ctrl Pts',(94.1750114835914,1.14093667234046,-1.89048031328777));
#17729=CARTESIAN_POINT('Ctrl Pts',(94.1685564835556,1.02366148421603,-1.95646657076188));
#17730=CARTESIAN_POINT('Ctrl Pts',(94.1605019136442,0.882728565424131,-2.01960707890652));
#17731=CARTESIAN_POINT('Ctrl Pts',(94.1594381506976,0.864217924280999,-2.02759704972671));
#17732=CARTESIAN_POINT('Ctrl Pts',(94.1578696584096,0.837134162115,-2.03884929666943));
#17733=CARTESIAN_POINT('Ctrl Pts',(94.1573763634874,0.828645671476639,-2.04231398296313));
#17734=CARTESIAN_POINT('Ctrl Pts',(94.1564951204699,0.813540513966217,-2.04836967452848));
#17735=CARTESIAN_POINT('Ctrl Pts',(94.1561084362098,0.806932592824048,-2.0509817845527));
#17736=CARTESIAN_POINT('Ctrl Pts',(94.1552634469718,0.792538271984392,-2.05659152388252));
#17737=CARTESIAN_POINT('Ctrl Pts',(94.1548044663219,0.784747560890426,-2.05957686665034));
#17738=CARTESIAN_POINT('Ctrl Pts',(94.1534869599285,0.762457040568895,-2.06797359482819));
#17739=CARTESIAN_POINT('Ctrl Pts',(94.1526224124811,0.747917208585949,-2.07327647676347));
#17740=CARTESIAN_POINT('Ctrl Pts',(94.1451748638944,0.623278475895987,-2.11725229583426));
#17741=CARTESIAN_POINT('Ctrl Pts',(94.1381936957908,0.51033363417477,-2.14727454984663));
#17742=CARTESIAN_POINT('Ctrl Pts',(94.1208700013375,0.226583140071448,-2.19904026816622));
#17743=CARTESIAN_POINT('Ctrl Pts',(94.1105980807696,0.0545569434765714,
-2.2100135847477));
#17744=CARTESIAN_POINT('Ctrl Pts',(94.0994680885465,-0.143690417938653,
-2.19947325445585));
#17745=CARTESIAN_POINT('Ctrl Pts',(94.0979852556208,-0.170337573629096,
-2.19757018833114));
#17746=CARTESIAN_POINT('Ctrl Pts',(94.0956298748282,-0.213034159776627,
-2.19373959500773));
#17747=CARTESIAN_POINT('Ctrl Pts',(94.0947478421117,-0.229107847546192,
-2.19211919788558));
#17748=CARTESIAN_POINT('Ctrl Pts',(94.0931836076428,-0.257760232961659,
-2.18891213882756));
#17749=CARTESIAN_POINT('Ctrl Pts',(94.0924993021811,-0.270345668103714,
-2.18739340730363));
#17750=CARTESIAN_POINT('Ctrl Pts',(94.0910674996146,-0.296781812468318,
-2.18397161055297));
#17751=CARTESIAN_POINT('Ctrl Pts',(94.0903207727717,-0.310628960843505,
-2.18204516473301));
#17752=CARTESIAN_POINT('Ctrl Pts',(94.0883493310487,-0.347337580166986,
-2.17658165942564));
#17753=CARTESIAN_POINT('Ctrl Pts',(94.0871318588954,-0.370163602299328,
-2.17281616245498));
#17754=CARTESIAN_POINT('Ctrl Pts',(94.0807996096661,-0.489606745909725,
-2.1511752827106));
#17755=CARTESIAN_POINT('Ctrl Pts',(94.0758811870315,-0.585012139986624,
-2.12721261051288));
#17756=CARTESIAN_POINT('Ctrl Pts',(94.0667462217839,-0.762351478572828,
-2.0698313738539));
#17757=CARTESIAN_POINT('Ctrl Pts',(94.0625163776412,-0.844493294563531,
-2.0376979614208));
#17758=CARTESIAN_POINT('Ctrl Pts',(94.0570318346265,-0.947217573138083,
-1.99023156558713));
#17759=CARTESIAN_POINT('Ctrl Pts',(94.0558152035112,-0.969764045397713,
-1.97934344848997));
#17760=CARTESIAN_POINT('Ctrl Pts',(94.0502530192008,-1.07140222953487,-1.92810692029083));
#17761=CARTESIAN_POINT('Ctrl Pts',(94.045835841344,-1.1481896513284,-1.88338961717163));
#17762=CARTESIAN_POINT('Ctrl Pts',(94.0403703586209,-1.23457791592129,-1.82583118452948));
#17763=CARTESIAN_POINT('Ctrl Pts',(94.0395713373945,-1.2470066320971,-1.81736528516943));
#17764=CARTESIAN_POINT('Ctrl Pts',(94.0383164186815,-1.26619272147761,-1.80400708573333));
#17765=CARTESIAN_POINT('Ctrl Pts',(94.0378661815826,-1.27301081731342,-1.79920233094015));
#17766=CARTESIAN_POINT('Ctrl Pts',(94.0370274410703,-1.28558669705435,-1.79023276165223));
#17767=CARTESIAN_POINT('Ctrl Pts',(94.0366396523033,-1.2913518005242,-1.78607867107639));
#17768=CARTESIAN_POINT('Ctrl Pts',(94.0357383987963,-1.30463786954054,-1.77640733861523));
#17769=CARTESIAN_POINT('Ctrl Pts',(94.035223595197,-1.31214397914477,-1.7708701744779));
#17770=CARTESIAN_POINT('Ctrl Pts',(94.0335679341264,-1.33602965786903,-1.75301476959742));
#17771=CARTESIAN_POINT('Ctrl Pts',(94.0324155622602,-1.35227219561552,-1.74051597998687));
#17772=CARTESIAN_POINT('Ctrl Pts',(94.0260068648147,-1.44067935144202,-1.67050132838555));
#17773=CARTESIAN_POINT('Ctrl Pts',(94.0205245701103,-1.50934601792695,-1.60872728705917));
#17774=CARTESIAN_POINT('Ctrl Pts',(94.0050296166324,-1.6903091583838,-1.4241169313775));
#17775=CARTESIAN_POINT('Ctrl Pts',(93.995001060159,-1.79289649630129,-1.29259063495724));
#17776=CARTESIAN_POINT('Ctrl Pts',(93.9830493245384,-1.90250050849489,-1.11355792286878));
#17777=CARTESIAN_POINT('Ctrl Pts',(93.9806026812108,-1.92417120065752,-1.07567885658972));
#17778=CARTESIAN_POINT('Ctrl Pts',(93.9771877153821,-1.9533065421853,-1.02105029295934));
#17779=CARTESIAN_POINT('Ctrl Pts',(93.9761865451057,-1.96170797451672,-1.00481441055363));
#17780=CARTESIAN_POINT('Ctrl Pts',(93.9744939846191,-1.97566747718466,-0.976994888475123));
#17781=CARTESIAN_POINT('Ctrl Pts',(93.9737990304719,-1.98132793429741,-0.965463939806464));
#17782=CARTESIAN_POINT('Ctrl Pts',(93.9723929637161,-1.99263299206583,-0.941916132673545));
#17783=CARTESIAN_POINT('Ctrl Pts',(93.9716821193975,-1.99827047187394,-0.929896431822365));
#17784=CARTESIAN_POINT('Ctrl Pts',(93.9699196131322,-2.01205017881955,-0.899812566318307));
#17785=CARTESIAN_POINT('Ctrl Pts',(93.968872583281,-2.02005814990925,-0.881687972976864));
#17786=CARTESIAN_POINT('Ctrl Pts',(93.9647637098073,-2.05075498347698,-0.809596780055301));
#17787=CARTESIAN_POINT('Ctrl Pts',(93.9617659996779,-2.07153525340022,-0.754841302692485));
#17788=CARTESIAN_POINT('Ctrl Pts',(93.9537973566608,-2.12183968627772,-0.604492560710857));
#17789=CARTESIAN_POINT('Ctrl Pts',(93.9489459130672,-2.14707856300133,-0.507612151778338));
#17790=CARTESIAN_POINT('Ctrl Pts',(93.9372734857204,-2.19192285542642,-0.270364889169396));
#17791=CARTESIAN_POINT('Ctrl Pts',(93.9305019197053,-2.20475028511078,-0.129189505346149));
#17792=CARTESIAN_POINT('Ctrl Pts',(93.9220958357517,-2.20385744177126,0.0318187137023454));
#17793=CARTESIAN_POINT('Ctrl Pts',(93.9210610612339,-2.20348740256429,0.0514127281607357));
#17794=CARTESIAN_POINT('Ctrl Pts',(93.9195224612757,-2.20256099543877,0.0801561656346075));
#17795=CARTESIAN_POINT('Ctrl Pts',(93.9190293005446,-2.20220874609843,0.0893117129892938));
#17796=CARTESIAN_POINT('Ctrl Pts',(93.9181487575143,-2.20148256736756,0.10555003003969));
#17797=CARTESIAN_POINT('Ctrl Pts',(93.9177626423583,-2.2011315235986,0.112633552907477));
#17798=CARTESIAN_POINT('Ctrl Pts',(93.9169116901552,-2.20028677740135,0.128162645728139));
#17799=CARTESIAN_POINT('Ctrl Pts',(93.9164460956575,-2.19977864548602,0.13660700033643));
#17800=CARTESIAN_POINT('Ctrl Pts',(93.9150906546537,-2.19816670936478,0.161047209297219));
#17801=CARTESIAN_POINT('Ctrl Pts',(93.9141942543842,-2.1969369720768,0.177033883603621));
#17802=CARTESIAN_POINT('Ctrl Pts',(93.9065278162353,-2.18503506853992,0.312424107077827));
#17803=CARTESIAN_POINT('Ctrl Pts',(93.8993424422437,-2.16481246936675,0.430777211013497));
#17804=CARTESIAN_POINT('Ctrl Pts',(93.8821181903364,-2.09366793878611,0.708528611365436));
#17805=CARTESIAN_POINT('Ctrl Pts',(93.8721557373993,-2.03403508891293,0.864971937865329));
#17806=CARTESIAN_POINT('Ctrl Pts',(93.8612708318752,-1.94482962318424,1.03729944259209));
#17807=CARTESIAN_POINT('Ctrl Pts',(93.8597637957971,-1.93191026705024,1.06116690934273));
#17808=CARTESIAN_POINT('Ctrl Pts',(93.8573778216672,-1.91054254792675,1.09895771096546));
#17809=CARTESIAN_POINT('Ctrl Pts',(93.85648900359,-1.90237527029695,1.11303604117105));
#17810=CARTESIAN_POINT('Ctrl Pts',(93.8549170723783,-1.88756231723248,1.13793040065963));
#17811=CARTESIAN_POINT('Ctrl Pts',(93.8542317812317,-1.88097779958548,1.14878180045678));
#17812=CARTESIAN_POINT('Ctrl Pts',(93.8528022295888,-1.86697741924999,1.17141154876758));
#17813=CARTESIAN_POINT('Ctrl Pts',(93.8520586935166,-1.85954297108029,1.18317777677668));
#17814=CARTESIAN_POINT('Ctrl Pts',(93.8501055568538,-1.83961363650393,1.21406731677005));
#17815=CARTESIAN_POINT('Ctrl Pts',(93.8489029538784,-1.8269318850441,1.23306841671087));
#17816=CARTESIAN_POINT('Ctrl Pts',(93.8428381209405,-1.76092389569107,1.32871388365581));
#17817=CARTESIAN_POINT('Ctrl Pts',(93.8381517794172,-1.70305908108346,1.40211477030022));
#17818=CARTESIAN_POINT('Ctrl Pts',(93.829079686912,-1.57975744356482,1.53958271077273));
#17819=CARTESIAN_POINT('Ctrl Pts',(93.8246976335095,-1.51464367833092,1.60368430573631));
#17820=CARTESIAN_POINT('Ctrl Pts',(93.8186737245841,-1.42078638182128,1.68525229344282));
#17821=CARTESIAN_POINT('Ctrl Pts',(93.8170669901237,-1.39534526113366,1.70637650515202));
#17822=CARTESIAN_POINT('Ctrl Pts',(93.8113662518331,-1.30418404530579,1.77866689177433));
#17823=CARTESIAN_POINT('Ctrl Pts',(93.8072070502701,-1.23605445340312,1.826668739746));
#17824=CARTESIAN_POINT('Ctrl Pts',(93.8020371332055,-1.15273581872842,1.87857341028165));
#17825=CARTESIAN_POINT('Ctrl Pts',(93.8012454167395,-1.14001230350998,1.88632177781117));
#17826=CARTESIAN_POINT('Ctrl Pts',(93.7999995738072,-1.12007095322274,1.89819021951072));
#17827=CARTESIAN_POINT('Ctrl Pts',(93.7995509781694,-1.11290647974577,1.90239959326288));
#17828=CARTESIAN_POINT('Ctrl Pts',(93.7987172854616,-1.09962598297259,1.91010164675259));
#17829=CARTESIAN_POINT('Ctrl Pts',(93.798332917789,-1.09351682331345,1.91360564275796));
#17830=CARTESIAN_POINT('Ctrl Pts',(93.7974347477554,-1.07927193067843,1.92168551721675));
#17831=CARTESIAN_POINT('Ctrl Pts',(93.7969195672158,-1.07112383915196,1.92623904076157));
#17832=CARTESIAN_POINT('Ctrl Pts',(93.7952614640521,-1.04496148098274,1.94064242885874));
#17833=CARTESIAN_POINT('Ctrl Pts',(93.7941069810965,-1.02683890501674,1.95029211523496));
#17834=CARTESIAN_POINT('Ctrl Pts',(93.7876751291781,-0.926209605777247,
2.00208262787474));
#17835=CARTESIAN_POINT('Ctrl Pts',(93.782170127685,-0.841249558976145,2.03923893800935));
#17836=CARTESIAN_POINT('Ctrl Pts',(93.7702655775841,-0.654643359567615,
2.10719883952728));
#17837=CARTESIAN_POINT('Ctrl Pts',(93.7638698039526,-0.55258383915252,2.13623451614533));
#17838=CARTESIAN_POINT('Ctrl Pts',(93.754913509879,-0.403762671966871,2.16718955117525));
#17839=CARTESIAN_POINT('Ctrl Pts',(93.7522306450708,-0.358411929414702,
2.17514967342432));
#17840=CARTESIAN_POINT('Ctrl Pts',(93.7464887600969,-0.259476925040162,
2.18933648342462));
#17841=CARTESIAN_POINT('Ctrl Pts',(93.7434460627509,-0.205845036979493,
2.19502871044619));
#17842=CARTESIAN_POINT('Ctrl Pts',(93.7393913588451,-0.132702182608141,
2.20008691841751));
#17843=CARTESIAN_POINT('Ctrl Pts',(93.7383265074971,-0.113332247361482,
2.20116972393609));
#17844=CARTESIAN_POINT('Ctrl Pts',(93.7365429726326,-0.080623317050864,
2.20256527870119));
#17845=CARTESIAN_POINT('Ctrl Pts',(93.7358201104746,-0.0672914576818401,
2.2030128907681));
#17846=CARTESIAN_POINT('Ctrl Pts',(93.7346098872167,-0.0448480070696404,
2.20356249382968));
#17847=CARTESIAN_POINT('Ctrl Pts',(93.7341205212728,-0.035738479639022,
2.20372906058751));
#17848=CARTESIAN_POINT('Ctrl Pts',(93.7331578692262,-0.0177525462416429,
2.20394637724993));
#17849=CARTESIAN_POINT('Ctrl Pts',(93.7326845030318,-0.00887635722052226,
2.204));
#17850=CARTESIAN_POINT('Ctrl Pts',(93.7322127872898,-1.52555169845894E-15,
2.204));
#17851=CARTESIAN_POINT('Ctrl Pts',(93.6281258142613,-2.08913978507926E-13,
2.204));
#17852=CARTESIAN_POINT('Ctrl Pts',(93.6287336333723,-0.0112591551814979,
2.204));
#17853=CARTESIAN_POINT('Ctrl Pts',(93.6293387394407,-0.022518296427486,
2.2039137237877));
#17854=CARTESIAN_POINT('Ctrl Pts',(93.6307286024886,-0.0484919604802062,
2.20351562898419));
#17855=CARTESIAN_POINT('Ctrl Pts',(93.6315114239032,-0.0632050857157136,
2.20314269369862));
#17856=CARTESIAN_POINT('Ctrl Pts',(93.6338368903869,-0.10715072333209,2.20158819953408));
#17857=CARTESIAN_POINT('Ctrl Pts',(93.6353659969666,-0.136365169972084,
2.19997193701538));
#17858=CARTESIAN_POINT('Ctrl Pts',(93.6473048774245,-0.366641036528467,
2.18262720805577));
#17859=CARTESIAN_POINT('Ctrl Pts',(93.6567740931849,-0.564697751164643,
2.13995414131552));
#17860=CARTESIAN_POINT('Ctrl Pts',(93.6695478127351,-0.810120517242369,
2.0505763457388));
#17861=CARTESIAN_POINT('Ctrl Pts',(93.6724963725378,-0.865196118094291,
2.02795303212838));
#17862=CARTESIAN_POINT('Ctrl Pts',(93.677303019617,-0.950744061277059,1.98869299048612));
#17863=CARTESIAN_POINT('Ctrl Pts',(93.6791006146663,-0.981856627121886,
1.97351751654895));
#17864=CARTESIAN_POINT('Ctrl Pts',(93.6815487943064,-1.02278999316325,1.952344313673));
#17865=CARTESIAN_POINT('Ctrl Pts',(93.6821628776929,-1.03294118527824,1.94699260027798));
#17866=CARTESIAN_POINT('Ctrl Pts',(93.6831877388142,-1.0496792338797,1.93800055154315));
#17867=CARTESIAN_POINT('Ctrl Pts',(93.6835957364622,-1.05629019837473,1.93440524340744));
#17868=CARTESIAN_POINT('Ctrl Pts',(93.6843710598922,-1.06875051628291,1.92754590138267));
#17869=CARTESIAN_POINT('Ctrl Pts',(93.6847379200292,-1.0746036592805,1.92428891826811));
#17870=CARTESIAN_POINT('Ctrl Pts',(93.6856151887193,-1.08850174694825,1.91647213909086));
#17871=CARTESIAN_POINT('Ctrl Pts',(93.6861270850565,-1.09653295611892,1.91188832910391));
#17872=CARTESIAN_POINT('Ctrl Pts',(93.6876918582071,-1.12085471828714,1.89780303517945));
#17873=CARTESIAN_POINT('Ctrl Pts',(93.6887539027612,-1.13705198914173,1.88814310538913));
#17874=CARTESIAN_POINT('Ctrl Pts',(93.6960922217737,-1.24703069730724,1.82062433108904));
#17875=CARTESIAN_POINT('Ctrl Pts',(93.702691806428,-1.33647556786597,1.7560147363038));
#17876=CARTESIAN_POINT('Ctrl Pts',(93.7153286775383,-1.49731043394918,1.62040651052834));
#17877=CARTESIAN_POINT('Ctrl Pts',(93.7213483601906,-1.56942478570504,1.55066560497573));
#17878=CARTESIAN_POINT('Ctrl Pts',(93.7320565384587,-1.69188073640857,1.41491358622701));
#17879=CARTESIAN_POINT('Ctrl Pts',(93.7367863396081,-1.74372700621387,1.35050340671083));
#17880=CARTESIAN_POINT('Ctrl Pts',(93.7426078167322,-1.80478696895649,1.2652487889178));
#17881=CARTESIAN_POINT('Ctrl Pts',(93.743831881397,-1.81746114043506,1.24697456084284));
#17882=CARTESIAN_POINT('Ctrl Pts',(93.7458027848477,-1.83759247484038,1.21698910962731));
#17883=CARTESIAN_POINT('Ctrl Pts',(93.7465559882761,-1.84521915616819,1.20539407441314));
#17884=CARTESIAN_POINT('Ctrl Pts',(93.7480002429084,-1.8597111975657,1.1829015675901));
#17885=CARTESIAN_POINT('Ctrl Pts',(93.7486918343562,-1.86659153540862,1.17201446520428));
#17886=CARTESIAN_POINT('Ctrl Pts',(93.7502793192397,-1.88224415579107,1.14675904695954));
#17887=CARTESIAN_POINT('Ctrl Pts',(93.7511726787168,-1.89094809673794,1.13234919103025));
#17888=CARTESIAN_POINT('Ctrl Pts',(93.7540717944158,-1.91883818234023,1.08495707885936));
#17889=CARTESIAN_POINT('Ctrl Pts',(93.7560527648294,-1.93733360653031,1.05157527375701));
#17890=CARTESIAN_POINT('Ctrl Pts',(93.7668476497605,-2.03466870231767,0.86460441527319));
#17891=CARTESIAN_POINT('Ctrl Pts',(93.775041516706,-2.09611601894787,0.702650431957959));
#17892=CARTESIAN_POINT('Ctrl Pts',(93.7880163133032,-2.16093663996481,0.443692506170338));
#17893=CARTESIAN_POINT('Ctrl Pts',(93.7926595442009,-2.17793923385807,0.350838455563421));
#17894=CARTESIAN_POINT('Ctrl Pts',(93.7986546785752,-2.19136715680751,0.23655390584678));
#17895=CARTESIAN_POINT('Ctrl Pts',(93.7997501360028,-2.19349986331265,0.215884353894427));
#17896=CARTESIAN_POINT('Ctrl Pts',(93.8013651879752,-2.19617545469124,0.185791224037283));
#17897=CARTESIAN_POINT('Ctrl Pts',(93.8018726531813,-2.19695060694801,0.176388862380202));
#17898=CARTESIAN_POINT('Ctrl Pts',(93.8027722207416,-2.1982093075537,0.15982298759138));
#17899=CARTESIAN_POINT('Ctrl Pts',(93.8031629131929,-2.19871825359597,0.152661674927733));
#17900=CARTESIAN_POINT('Ctrl Pts',(93.8040165168038,-2.19974849023385,0.137089698353008));
#17901=CARTESIAN_POINT('Ctrl Pts',(93.8044801150386,-2.2002565339156,0.128678614389766));
#17902=CARTESIAN_POINT('Ctrl Pts',(93.8057870222722,-2.20154567271148,0.105088795833398));
#17903=CARTESIAN_POINT('Ctrl Pts',(93.8066359965997,-2.20221799361621,0.0899048745588194));
#17904=CARTESIAN_POINT('Ctrl Pts',(93.8126810266257,-2.20585549267657,-0.0173342323559837));
#17905=CARTESIAN_POINT('Ctrl Pts',(93.8181267267075,-2.20320440024947,-0.109481239464676));
#17906=CARTESIAN_POINT('Ctrl Pts',(93.8249102580592,-2.19285525527252,-0.222385162907419));
#17907=CARTESIAN_POINT('Ctrl Pts',(93.8261874391232,-2.19060462044845,-0.243558446293098));
#17908=CARTESIAN_POINT('Ctrl Pts',(93.8327451920336,-2.17748831968346,-0.351981421917578));
#17909=CARTESIAN_POINT('Ctrl Pts',(93.8380362644771,-2.16171506968749,-0.438560582336383));
#17910=CARTESIAN_POINT('Ctrl Pts',(93.8490398235673,-2.1174243786285,-0.619521972479176));
#17911=CARTESIAN_POINT('Ctrl Pts',(93.8547136670615,-2.08766421985139,-0.713411240246326));
#17912=CARTESIAN_POINT('Ctrl Pts',(93.8614788548914,-2.04322166096454,-0.826682129239053));
#17913=CARTESIAN_POINT('Ctrl Pts',(93.8627619781991,-2.03437444063568,-0.848220957466346));
#17914=CARTESIAN_POINT('Ctrl Pts',(93.8648037814182,-2.01962308149178,-0.882574350665131));
#17915=CARTESIAN_POINT('Ctrl Pts',(93.8655696964814,-2.01393449846335,-0.895479047573452));
#17916=CARTESIAN_POINT('Ctrl Pts',(93.8670232617706,-2.00284290995776,-0.920000206486861));
#17917=CARTESIAN_POINT('Ctrl Pts',(93.8677116233329,-1.99746173326652,-0.931625856041603));
#17918=CARTESIAN_POINT('Ctrl Pts',(93.8692711769825,-1.98497820086649,-0.957990181228405));
#17919=CARTESIAN_POINT('Ctrl Pts',(93.8701401323573,-1.97781244231909,-0.972698107199681));
#17920=CARTESIAN_POINT('Ctrl Pts',(93.8728735893441,-1.95461025346047,-1.01900456336722));
#17921=CARTESIAN_POINT('Ctrl Pts',(93.8747171890475,-1.93797487822762,-1.05029762341759));
#17922=CARTESIAN_POINT('Ctrl Pts',(93.8855563538931,-1.83445282090702,-1.23419309803679));
#17923=CARTESIAN_POINT('Ctrl Pts',(93.8938938184469,-1.73034073615046,-1.3763624272371));
#17924=CARTESIAN_POINT('Ctrl Pts',(93.9070541069621,-1.54542852665354,-1.57427418794442));
#17925=CARTESIAN_POINT('Ctrl Pts',(93.9117404827267,-1.47596349815318,-1.63957828421042));
#17926=CARTESIAN_POINT('Ctrl Pts',(93.9177885045925,-1.38639995059095,-1.71346047977437));
#17927=CARTESIAN_POINT('Ctrl Pts',(93.9188887330871,-1.37011191383643,-1.72651235727779));
#17928=CARTESIAN_POINT('Ctrl Pts',(93.9205095559644,-1.34618302383223,-1.74513512090484));
#17929=CARTESIAN_POINT('Ctrl Pts',(93.9210178990036,-1.3386873540474,-1.75089162582198));
#17930=CARTESIAN_POINT('Ctrl Pts',(93.9219149451999,-1.32548280182915,-1.7608980642651));
#17931=CARTESIAN_POINT('Ctrl Pts',(93.922302192393,-1.31979002257752,-1.76516881504841));
#17932=CARTESIAN_POINT('Ctrl Pts',(93.9231501574687,-1.30734240366863,-1.77441319855071));
#17933=CARTESIAN_POINT('Ctrl Pts',(93.9236115733144,-1.30057992844843,-1.77937579070851));
#17934=CARTESIAN_POINT('Ctrl Pts',(93.9249066083704,-1.28162432728128,-1.79312043108407));
#17935=CARTESIAN_POINT('Ctrl Pts',(93.9257457372506,-1.26936969459584,-1.80181640290108));
#17936=CARTESIAN_POINT('Ctrl Pts',(93.9313567372293,-1.18753258469663,-1.85863935991779));
#17937=CARTESIAN_POINT('Ctrl Pts',(93.936339722643,-1.11532292312177,-1.90284683080483));
#17938=CARTESIAN_POINT('Ctrl Pts',(93.9432173894367,-1.01377566049741,-1.9572460165996));
#17939=CARTESIAN_POINT('Ctrl Pts',(93.9450533276944,-0.986494221072495,
-1.9711372791156));
#17940=CARTESIAN_POINT('Ctrl Pts',(93.9523657579225,-0.876857260786852,
-2.024116269418));
#17941=CARTESIAN_POINT('Ctrl Pts',(93.9578493012834,-0.792396846609868,
-2.05864856761366));
#17942=CARTESIAN_POINT('Ctrl Pts',(93.9687685622576,-0.616896794506573,
-2.11799650474594));
#17943=CARTESIAN_POINT('Ctrl Pts',(93.974185283782,-0.525908952390281,-2.14240382860225));
#17944=CARTESIAN_POINT('Ctrl Pts',(93.9806962797359,-0.411050054205773,
-2.16545242759511));
#17945=CARTESIAN_POINT('Ctrl Pts',(93.9819650851626,-0.38840036454108,-2.16962936395374));
#17946=CARTESIAN_POINT('Ctrl Pts',(93.9839897050202,-0.351835552883299,
-2.17578148887631));
#17947=CARTESIAN_POINT('Ctrl Pts',(93.9847525397047,-0.337960179352446,
-2.17797986070288));
#17948=CARTESIAN_POINT('Ctrl Pts',(93.986203738612,-0.311379228581965,-2.18193112815227));
#17949=CARTESIAN_POINT('Ctrl Pts',(93.9868927736704,-0.298677555354851,
-2.1837060698626));
#17950=CARTESIAN_POINT('Ctrl Pts',(93.9884585665339,-0.269633472078678,
-2.18750655792812));
#17951=CARTESIAN_POINT('Ctrl Pts',(93.9893330209238,-0.253282303271566,
-2.18946003502315));
#17952=CARTESIAN_POINT('Ctrl Pts',(93.9916537746351,-0.209552615840613,
-2.19418798245453));
#17953=CARTESIAN_POINT('Ctrl Pts',(93.9930898070505,-0.182141035067087,
-2.19663331752821));
#17954=CARTESIAN_POINT('Ctrl Pts',(94.0029344693662,0.00797648378945016,
-2.21000990056251));
#17955=CARTESIAN_POINT('Ctrl Pts',(94.0107648160588,0.171409596627473,-2.20336810998709));
#17956=CARTESIAN_POINT('Ctrl Pts',(94.0245877026155,0.453859778231991,-2.16024713040359));
#17957=CARTESIAN_POINT('Ctrl Pts',(94.0305477676455,0.573324585697993,-2.13165390454477));
#17958=CARTESIAN_POINT('Ctrl Pts',(94.0378430418371,0.705201650376367,-2.08819788718577));
#17959=CARTESIAN_POINT('Ctrl Pts',(94.0387047123868,0.720570069862809,-2.08294467699216));
#17960=CARTESIAN_POINT('Ctrl Pts',(94.040034701388,0.743941466074856,-2.07466630129696));
#17961=CARTESIAN_POINT('Ctrl Pts',(94.0404961534403,0.751987525150952,-2.07176348160489));
#17962=CARTESIAN_POINT('Ctrl Pts',(94.0413492784867,0.766742012563689,-2.06634315291636));
#17963=CARTESIAN_POINT('Ctrl Pts',(94.0417401327836,0.773455299553895,-2.0638396824325));
#17964=CARTESIAN_POINT('Ctrl Pts',(94.0426404568422,0.78881407163978,-2.05802673819502));
#17965=CARTESIAN_POINT('Ctrl Pts',(94.0431511823327,0.797450980293317,-2.05469550601569));
#17966=CARTESIAN_POINT('Ctrl Pts',(94.0447645051604,0.824507919163155,-2.04406342634091));
#17967=CARTESIAN_POINT('Ctrl Pts',(94.0458777428487,0.842850147761035,-2.03656872513847));
#17968=CARTESIAN_POINT('Ctrl Pts',(94.0548525469806,0.98837693284134,-1.97480331619096));
#17969=CARTESIAN_POINT('Ctrl Pts',(94.0632251370994,1.11029020981144,-1.90892320942486));
#17970=CARTESIAN_POINT('Ctrl Pts',(94.0805647689565,1.35048371035123,-1.74829025427942));
#17971=CARTESIAN_POINT('Ctrl Pts',(94.0894594166803,1.46684413759872,-1.65187973913397));
#17972=CARTESIAN_POINT('Ctrl Pts',(94.0992736410334,1.59018483655103,-1.52629210731244));
#17973=CARTESIAN_POINT('Ctrl Pts',(94.1006701061558,1.60759173424973,-1.50794704894518));
#17974=CARTESIAN_POINT('Ctrl Pts',(94.1028476770273,1.63449857853355,-1.47859444911243));
#17975=CARTESIAN_POINT('Ctrl Pts',(94.1036378074455,1.64421153849958,-1.46778594456842));
#17976=CARTESIAN_POINT('Ctrl Pts',(94.1051118608522,1.66223382036615,-1.447327487709));
#17977=CARTESIAN_POINT('Ctrl Pts',(94.1057967983012,1.67056774053059,-1.43770009528951));
#17978=CARTESIAN_POINT('Ctrl Pts',(94.1073297269656,1.68912482913058,-1.41588360153803));
#17979=CARTESIAN_POINT('Ctrl Pts',(94.1081757492044,1.69930045788661,-1.40365488397305));
#17980=CARTESIAN_POINT('Ctrl Pts',(94.1106557845079,1.72892265395412,-1.36726166907725));
#17981=CARTESIAN_POINT('Ctrl Pts',(94.1122747777999,1.74799294552133,-1.3427951453298));
#17982=CARTESIAN_POINT('Ctrl Pts',(94.1212575445019,1.85208896335321,-1.20326617332785));
#17983=CARTESIAN_POINT('Ctrl Pts',(94.1281964835753,1.92627094073789,-1.08054061348735));
#17984=CARTESIAN_POINT('Ctrl Pts',(94.139943922966,2.03120116212142,-0.861297729753891));
#17985=CARTESIAN_POINT('Ctrl Pts',(94.1447598715132,2.06817413754088,-0.768287312700597));
#17986=CARTESIAN_POINT('Ctrl Pts',(94.1513976595986,2.10844196122829,-0.642732600990195));
#17987=CARTESIAN_POINT('Ctrl Pts',(94.1530244959375,2.11751933703716,-0.612163694157456));
#17988=CARTESIAN_POINT('Ctrl Pts',(94.1558392275181,2.1318071349637,-0.559920251272809));
#17989=CARTESIAN_POINT('Ctrl Pts',(94.1570115627271,2.13735785235526,-0.538343463206542));
#17990=CARTESIAN_POINT('Ctrl Pts',(94.1587193841732,2.14485416879634,-0.507257994039228));
#17991=CARTESIAN_POINT('Ctrl Pts',(94.1592407034452,2.1470656975113,-0.49781418358351));
#17992=CARTESIAN_POINT('Ctrl Pts',(94.1601556393773,2.15081203668273,-0.481326860457285));
#17993=CARTESIAN_POINT('Ctrl Pts',(94.1605476723756,2.1523747369622,-0.474289947609504));
#17994=CARTESIAN_POINT('Ctrl Pts',(94.1613933439577,2.15565429229551,-0.459171884046771));
#17995=CARTESIAN_POINT('Ctrl Pts',(94.1618475495867,2.15736021605881,-0.451088838901748));
#17996=CARTESIAN_POINT('Ctrl Pts',(94.1631036262067,2.16192742783788,-0.428829738088441));
#17997=CARTESIAN_POINT('Ctrl Pts',(94.1639105095529,2.1646946421005,-0.414635057934217));
#17998=CARTESIAN_POINT('Ctrl Pts',(94.1685679884974,2.17973604137456,-0.333220552503686));
#17999=CARTESIAN_POINT('Ctrl Pts',(94.172556682083,2.18901761289181,-0.265490960917877));
#18000=CARTESIAN_POINT('Ctrl Pts',(94.1844734322497,2.20701701245976,-0.0653798293045088));
#18001=CARTESIAN_POINT('Ctrl Pts',(94.1925365281866,2.20695399425554,0.0674903382250955));
#18002=CARTESIAN_POINT('Ctrl Pts',(94.2062816590316,2.18589862653696,0.29908431293463));
#18003=CARTESIAN_POINT('Ctrl Pts',(94.2120499840789,2.17008973345864,0.397893181607666));
#18004=CARTESIAN_POINT('Ctrl Pts',(94.2189080683085,2.14237349742451,0.518071411255271));
#18005=CARTESIAN_POINT('Ctrl Pts',(94.2201961472389,2.13675944818476,0.540759937165932));
#18006=CARTESIAN_POINT('Ctrl Pts',(94.2222438966813,2.12717597949967,0.577007590527999));
#18007=CARTESIAN_POINT('Ctrl Pts',(94.223010877303,2.1234353477289,0.590624876171923));
#18008=CARTESIAN_POINT('Ctrl Pts',(94.2244652758879,2.11605352943742,0.616520430960001));
#18009=CARTESIAN_POINT('Ctrl Pts',(94.2251534190728,2.11243570993544,0.628804709127454));
#18010=CARTESIAN_POINT('Ctrl Pts',(94.226710884999,2.10396296895939,0.656675184817543));
#18011=CARTESIAN_POINT('Ctrl Pts',(94.2275779934023,2.0990415063573,0.672240468187701));
#18012=CARTESIAN_POINT('Ctrl Pts',(94.2302991953238,2.08295309983159,0.721223793201713));
#18013=CARTESIAN_POINT('Ctrl Pts',(94.2321326604006,2.07115727393851,0.754430316823035));
#18014=CARTESIAN_POINT('Ctrl Pts',(94.2429753738849,1.99576192884313,0.951557843751273));
#18015=CARTESIAN_POINT('Ctrl Pts',(94.2513236441277,1.9135334541249,1.10766447716915));
#18016=CARTESIAN_POINT('Ctrl Pts',(94.2644978449376,1.75946372857195,1.33078522260906));
#18017=CARTESIAN_POINT('Ctrl Pts',(94.2691874362034,1.70027463848923,1.40561897996181));
#18018=CARTESIAN_POINT('Ctrl Pts',(94.2752394002679,1.62244897398795,1.4918817827717));
#18019=CARTESIAN_POINT('Ctrl Pts',(94.2763399829783,1.60824390305983,1.50718393459308));
#18020=CARTESIAN_POINT('Ctrl Pts',(94.2779612342288,1.58729544461619,1.52911690818725));
#18021=CARTESIAN_POINT('Ctrl Pts',(94.2784696423442,1.58072299537368,1.53591020332835));
#18022=CARTESIAN_POINT('Ctrl Pts',(94.2793667602288,1.56912568381353,1.54774391967337));
#18023=CARTESIAN_POINT('Ctrl Pts',(94.2797540132216,1.56411981085483,1.55280258514089));
#18024=CARTESIAN_POINT('Ctrl Pts',(94.2806019380651,1.55316108867777,1.56377011688736));
#18025=CARTESIAN_POINT('Ctrl Pts',(94.2810633072883,1.54719907656801,1.56966918761325));
#18026=CARTESIAN_POINT('Ctrl Pts',(94.2823580891429,1.5304645201801,1.58603910378772));
#18027=CARTESIAN_POINT('Ctrl Pts',(94.2831970081457,1.51961856951106,1.59643385837314));
#18028=CARTESIAN_POINT('Ctrl Pts',(94.288800145217,1.44708944027138,1.66453693218984));
#18029=CARTESIAN_POINT('Ctrl Pts',(94.293774811282,1.38224359951118,1.71876439983942));
#18030=CARTESIAN_POINT('Ctrl Pts',(94.3007199893729,1.28886147607454,1.78814669180442));
#18031=CARTESIAN_POINT('Ctrl Pts',(94.3026324622335,1.26286031742984,1.806603518381));
#18032=CARTESIAN_POINT('Ctrl Pts',(94.3100816727387,1.1601843201433,1.87618769637456));
#18033=CARTESIAN_POINT('Ctrl Pts',(94.3156234931547,1.08072965325937,1.92305299036714));
#18034=CARTESIAN_POINT('Ctrl Pts',(94.3264792402995,0.916373831894321,2.00658333779552));
#18035=CARTESIAN_POINT('Ctrl Pts',(94.3317821913897,0.831628499643467,2.04316300673931));
#18036=CARTESIAN_POINT('Ctrl Pts',(94.3381800540566,0.723269182191769,2.08207170247906));
#18037=CARTESIAN_POINT('Ctrl Pts',(94.3394421217506,0.701586789984342,2.08947766589662));
#18038=CARTESIAN_POINT('Ctrl Pts',(94.341458653904,0.666453631418346,2.10086938712543));
#18039=CARTESIAN_POINT('Ctrl Pts',(94.3422200383473,0.65307381631619,2.10506703641674));
#18040=CARTESIAN_POINT('Ctrl Pts',(94.3436701460033,0.627375033145629,2.11286091010195));
#18041=CARTESIAN_POINT('Ctrl Pts',(94.3443595207881,0.61506297278531,2.11647778320735));
#18042=CARTESIAN_POINT('Ctrl Pts',(94.3459283606194,0.586830930631863,2.12450425327059));
#18043=CARTESIAN_POINT('Ctrl Pts',(94.3468054897548,0.570891456146901,2.1288428379435));
#18044=CARTESIAN_POINT('Ctrl Pts',(94.34913842456,0.52809549635576,2.13997628649839));
#18045=CARTESIAN_POINT('Ctrl Pts',(94.3505837868944,0.50115675532425,2.14644481771647));
#18046=CARTESIAN_POINT('Ctrl Pts',(94.3602477325801,0.318402464875393,2.18669945921583));
#18047=CARTESIAN_POINT('Ctrl Pts',(94.3679174200527,0.159443559683195,2.20399999999185));
#18048=CARTESIAN_POINT('Ctrl Pts',(94.3756281550323,1.1263660143479E-10,
2.204));
#18049=CARTESIAN_POINT('Origin',(66.9212607628943,0.,0.));
#18050=CARTESIAN_POINT('',(95.2361698906488,-1.9935815181446E-11,2.204));
#18051=CARTESIAN_POINT('',(95.1243866264839,2.95873024051195E-11,2.204));
#18052=CARTESIAN_POINT('',(66.9212607628943,-2.69912154532077E-16,2.204));
#18053=CARTESIAN_POINT('',(95.2361199581431,0.000963537602863376,2.20400005961913));
#18054=CARTESIAN_POINT('Ctrl Pts',(95.2361698906488,-1.9935815181446E-11,
2.204));
#18055=CARTESIAN_POINT('Ctrl Pts',(95.2361534167709,0.000320954503179185,
2.204));
#18056=CARTESIAN_POINT('Ctrl Pts',(95.2361369400511,0.000641910946360297,
2.20399992989215));
#18057=CARTESIAN_POINT('Ctrl Pts',(95.2361204604807,0.000962869286795163,
2.20399978967393));
#18058=CARTESIAN_POINT('Ctrl Pts',(95.2361204249416,0.000963561450979549,
2.20399978937144));
#18059=CARTESIAN_POINT('Ctrl Pts',(95.235034291354,0.0221172408984992,2.20399054124439));
#18060=CARTESIAN_POINT('Ctrl Pts',(95.2339362974794,0.0432690499204987,
2.20367674869492));
#18061=CARTESIAN_POINT('Ctrl Pts',(95.2320670260183,0.0787998801185974,
2.20263790837682));
#18062=CARTESIAN_POINT('Ctrl Pts',(95.2313035034934,0.0931825240550623,
2.2020763320936));
#18063=CARTESIAN_POINT('Ctrl Pts',(95.2301493654033,0.114704524566008,2.20102477565529));
#18064=CARTESIAN_POINT('Ctrl Pts',(95.2297643210824,0.121848945618526,2.20064082089274));
#18065=CARTESIAN_POINT('Ctrl Pts',(95.2290094347842,0.135782261522555,2.19982395966916));
#18066=CARTESIAN_POINT('Ctrl Pts',(95.2286397739114,0.142571301378628,2.19939439381365));
#18067=CARTESIAN_POINT('Ctrl Pts',(95.2278371408031,0.157236031786589,2.19839832052389));
#18068=CARTESIAN_POINT('Ctrl Pts',(95.2274035867278,0.16511073059419,2.19782091809055));
#18069=CARTESIAN_POINT('Ctrl Pts',(95.2262281816644,0.1863403244267,2.19614954718092));
#18070=CARTESIAN_POINT('Ctrl Pts',(95.2254821220025,0.199688415309678,2.19497609750168));
#18071=CARTESIAN_POINT('Ctrl Pts',(95.2219143401863,0.262972317062414,2.18883070555597));
#18072=CARTESIAN_POINT('Ctrl Pts',(95.2190182477043,0.312736353958185,2.18227623078205));
#18073=CARTESIAN_POINT('Ctrl Pts',(95.2078279590943,0.50090670280392,2.15092392354501));
#18074=CARTESIAN_POINT('Ctrl Pts',(95.1992580400119,0.637053700804592,2.11460271663876));
#18075=CARTESIAN_POINT('Ctrl Pts',(95.1842853950377,0.873312631742267,2.0266656605574));
#18076=CARTESIAN_POINT('Ctrl Pts',(95.1778175205937,0.974718920767726,1.97989328345489));
#18077=CARTESIAN_POINT('Ctrl Pts',(95.1702883970305,1.09294492822253,1.9140672095617));
#18078=CARTESIAN_POINT('Ctrl Pts',(95.1689766546022,1.11354092839653,1.90215892140788));
#18079=CARTESIAN_POINT('Ctrl Pts',(95.166905421712,1.14604929658732,1.88265408658885));
#18080=CARTESIAN_POINT('Ctrl Pts',(95.1661382050772,1.15808799446417,1.87527267619657));
#18081=CARTESIAN_POINT('Ctrl Pts',(95.1646919929783,1.18077148234855,1.8610627645891));
#18082=CARTESIAN_POINT('Ctrl Pts',(95.1640121848691,1.19143001854378,1.85425737895985));
#18083=CARTESIAN_POINT('Ctrl Pts',(95.1624710440022,1.21557934301188,1.83854404035458));
#18084=CARTESIAN_POINT('Ctrl Pts',(95.1616119025858,1.22903195962704,1.82957858222485));
#18085=CARTESIAN_POINT('Ctrl Pts',(95.1593772704201,1.26398298200435,1.80572610132774));
#18086=CARTESIAN_POINT('Ctrl Pts',(95.1580107170575,1.28531753391579,1.79060287168786));
#18087=CARTESIAN_POINT('Ctrl Pts',(95.1474854028872,1.44912051622182,1.67005286316826));
#18088=CARTESIAN_POINT('Ctrl Pts',(95.139031833913,1.578667907882,1.54817277635287));
#18089=CARTESIAN_POINT('Ctrl Pts',(95.12498508029,1.76430809959199,1.3257037696467));
#18090=CARTESIAN_POINT('Ctrl Pts',(95.1194754492507,1.82966199575958,1.23393876170364));
#18091=CARTESIAN_POINT('Ctrl Pts',(95.1127469769345,1.89564245244932,1.12445157263748));
#18092=CARTESIAN_POINT('Ctrl Pts',(95.1119314307482,1.90342799846769,1.11122161389339));
#18093=CARTESIAN_POINT('Ctrl Pts',(95.110660901158,1.91521738037532,1.09070048692753));
#18094=CARTESIAN_POINT('Ctrl Pts',(95.1102119395426,1.91931934800904,1.08346592102867));
#18095=CARTESIAN_POINT('Ctrl Pts',(95.1093742688837,1.92685179073015,1.07000407594121));
#18096=CARTESIAN_POINT('Ctrl Pts',(95.1089862571221,1.93029319280301,1.06378321624338));
#18097=CARTESIAN_POINT('Ctrl Pts',(95.1080913765542,1.93812198763543,1.04946839923132));
#18098=CARTESIAN_POINT('Ctrl Pts',(95.1075832542255,1.94248881721917,1.04136350459573));
#18099=CARTESIAN_POINT('Ctrl Pts',(95.1059412231075,1.95635519134849,1.01523662197354));
#18100=CARTESIAN_POINT('Ctrl Pts',(95.1047958887181,1.96565542105491,0.997110695217857));
#18101=CARTESIAN_POINT('Ctrl Pts',(95.0963711596122,2.03150955616834,0.86425977290282));
#18102=CARTESIAN_POINT('Ctrl Pts',(95.0886566902527,2.07822856813308,0.744941207618189));
#18103=CARTESIAN_POINT('Ctrl Pts',(95.0744496687078,2.1450114881738,0.518022526023417));
#18104=CARTESIAN_POINT('Ctrl Pts',(95.067965488725,2.16794032957263,0.41165531179129));
#18105=CARTESIAN_POINT('Ctrl Pts',(95.0593128611373,2.18860861591518,0.263254048796924));
#18106=CARTESIAN_POINT('Ctrl Pts',(95.0569660405474,2.19314365740099,0.222332115690185));
#18107=CARTESIAN_POINT('Ctrl Pts',(95.0528875336054,2.19911568941843,0.149980388134773));
#18108=CARTESIAN_POINT('Ctrl Pts',(95.0511420358666,2.2010310004753,0.118602744839227));
#18109=CARTESIAN_POINT('Ctrl Pts',(95.0485564715739,2.2028953475529,0.0715144192108333));
#18110=CARTESIAN_POINT('Ctrl Pts',(95.0477008013508,2.20334867824945,0.0558287062442669));
#18111=CARTESIAN_POINT('Ctrl Pts',(95.0461737218198,2.20386184573531,0.0276559062943479));
#18112=CARTESIAN_POINT('Ctrl Pts',(95.0455004185594,2.20398315373905,0.0151707356315025));
#18113=CARTESIAN_POINT('Ctrl Pts',(95.0440587550774,2.20401588316389,-0.0116951525354532));
#18114=CARTESIAN_POINT('Ctrl Pts',(95.0432915092199,2.20389266473295,-0.0260753822545955));
#18115=CARTESIAN_POINT('Ctrl Pts',(95.0412362449073,2.2031816044467,-0.064808951448164));
#18116=CARTESIAN_POINT('Ctrl Pts',(95.0399564557445,2.20233073985652,-0.0891558005461899));
#18117=CARTESIAN_POINT('Ctrl Pts',(95.0315932389294,2.19405778963238,-0.249613337088624));
#18118=CARTESIAN_POINT('Ctrl Pts',(95.0249103787182,2.17442615927617,-0.384802077922835));
#18119=CARTESIAN_POINT('Ctrl Pts',(95.0130030172164,2.11669629057034,-0.623882905709597));
#18120=CARTESIAN_POINT('Ctrl Pts',(95.007758015422,2.08305285455629,-0.728369063763963));
#18121=CARTESIAN_POINT('Ctrl Pts',(95.0004310549454,2.02786269836783,-0.864149695421951));
#18122=CARTESIAN_POINT('Ctrl Pts',(94.9985573938579,2.01308827797242,-0.898029597374532));
#18123=CARTESIAN_POINT('Ctrl Pts',(94.9953613567737,1.98699335988482,-0.953985225592102));
#18124=CARTESIAN_POINT('Ctrl Pts',(94.9940607935359,1.97613909571453,-0.97627075955252));
#18125=CARTESIAN_POINT('Ctrl Pts',(94.9922023792946,1.96035647797519,-1.00733291792418));
#18126=CARTESIAN_POINT('Ctrl Pts',(94.9916624810694,1.9557399792254,-1.01626682227587));
#18127=CARTESIAN_POINT('Ctrl Pts',(94.9907294643382,1.94771303597018,-1.03154340022193));
#18128=CARTESIAN_POINT('Ctrl Pts',(94.9903381850216,1.94433229484852,-1.03790162519033));
#18129=CARTESIAN_POINT('Ctrl Pts',(94.9895111156178,1.93715754938451,-1.05123722563457));
#18130=CARTESIAN_POINT('Ctrl Pts',(94.989074936077,1.93335694718378,-1.05821074762367));
#18131=CARTESIAN_POINT('Ctrl Pts',(94.9878850716683,1.92294107939062,-1.07707884950993));
#18132=CARTESIAN_POINT('Ctrl Pts',(94.9871270062952,1.91625329581452,-1.08893274816912));
#18133=CARTESIAN_POINT('Ctrl Pts',(94.9834050139651,1.88314172091705,-1.146372330892));
#18134=CARTESIAN_POINT('Ctrl Pts',(94.9803590507822,1.85520046105624,-1.19105948231881));
#18135=CARTESIAN_POINT('Ctrl Pts',(94.9700425056672,1.75685411846685,-1.33647926243897));
#18136=CARTESIAN_POINT('Ctrl Pts',(94.9625800219913,1.67963161745368,-1.43232346963056));
#18137=CARTESIAN_POINT('Ctrl Pts',(94.9477658579539,1.50829172585012,-1.61195230976075));
#18138=CARTESIAN_POINT('Ctrl Pts',(94.9404493399489,1.4141655600777,-1.69513360243851));
#18139=CARTESIAN_POINT('Ctrl Pts',(94.9321142539047,1.29395568143355,-1.78434436404062));
#18140=CARTESIAN_POINT('Ctrl Pts',(94.9307740328803,1.27420983714685,-1.79849811582516));
#18141=CARTESIAN_POINT('Ctrl Pts',(94.9286686732144,1.24253326774592,-1.82042015417996));
#18142=CARTESIAN_POINT('Ctrl Pts',(94.9278953630936,1.23075475787889,-1.82840400309037));
#18143=CARTESIAN_POINT('Ctrl Pts',(94.9264439770461,1.20837981936524,-1.84325625942839));
#18144=CARTESIAN_POINT('Ctrl Pts',(94.9257650131254,1.1978001204572,-1.85014872548477));
#18145=CARTESIAN_POINT('Ctrl Pts',(94.9242342025997,1.17369472654239,-1.86555947889423));
#18146=CARTESIAN_POINT('Ctrl Pts',(94.9233844331037,1.16013434525974,-1.87402235834642));
#18147=CARTESIAN_POINT('Ctrl Pts',(94.9211913374608,1.12468187317863,-1.89561554201962));
#18148=CARTESIAN_POINT('Ctrl Pts',(94.9198563984633,1.10265130626867,-1.90851454435554));
#18149=CARTESIAN_POINT('Ctrl Pts',(94.9090749537497,0.921226363175545,-2.0105493212117));
#18150=CARTESIAN_POINT('Ctrl Pts',(94.9003864863108,0.751548646407268,-2.07993878901998));
#18151=CARTESIAN_POINT('Ctrl Pts',(94.8862642060755,0.470631081367228,-2.15589117266787));
#18152=CARTESIAN_POINT('Ctrl Pts',(94.8809422137238,0.364083155954069,-2.17641876824584));
#18153=CARTESIAN_POINT('Ctrl Pts',(94.874433432658,0.241279882483361,-2.19080669527446));
#18154=CARTESIAN_POINT('Ctrl Pts',(94.8736207425861,0.226070421096619,-2.19242835607495));
#18155=CARTESIAN_POINT('Ctrl Pts',(94.872353729714,0.202578854612774,-2.19468603227857));
#18156=CARTESIAN_POINT('Ctrl Pts',(94.8719053762367,0.194307682139324,-2.19543378235174));
#18157=CARTESIAN_POINT('Ctrl Pts',(94.871068210702,0.178946681053206,-2.19673499907297));
#18158=CARTESIAN_POINT('Ctrl Pts',(94.8706800876153,0.1718581742011,-2.19730092024401));
#18159=CARTESIAN_POINT('Ctrl Pts',(94.8697841413254,0.155569351669554,-2.19852206051814));
#18160=CARTESIAN_POINT('Ctrl Pts',(94.8692750536711,0.146367547925755,-2.1991538391913));
#18161=CARTESIAN_POINT('Ctrl Pts',(94.8676680549721,0.117477854212301,-2.20095523229551));
#18162=CARTESIAN_POINT('Ctrl Pts',(94.8665596339758,0.0977785833283383,
-2.20191831693362));
#18163=CARTESIAN_POINT('Ctrl Pts',(94.8577161902663,-0.0578669185339179,
-2.20743503057469));
#18164=CARTESIAN_POINT('Ctrl Pts',(94.8494870869832,-0.193948241748064,
-2.1996584259774));
#18165=CARTESIAN_POINT('Ctrl Pts',(94.8321449184953,-0.479651929512035,
-2.15660294673373));
#18166=CARTESIAN_POINT('Ctrl Pts',(94.8231113219096,-0.628109524122365,
-2.11813469312318));
#18167=CARTESIAN_POINT('Ctrl Pts',(94.8131805211587,-0.794983783736224,
-2.05578460829656));
#18168=CARTESIAN_POINT('Ctrl Pts',(94.8117905862858,-0.818410555507513,
-2.04657123231314));
#18169=CARTESIAN_POINT('Ctrl Pts',(94.8096257451738,-0.85499860784024,-2.03145297895365));
#18170=CARTESIAN_POINT('Ctrl Pts',(94.8088418661278,-0.86826802523822,-2.02581698960101));
#18171=CARTESIAN_POINT('Ctrl Pts',(94.8073810912693,-0.893031026706379,
-2.01501126026169));
#18172=CARTESIAN_POINT('Ctrl Pts',(94.8067031798594,-0.904537362872433,
-2.00987237454781));
#18173=CARTESIAN_POINT('Ctrl Pts',(94.805188253072,-0.930278418503375,-1.99811024067187));
#18174=CARTESIAN_POINT('Ctrl Pts',(94.804353136375,-0.944487792810443,-1.99143297560836));
#18175=CARTESIAN_POINT('Ctrl Pts',(94.8019131369097,-0.986046874456804,
-1.97135866241666));
#18176=CARTESIAN_POINT('Ctrl Pts',(94.8003226844289,-1.01319221663068,-1.95754567382915));
#18177=CARTESIAN_POINT('Ctrl Pts',(94.7906560052066,-1.17824084975404,-1.86920682850032));
#18178=CARTESIAN_POINT('Ctrl Pts',(94.7831046846063,-1.3081539053577,-1.78070884483692));
#18179=CARTESIAN_POINT('Ctrl Pts',(94.7692489477125,-1.5264897961657,-1.59508518032524));
#18180=CARTESIAN_POINT('Ctrl Pts',(94.7629644610338,-1.6177585434519,-1.50243703220189));
#18181=CARTESIAN_POINT('Ctrl Pts',(94.7553208821739,-1.71017706520948,-1.39037754629946));
#18182=CARTESIAN_POINT('Ctrl Pts',(94.7544991678363,-1.71989366412518,-1.37833997001578));
#18183=CARTESIAN_POINT('Ctrl Pts',(94.7532210452214,-1.73465329049182,-1.35965567199704));
#18184=CARTESIAN_POINT('Ctrl Pts',(94.7527707727349,-1.73978682458111,-1.35308070157673));
#18185=CARTESIAN_POINT('Ctrl Pts',(94.7519320023424,-1.74922405065409,-1.34085111620507));
#18186=CARTESIAN_POINT('Ctrl Pts',(94.7515442195634,-1.75353786264935,-1.33520464908103));
#18187=CARTESIAN_POINT('Ctrl Pts',(94.7506515887248,-1.76335625653888,-1.32222343418918));
#18188=CARTESIAN_POINT('Ctrl Pts',(94.7501455103028,-1.76884242930961,-1.31487510871631));
#18189=CARTESIAN_POINT('Ctrl Pts',(94.7485167790847,-1.78624953605257,-1.29125347018468));
#18190=CARTESIAN_POINT('Ctrl Pts',(94.7473829486007,-1.79799264936999,-1.27485109064596));
#18191=CARTESIAN_POINT('Ctrl Pts',(94.7386147721744,-1.88612396260674,-1.14811217772825));
#18192=CARTESIAN_POINT('Ctrl Pts',(94.7305011038329,-1.95251109037437,-1.03117447493581));
#18193=CARTESIAN_POINT('Ctrl Pts',(94.7161772305613,-2.05091244200055,-0.813805043572388));
#18194=CARTESIAN_POINT('Ctrl Pts',(94.7099584429775,-2.0871653996624,-0.715726568664627));
#18195=CARTESIAN_POINT('Ctrl Pts',(94.700467685991,-2.13310644386122,-0.557747925577904));
#18196=CARTESIAN_POINT('Ctrl Pts',(94.6970678167327,-2.14751854418209,-0.499390552193682));
#18197=CARTESIAN_POINT('Ctrl Pts',(94.6926375361158,-2.16352444776319,-0.42092472794631));
#18198=CARTESIAN_POINT('Ctrl Pts',(94.6915400276347,-2.16725354628873,-0.401282650983361));
#18199=CARTESIAN_POINT('Ctrl Pts',(94.6897258679657,-2.17301980079748,-0.368480883056216));
#18200=CARTESIAN_POINT('Ctrl Pts',(94.6890045276649,-2.17520583035337,-0.355348874123209));
#18201=CARTESIAN_POINT('Ctrl Pts',(94.687595971072,-2.17926312204301,-0.329533879403545));
#18202=CARTESIAN_POINT('Ctrl Pts',(94.6869085083772,-2.18114296809764,-0.316852797178928));
#18203=CARTESIAN_POINT('Ctrl Pts',(94.6852567345983,-2.18541516806019,-0.286191420545203));
#18204=CARTESIAN_POINT('Ctrl Pts',(94.6842959584682,-2.18769643320147,-0.268196436409533));
#18205=CARTESIAN_POINT('Ctrl Pts',(94.6811038473573,-2.19458532623544,-0.207898676397314));
#18206=CARTESIAN_POINT('Ctrl Pts',(94.6789037521193,-2.19819017653519,-0.165489784054177));
#18207=CARTESIAN_POINT('Ctrl Pts',(94.6682138190484,-2.20990147646216,0.0440323985060621));
#18208=CARTESIAN_POINT('Ctrl Pts',(94.6602776964772,-2.20019065038445,0.21158057162421));
#18209=CARTESIAN_POINT('Ctrl Pts',(94.6476357512053,-2.15579778035772,0.467687398990503));
#18210=CARTESIAN_POINT('Ctrl Pts',(94.6430693362984,-2.13424191325306,0.557856511142384));
#18211=CARTESIAN_POINT('Ctrl Pts',(94.6371721881968,-2.10106050872926,0.66601966144325));
#18212=CARTESIAN_POINT('Ctrl Pts',(94.6360895178568,-2.09476593540462,0.685560403608739));
#18213=CARTESIAN_POINT('Ctrl Pts',(94.6344928787604,-2.08521386756964,0.713853099137779));
#18214=CARTESIAN_POINT('Ctrl Pts',(94.6339907527263,-2.08217208954237,0.722677316518574));
#18215=CARTESIAN_POINT('Ctrl Pts',(94.6331039767517,-2.07673696826687,0.738125440852542));
#18216=CARTESIAN_POINT('Ctrl Pts',(94.6327207399044,-2.07436779439653,0.74475758070498));
#18217=CARTESIAN_POINT('Ctrl Pts',(94.6318811041838,-2.06913384529123,0.759190479382962));
#18218=CARTESIAN_POINT('Ctrl Pts',(94.631424015605,-2.06625677266356,0.766986309193326));
#18219=CARTESIAN_POINT('Ctrl Pts',(94.6301405320204,-2.05809859330971,0.788712963103273));
#18220=CARTESIAN_POINT('Ctrl Pts',(94.6293087134069,-2.05272031400722,0.802606532306444));
#18221=CARTESIAN_POINT('Ctrl Pts',(94.6237780017179,-2.01633326036626,0.893845649029568));
#18222=CARTESIAN_POINT('Ctrl Pts',(94.6188738690157,-1.98110259542662,0.969427575944329));
#18223=CARTESIAN_POINT('Ctrl Pts',(94.6119866657102,-1.92649429640844,1.07110508175645));
#18224=CARTESIAN_POINT('Ctrl Pts',(94.6100616094788,-1.9106906086445,1.09904855367106));
#18225=CARTESIAN_POINT('Ctrl Pts',(94.6026644779208,-1.84772537843845,1.20491581884325));
#18226=CARTESIAN_POINT('Ctrl Pts',(94.5971856007205,-1.79635878213794,1.28023735504981));
#18227=CARTESIAN_POINT('Ctrl Pts',(94.5862550313957,-1.68258466530683,1.42668474142382));
#18228=CARTESIAN_POINT('Ctrl Pts',(94.5808233012484,-1.61996119534367,1.49741437338544));
#18229=CARTESIAN_POINT('Ctrl Pts',(94.5743055809071,-1.53673671437914,1.58005723463099));
#18230=CARTESIAN_POINT('Ctrl Pts',(94.5730438219896,-1.5202334454677,1.59594201688346));
#18231=CARTESIAN_POINT('Ctrl Pts',(94.571032557923,-1.49329885332566,1.62107020312033));
#18232=CARTESIAN_POINT('Ctrl Pts',(94.570276084166,-1.48302256647159,1.63047666301964));
#18233=CARTESIAN_POINT('Ctrl Pts',(94.5688384817129,-1.46321702831027,1.64826361241219));
#18234=CARTESIAN_POINT('Ctrl Pts',(94.5681566772875,-1.45370326649285,1.65666044507058));
#18235=CARTESIAN_POINT('Ctrl Pts',(94.566609550832,-1.43184237692007,1.67562150747281));
#18236=CARTESIAN_POINT('Ctrl Pts',(94.5657464534221,-1.41944979736318,1.68613235557603));
#18237=CARTESIAN_POINT('Ctrl Pts',(94.5634614017015,-1.38612460232055,1.71376952841054));
#18238=CARTESIAN_POINT('Ctrl Pts',(94.5620493238293,-1.36499077232947,1.73064949775185));
#18239=CARTESIAN_POINT('Ctrl Pts',(94.5519606208862,-1.21026655704501,1.84963267221418));
#18240=CARTESIAN_POINT('Ctrl Pts',(94.5439059182204,-1.06569385211044,1.9365401087172));
#18241=CARTESIAN_POINT('Ctrl Pts',(94.5299652239656,-0.803561649952779,
2.05578789240313));
#18242=CARTESIAN_POINT('Ctrl Pts',(94.5241256282431,-0.690634770208763,
2.09642366112328));
#18243=CARTESIAN_POINT('Ctrl Pts',(94.5170090817207,-0.560092942335982,
2.13170113889706));
#18244=CARTESIAN_POINT('Ctrl Pts',(94.5161898261469,-0.545163222984276,
2.13556804700443));
#18245=CARTESIAN_POINT('Ctrl Pts',(94.5149147299864,-0.522107505112866,
2.14128213249482));
#18246=CARTESIAN_POINT('Ctrl Pts',(94.5144649796325,-0.514009270853523,
2.14324050976239));
#18247=CARTESIAN_POINT('Ctrl Pts',(94.5136266490381,-0.498982642042792,
2.14678430167562));
#18248=CARTESIAN_POINT('Ctrl Pts',(94.5132387768276,-0.492057460226592,
2.1483821741579));
#18249=CARTESIAN_POINT('Ctrl Pts',(94.5123452575692,-0.476165233616216,
2.15196817572778));
#18250=CARTESIAN_POINT('Ctrl Pts',(94.5118383709981,-0.4671933852342,2.15393377188569));
#18251=CARTESIAN_POINT('Ctrl Pts',(94.5102043896584,-0.438400797491839,
2.16005343885146));
#18252=CARTESIAN_POINT('Ctrl Pts',(94.5090660196636,-0.418535533573185,
2.16399031088738));
#18253=CARTESIAN_POINT('Ctrl Pts',(94.5003582155636,-0.267775662567264,
2.19171423353927));
#18254=CARTESIAN_POINT('Ctrl Pts',(94.4923181198752,-0.135031132672781,
2.20387769499502));
#18255=CARTESIAN_POINT('Ctrl Pts',(94.4842916325511,-0.00134083298710741,
2.20399969411079));
#18256=CARTESIAN_POINT('Ctrl Pts',(94.4842513832266,-0.000670412990111774,
2.20399999999996));
#18257=CARTESIAN_POINT('Ctrl Pts',(94.4842111356677,-1.34689240618509E-10,
2.204));
#18258=CARTESIAN_POINT('',(95.1243292764227,0.000992167725779152,2.20400002542528));
#18259=CARTESIAN_POINT('Ctrl Pts',(94.3756281550323,1.12638885946569E-10,
2.204));
#18260=CARTESIAN_POINT('Ctrl Pts',(94.3756603584168,-0.000665905572939986,
2.20400000000003));
#18261=CARTESIAN_POINT('Ctrl Pts',(94.3756925632963,-0.00133181967448933,
2.20399969821039));
#18262=CARTESIAN_POINT('Ctrl Pts',(94.3814370060071,-0.120107845755977,
2.2038920376001));
#18263=CARTESIAN_POINT('Ctrl Pts',(94.3871674758867,-0.238006547199598,
2.19429103065167));
#18264=CARTESIAN_POINT('Ctrl Pts',(94.3943898537762,-0.374833827996369,
2.17198936119313));
#18265=CARTESIAN_POINT('Ctrl Pts',(94.3954728914742,-0.395065404477184,
2.1684006664732));
#18266=CARTESIAN_POINT('Ctrl Pts',(94.3970750084256,-0.424509131606257,
2.16275218550346));
#18267=CARTESIAN_POINT('Ctrl Pts',(94.3975823208827,-0.43376345833301,2.16091514742445));
#18268=CARTESIAN_POINT('Ctrl Pts',(94.3984825076259,-0.450055370000045,
2.15757223671038));
#18269=CARTESIAN_POINT('Ctrl Pts',(94.3988739814633,-0.457097789643795,
2.15609123235015));
#18270=CARTESIAN_POINT('Ctrl Pts',(94.3997224283165,-0.472267062230176,
2.15282350751547));
#18271=CARTESIAN_POINT('Ctrl Pts',(94.4001800119445,-0.480390961667001,
2.15102527922317));
#18272=CARTESIAN_POINT('Ctrl Pts',(94.4014767735422,-0.503260164331028,
2.14582715759506));
#18273=CARTESIAN_POINT('Ctrl Pts',(94.4023216249636,-0.51798063809598,2.14232140817679));
#18274=CARTESIAN_POINT('Ctrl Pts',(94.408509077786,-0.624604415317,2.11576530881441));
#18275=CARTESIAN_POINT('Ctrl Pts',(94.4141170458627,-0.714964907046716,
2.08696318169097));
#18276=CARTESIAN_POINT('Ctrl Pts',(94.428827143887,-0.943795594881254,1.99741477382729));
#18277=CARTESIAN_POINT('Ctrl Pts',(94.437961870912,-1.07839850063502,1.92807712305759));
#18278=CARTESIAN_POINT('Ctrl Pts',(94.4501225136957,-1.25481204349963,1.81290416886955));
#18279=CARTESIAN_POINT('Ctrl Pts',(94.4535010828379,-1.3034228480651,1.77827574302474));
#18280=CARTESIAN_POINT('Ctrl Pts',(94.4579509887189,-1.36692043279413,1.72903802857983));
#18281=CARTESIAN_POINT('Ctrl Pts',(94.4590876281688,-1.38308986876587,1.71613123916088));
#18282=CARTESIAN_POINT('Ctrl Pts',(94.4609536206613,-1.40954468585156,1.69439763734456));
#18283=CARTESIAN_POINT('Ctrl Pts',(94.4616881254762,-1.41993441027096,1.68570040543558));
#18284=CARTESIAN_POINT('Ctrl Pts',(94.4631214951614,-1.44015962619177,1.66845021270613));
#18285=CARTESIAN_POINT('Ctrl Pts',(94.463820622714,-1.45000074061522,1.6599047332576));
#18286=CARTESIAN_POINT('Ctrl Pts',(94.465480402562,-1.47330248513692,1.63930541420828));
#18287=CARTESIAN_POINT('Ctrl Pts',(94.4664376893326,-1.48669193782314,1.62717225942816));
#18288=CARTESIAN_POINT('Ctrl Pts',(94.4697371336208,-1.53264337467385,1.58449158278119));
#18289=CARTESIAN_POINT('Ctrl Pts',(94.4720440914672,-1.56442629826278,1.5531194417556));
#18290=CARTESIAN_POINT('Ctrl Pts',(94.4776793394126,-1.64085384205909,1.47295124449219));
#18291=CARTESIAN_POINT('Ctrl Pts',(94.4809618613709,-1.68429762687299,1.42307027012563));
#18292=CARTESIAN_POINT('Ctrl Pts',(94.490380402647,-1.80395091522768,1.27251781388112));
#18293=CARTESIAN_POINT('Ctrl Pts',(94.4963708138563,-1.8738342020333,1.16716936691133));
#18294=CARTESIAN_POINT('Ctrl Pts',(94.5062557194725,-1.97007732161288,0.990947608061888));
#18295=CARTESIAN_POINT('Ctrl Pts',(94.5100033845764,-2.00248616266083,0.923703958155115));
#18296=CARTESIAN_POINT('Ctrl Pts',(94.5147125526,-2.03716335532569,0.841308871634398));
#18297=CARTESIAN_POINT('Ctrl Pts',(94.5154994511445,-2.0427681408028,0.827607064443033));
#18298=CARTESIAN_POINT('Ctrl Pts',(94.5167419694619,-2.05131328635725,0.806101312884716));
#18299=CARTESIAN_POINT('Ctrl Pts',(94.5171921723073,-2.05434820126022,0.798335135613543));
#18300=CARTESIAN_POINT('Ctrl Pts',(94.5179965230591,-2.05966021507238,0.784511108820873));
#18301=CARTESIAN_POINT('Ctrl Pts',(94.5183496238474,-2.06195479903506,0.778460201139327));
#18302=CARTESIAN_POINT('Ctrl Pts',(94.5192058439,-2.06742945941987,0.763829273339396));
#18303=CARTESIAN_POINT('Ctrl Pts',(94.5197105122668,-2.07058276322769,0.755239526897));
#18304=CARTESIAN_POINT('Ctrl Pts',(94.5212857947462,-2.08020229020692,0.728522372076816));
#18305=CARTESIAN_POINT('Ctrl Pts',(94.5223663736296,-2.0864844573493,0.710330185616078));
#18306=CARTESIAN_POINT('Ctrl Pts',(94.5279854006355,-2.11759212056749,0.616272217557925));
#18307=CARTESIAN_POINT('Ctrl Pts',(94.5326957119678,-2.13851919186233,0.539185872900125));
#18308=CARTESIAN_POINT('Ctrl Pts',(94.549582625566,-2.19766874144523,0.262741197554854));
#18309=CARTESIAN_POINT('Ctrl Pts',(94.5618807067509,-2.21252895118918,0.059380895671477));
#18310=CARTESIAN_POINT('Ctrl Pts',(94.574745497895,-2.19762135603939,-0.169650800625656));
#18311=CARTESIAN_POINT('Ctrl Pts',(94.5762192447749,-2.19541801600012,-0.196114355639268));
#18312=CARTESIAN_POINT('Ctrl Pts',(94.5785773159967,-2.19108442030512,-0.238815696861388));
#18313=CARTESIAN_POINT('Ctrl Pts',(94.5794707986488,-2.18925054200563,-0.255080298515061));
#18314=CARTESIAN_POINT('Ctrl Pts',(94.5810516645112,-2.18566261717819,-0.284003865194152));
#18315=CARTESIAN_POINT('Ctrl Pts',(94.5817412426445,-2.18397934293876,-0.296670711041313));
#18316=CARTESIAN_POINT('Ctrl Pts',(94.5831922750453,-2.1801866670565,-0.323427015661422));
#18317=CARTESIAN_POINT('Ctrl Pts',(94.5839528532646,-2.17805062024215,-0.33751214255634));
#18318=CARTESIAN_POINT('Ctrl Pts',(94.585980754515,-2.1719575953012,-0.375219716176894));
#18319=CARTESIAN_POINT('Ctrl Pts',(94.5872401782358,-2.16775182265475,-0.398800358343093));
#18320=CARTESIAN_POINT('Ctrl Pts',(94.5943151576711,-2.14173436744721,-0.53206785181755));
#18321=CARTESIAN_POINT('Ctrl Pts',(94.5998711615385,-2.11198292317703,-0.640042334683499));
#18322=CARTESIAN_POINT('Ctrl Pts',(94.6098883553534,-2.04246581987901,-0.833507129531586));
#18323=CARTESIAN_POINT('Ctrl Pts',(94.6143739435136,-2.00517748515058,-0.919599753557666));
#18324=CARTESIAN_POINT('Ctrl Pts',(94.6234759138139,-1.92025371798433,-1.08575672111937));
#18325=CARTESIAN_POINT('Ctrl Pts',(94.6280830984615,-1.87280386056076,-1.16569473670524));
#18326=CARTESIAN_POINT('Ctrl Pts',(94.633770959352,-1.81188572022221,-1.25495717496773));
#18327=CARTESIAN_POINT('Ctrl Pts',(94.6345789534238,-1.80318169629193,-1.26743170184523));
#18328=CARTESIAN_POINT('Ctrl Pts',(94.6358476899361,-1.7894548422516,-1.28667727845705));
#18329=CARTESIAN_POINT('Ctrl Pts',(94.6363026406733,-1.78452094574,-1.29351151552009));
#18330=CARTESIAN_POINT('Ctrl Pts',(94.6371501145204,-1.77531238233518,-1.30611388783453));
#18331=CARTESIAN_POINT('Ctrl Pts',(94.6375419071523,-1.77104859570609,-1.3118896332484));
#18332=CARTESIAN_POINT('Ctrl Pts',(94.6384528752134,-1.76111882308256,-1.32520391726211));
#18333=CARTESIAN_POINT('Ctrl Pts',(94.6389734211871,-1.75543261148422,-1.33272700550586));
#18334=CARTESIAN_POINT('Ctrl Pts',(94.6406496700567,-1.73707649153843,-1.35669160538816));
#18335=CARTESIAN_POINT('Ctrl Pts',(94.6418171791544,-1.72422288166653,-1.37299025494268));
#18336=CARTESIAN_POINT('Ctrl Pts',(94.6483461243012,-1.65184258107557,-1.46215053888393));
#18337=CARTESIAN_POINT('Ctrl Pts',(94.6539413704332,-1.58793173548193,-1.53131904804282));
#18338=CARTESIAN_POINT('Ctrl Pts',(94.669891758723,-1.39528361127149,-1.71474831573362));
#18339=CARTESIAN_POINT('Ctrl Pts',(94.6802492947213,-1.25729596392934,-1.81835139077675));
#18340=CARTESIAN_POINT('Ctrl Pts',(94.6921566030249,-1.07556145416562,-1.92412306623286));
#18341=CARTESIAN_POINT('Ctrl Pts',(94.6942954122609,-1.0419719778218,-1.94251812638679));
#18342=CARTESIAN_POINT('Ctrl Pts',(94.69726157423,-0.994054931522833,-1.96715882033234));
#18343=CARTESIAN_POINT('Ctrl Pts',(94.6981145982998,-0.980115643916835,
-1.97414092037179));
#18344=CARTESIAN_POINT('Ctrl Pts',(94.6996682424122,-0.954438726629095,
-1.98666331762068));
#18345=CARTESIAN_POINT('Ctrl Pts',(94.7003704187746,-0.942724077335754,
-1.99224891631784));
#18346=CARTESIAN_POINT('Ctrl Pts',(94.7017907621722,-0.918807470638382,
-2.00339427104166));
#18347=CARTESIAN_POINT('Ctrl Pts',(94.7025086578334,-0.906602738075145,
-2.0089468035757));
#18348=CARTESIAN_POINT('Ctrl Pts',(94.7042883342142,-0.876062217245818,
-2.02250618483475));
#18349=CARTESIAN_POINT('Ctrl Pts',(94.7053453933834,-0.85766645096825,-2.03037547516879));
#18350=CARTESIAN_POINT('Ctrl Pts',(94.7094966433949,-0.784448118199279,
-2.06052391041379));
#18351=CARTESIAN_POINT('Ctrl Pts',(94.7125252949487,-0.728842879037055,
-2.0808427294667));
#18352=CARTESIAN_POINT('Ctrl Pts',(94.7205977814119,-0.575800747787049,
-2.12987715655826));
#18353=CARTESIAN_POINT('Ctrl Pts',(94.7255183207916,-0.477089153385412,
-2.15413803855601));
#18354=CARTESIAN_POINT('Ctrl Pts',(94.7371276332037,-0.240453739452461,
-2.19522668619101));
#18355=CARTESIAN_POINT('Ctrl Pts',(94.7437755048809,-0.101935440147125,
-2.20600059452965));
#18356=CARTESIAN_POINT('Ctrl Pts',(94.7520424886914,0.0564468562763539,
-2.20336593864636));
#18357=CARTESIAN_POINT('Ctrl Pts',(94.7530872300339,0.0762297046191279,
-2.2027702298515));
#18358=CARTESIAN_POINT('Ctrl Pts',(94.7546408236654,0.105245319595247,-2.20150517594025));
#18359=CARTESIAN_POINT('Ctrl Pts',(94.7551388072197,0.114486684909912,-2.20104393634964));
#18360=CARTESIAN_POINT('Ctrl Pts',(94.7560281385079,0.130878214525047,-2.20012232102227));
#18361=CARTESIAN_POINT('Ctrl Pts',(94.756418195624,0.138029411599341,-2.19968525341839));
#18362=CARTESIAN_POINT('Ctrl Pts',(94.7572784795002,0.153716898625965,-2.19864966208269));
#18363=CARTESIAN_POINT('Ctrl Pts',(94.7577494858428,0.162251769185203,-2.19803630084633));
#18364=CARTESIAN_POINT('Ctrl Pts',(94.7591228985708,0.18699071275373,-2.19611355803785));
#18365=CARTESIAN_POINT('Ctrl Pts',(94.7600320465024,0.203183808262649,-2.19467459882351));
#18366=CARTESIAN_POINT('Ctrl Pts',(94.7680361211263,0.344320810274916,-2.18055746602971));
#18367=CARTESIAN_POINT('Ctrl Pts',(94.7755839175224,0.467975235483891,-2.15740157320715));
#18368=CARTESIAN_POINT('Ctrl Pts',(94.7927226877972,0.742869450418756,-2.08116949469576));
#18369=CARTESIAN_POINT('Ctrl Pts',(94.8022353651095,0.891694734497508,-2.02188449193232));
#18370=CARTESIAN_POINT('Ctrl Pts',(94.8127596822778,1.05730873895497,-1.93403275758604));
#18371=CARTESIAN_POINT('Ctrl Pts',(94.8143001093834,1.0815514271325,-1.92058092409919));
#18372=CARTESIAN_POINT('Ctrl Pts',(94.8167328458202,1.11982979408872,-1.89838623141298));
#18373=CARTESIAN_POINT('Ctrl Pts',(94.8176355316651,1.13403149155927,-1.88993694299338));
#18374=CARTESIAN_POINT('Ctrl Pts',(94.8192289007036,1.15909106293141,-1.87464358907408));
#18375=CARTESIAN_POINT('Ctrl Pts',(94.8199218584762,1.16998658611627,-1.86786297041886));
#18376=CARTESIAN_POINT('Ctrl Pts',(94.8213645344086,1.19266006286278,-1.85347633414525));
#18377=CARTESIAN_POINT('Ctrl Pts',(94.8221135428954,1.20442593935234,-1.84585230065864));
#18378=CARTESIAN_POINT('Ctrl Pts',(94.8240750096577,1.23521472665582,-1.82548209306741));
#18379=CARTESIAN_POINT('Ctrl Pts',(94.8252804762971,1.25411339267919,-1.81255067331888));
#18380=CARTESIAN_POINT('Ctrl Pts',(94.8312768231741,1.34792013137746,-1.74619367133545));
#18381=CARTESIAN_POINT('Ctrl Pts',(94.8358975204975,1.41963583984997,-1.68840679977406));
#18382=CARTESIAN_POINT('Ctrl Pts',(94.8449594687033,1.55566243577444,-1.56398682131651));
#18383=CARTESIAN_POINT('Ctrl Pts',(94.849391527499,1.61980780340455,-1.49745230921312));
#18384=CARTESIAN_POINT('Ctrl Pts',(94.8553970476742,1.70008183819309,-1.40297512291247));
#18385=CARTESIAN_POINT('Ctrl Pts',(94.8569345307262,1.72005043297731,-1.37842080248154));
#18386=CARTESIAN_POINT('Ctrl Pts',(94.8626328911062,1.79152490284368,-1.28655995975371));
#18387=CARTESIAN_POINT('Ctrl Pts',(94.8668603793646,1.83966084014513,-1.21673466517276));
#18388=CARTESIAN_POINT('Ctrl Pts',(94.8721130381572,1.89145695877538,-1.13147359432857));
#18389=CARTESIAN_POINT('Ctrl Pts',(94.8729116922183,1.89912908514909,-1.11854844101027));
#18390=CARTESIAN_POINT('Ctrl Pts',(94.8741688237443,1.91087619665093,-1.09828891294088));
#18391=CARTESIAN_POINT('Ctrl Pts',(94.874621676791,1.91504265173824,-1.09100779672539));
#18392=CARTESIAN_POINT('Ctrl Pts',(94.8754636883955,1.92266671725094,-1.07750607613209));
#18393=CARTESIAN_POINT('Ctrl Pts',(94.8758521074995,1.92613588463787,-1.07129230323676));
#18394=CARTESIAN_POINT('Ctrl Pts',(94.8767607524788,1.9341413693502,-1.05678874928612));
#18395=CARTESIAN_POINT('Ctrl Pts',(94.8772823973392,1.93865451761071,-1.048486505341));
#18396=CARTESIAN_POINT('Ctrl Pts',(94.8789657872865,1.95296068367755,-1.0217611664808));
#18397=CARTESIAN_POINT('Ctrl Pts',(94.8801394747046,1.96254526295985,-1.00322845825735));
#18398=CARTESIAN_POINT('Ctrl Pts',(94.8867372012658,2.01437870852171,-0.899417392524892));
#18399=CARTESIAN_POINT('Ctrl Pts',(94.8924000728882,2.05132959551711,-0.811613930327904));
#18400=CARTESIAN_POINT('Ctrl Pts',(94.9086214533789,2.13989618315697,-0.556054388239939));
#18401=CARTESIAN_POINT('Ctrl Pts',(94.9191735626596,2.1773438098686,-0.384115138328087));
#18402=CARTESIAN_POINT('Ctrl Pts',(94.9310850295551,2.19740697483563,-0.174040956457307));
#18403=CARTESIAN_POINT('Ctrl Pts',(94.9330720868704,2.19993538459887,-0.138463643182172));
#18404=CARTESIAN_POINT('Ctrl Pts',(94.9359337918393,2.20236468671953,-0.0864566731110639));
#18405=CARTESIAN_POINT('Ctrl Pts',(94.9368295051764,2.20294706206198,-0.0700659111716392));
#18406=CARTESIAN_POINT('Ctrl Pts',(94.9384149387745,2.2036585173826,-0.0408580337970744));
#18407=CARTESIAN_POINT('Ctrl Pts',(94.9391068563871,2.20385884509099,-0.0280435511618437));
#18408=CARTESIAN_POINT('Ctrl Pts',(94.9405517048102,2.20404468462632,-0.00114675610603145));
#18409=CARTESIAN_POINT('Ctrl Pts',(94.9413038794707,2.20400702831426,0.0129351701960996));
#18410=CARTESIAN_POINT('Ctrl Pts',(94.9432835338189,2.20355021233875,0.0502000084250539));
#18411=CARTESIAN_POINT('Ctrl Pts',(94.9445037777823,2.20290018123056,0.073378638528881));
#18412=CARTESIAN_POINT('Ctrl Pts',(94.9507571325891,2.19764897460059,0.193144077679191));
#18413=CARTESIAN_POINT('Ctrl Pts',(94.9556007948011,2.18706093207713,0.289366295581169));
#18414=CARTESIAN_POINT('Ctrl Pts',(94.9670460678092,2.14633691738416,0.519165870379614));
#18415=CARTESIAN_POINT('Ctrl Pts',(94.9735132740383,2.11002345446319,0.65122495560932));
#18416=CARTESIAN_POINT('Ctrl Pts',(94.9836285781819,2.0377162494379,0.842578368128476));
#18417=CARTESIAN_POINT('Ctrl Pts',(94.9870562378527,2.01079654792246,0.904942821402023));
#18418=CARTESIAN_POINT('Ctrl Pts',(94.9913968969472,1.97471083384666,0.97894941946147));
#18419=CARTESIAN_POINT('Ctrl Pts',(94.9921655217908,1.96824969470334,0.991875980380583));
#18420=CARTESIAN_POINT('Ctrl Pts',(94.9933853103976,1.95789713922495,1.01208843483221));
#18421=CARTESIAN_POINT('Ctrl Pts',(94.9938313730318,1.95409097653468,1.01941780375403));
#18422=CARTESIAN_POINT('Ctrl Pts',(94.9946717075392,1.94688539499829,1.03310465649419));
#18423=CARTESIAN_POINT('Ctrl Pts',(94.9950653732984,1.94349587326475,1.03946705473974));
#18424=CARTESIAN_POINT('Ctrl Pts',(94.9959935239273,1.93547084701258,1.05435419036693));
#18425=CARTESIAN_POINT('Ctrl Pts',(94.9965295595233,1.93081018984679,1.06286507230188));
#18426=CARTESIAN_POINT('Ctrl Pts',(94.9983084208148,1.91525232064573,1.09083544535661));
#18427=CARTESIAN_POINT('Ctrl Pts',(94.9995650842185,1.90411625989537,1.11015972330232));
#18428=CARTESIAN_POINT('Ctrl Pts',(95.0026553827308,1.87632760367246,1.15673263157023));
#18429=CARTESIAN_POINT('Ctrl Pts',(95.0045034541841,1.859372564361,1.18379438500978));
#18430=CARTESIAN_POINT('Ctrl Pts',(95.0122371096884,1.78677878771326,1.29425155196647));
#18431=CARTESIAN_POINT('Ctrl Pts',(95.0182866652785,1.72607166508914,1.37416913101112));
#18432=CARTESIAN_POINT('Ctrl Pts',(95.0328681820659,1.5662869875503,1.5571514175172));
#18433=CARTESIAN_POINT('Ctrl Pts',(95.0413139952279,1.46220806014156,1.65527456326024));
#18434=CARTESIAN_POINT('Ctrl Pts',(95.051075126406,1.32482885774414,1.76164893967077));
#18435=CARTESIAN_POINT('Ctrl Pts',(95.0527982697611,1.29989972305135,1.78012340508014));
#18436=CARTESIAN_POINT('Ctrl Pts',(95.0553742590352,1.26160864439989,1.80726664890969));
#18437=CARTESIAN_POINT('Ctrl Pts',(95.0562420197389,1.24852990153853,1.81632657183962));
#18438=CARTESIAN_POINT('Ctrl Pts',(95.057794578453,1.22480897708247,1.8323812657761));
#18439=CARTESIAN_POINT('Ctrl Pts',(95.0584812823748,1.21420219599957,1.83942685916755));
#18440=CARTESIAN_POINT('Ctrl Pts',(95.0599442115389,1.19136254978204,1.85431453413357));
#18441=CARTESIAN_POINT('Ctrl Pts',(95.0607193619697,1.17911195102925,1.86212838904119));
#18442=CARTESIAN_POINT('Ctrl Pts',(95.0628311415837,1.1453365721306,1.88320452680582));
#18443=CARTESIAN_POINT('Ctrl Pts',(95.0641586604965,1.12365913181226,1.89621870522438));
#18444=CARTESIAN_POINT('Ctrl Pts',(95.0732955525266,0.971499688881277,1.9840427023134));
#18445=CARTESIAN_POINT('Ctrl Pts',(95.0806084984028,0.833881793724874,2.04569894083342));
#18446=CARTESIAN_POINT('Ctrl Pts',(95.0919755234633,0.610576225909772,2.11943240375127));
#18447=CARTESIAN_POINT('Ctrl Pts',(95.0960573438333,0.528645867197792,2.1413382577356));
#18448=CARTESIAN_POINT('Ctrl Pts',(95.103286690977,0.386007031158793,2.1707890096286));
#18449=CARTESIAN_POINT('Ctrl Pts',(95.1063719261145,0.325872097147621,2.18062664968732));
#18450=CARTESIAN_POINT('Ctrl Pts',(95.1103772907329,0.25032707108405,2.18979068910146));
#18451=CARTESIAN_POINT('Ctrl Pts',(95.1111844849624,0.235224001110319,2.19146447575686));
#18452=CARTESIAN_POINT('Ctrl Pts',(95.1124522278693,0.211721613711599,2.19382336383564));
#18453=CARTESIAN_POINT('Ctrl Pts',(95.1129069992533,0.203333360523734,2.19461671668196));
#18454=CARTESIAN_POINT('Ctrl Pts',(95.1137506618996,0.187856377468746,2.19599102178044));
#18455=CARTESIAN_POINT('Ctrl Pts',(95.1141387878109,0.180769143098662,2.19658578222223));
#18456=CARTESIAN_POINT('Ctrl Pts',(95.1149152780157,0.166654566063787,2.19770150590659));
#18457=CARTESIAN_POINT('Ctrl Pts',(95.1153035821304,0.159627434170662,2.19822308533632));
#18458=CARTESIAN_POINT('Ctrl Pts',(95.1162074481433,0.143338726683818,2.19935357706634));
#18459=CARTESIAN_POINT('Ctrl Pts',(95.1167242955759,0.134075626027717,2.19993769638116));
#18460=CARTESIAN_POINT('Ctrl Pts',(95.1195564510705,0.0835752989115121,
2.20280205199079));
#18461=CARTESIAN_POINT('Ctrl Pts',(95.1219242869929,0.0422862894867362,
2.20398120245318));
#18462=CARTESIAN_POINT('Ctrl Pts',(95.1243288921836,0.000991366063952221,
2.20399977704022));
#18463=CARTESIAN_POINT('Ctrl Pts',(95.1243288469655,0.000992142605052562,
2.20399977669079));
#18464=CARTESIAN_POINT('Ctrl Pts',(95.1243481046162,0.000661425794219861,
2.20399992556478));
#18465=CARTESIAN_POINT('Ctrl Pts',(95.1243673644587,0.000330711594234764,
2.204));
#18466=CARTESIAN_POINT('Ctrl Pts',(95.1243866264839,2.95873024051195E-11,
2.204));
#18467=CARTESIAN_POINT('Origin',(66.9212607628943,0.,0.));
#18468=CARTESIAN_POINT('',(95.9829026914895,-1.13898760397551E-11,2.204));
#18469=CARTESIAN_POINT('',(95.8777130322977,9.44243789243157E-12,2.204));
#18470=CARTESIAN_POINT('',(66.9212607628943,-2.69912154532077E-16,2.204));
#18471=CARTESIAN_POINT('Ctrl Pts',(95.9829026914895,-1.13898760397551E-11,
2.204));
#18472=CARTESIAN_POINT('Ctrl Pts',(95.9828788298517,0.000477678869200619,
2.204));
#18473=CARTESIAN_POINT('Ctrl Pts',(95.9828549715523,0.000955359704270702,
2.20399984473618));
#18474=CARTESIAN_POINT('Ctrl Pts',(95.9772330995163,0.113530410574079,2.20392664806559));
#18475=CARTESIAN_POINT('Ctrl Pts',(95.971843390864,0.225462406806485,2.19530176314732));
#18476=CARTESIAN_POINT('Ctrl Pts',(95.960748388197,0.452160190387588,2.16030593424989));
#18477=CARTESIAN_POINT('Ctrl Pts',(95.9550547837466,0.566442579419279,2.13319190341888));
#18478=CARTESIAN_POINT('Ctrl Pts',(95.9479704766969,0.695808852201622,2.09136698605005));
#18479=CARTESIAN_POINT('Ctrl Pts',(95.9469854486833,0.713531039618399,2.08538707198984));
#18480=CARTESIAN_POINT('Ctrl Pts',(95.9454995899027,0.739819876967249,2.07614222474404));
#18481=CARTESIAN_POINT('Ctrl Pts',(95.9450080326983,0.748446153979837,2.07304807864895));
#18482=CARTESIAN_POINT('Ctrl Pts',(95.9441552683583,0.763283024209296,2.06762158867299));
#18483=CARTESIAN_POINT('Ctrl Pts',(95.9437955483123,0.769502913561527,2.06531481198765));
#18484=CARTESIAN_POINT('Ctrl Pts',(95.9430286584377,0.782678114204441,2.06036073396123));
#18485=CARTESIAN_POINT('Ctrl Pts',(95.9426210487632,0.789630580475892,2.05770622947755));
#18486=CARTESIAN_POINT('Ctrl Pts',(95.9415882394253,0.807124976781946,2.05092501920776));
#18487=CARTESIAN_POINT('Ctrl Pts',(95.940960382653,0.817648699440852,2.04675224577705));
#18488=CARTESIAN_POINT('Ctrl Pts',(95.9384350863003,0.859557583582711,2.02976011459988));
#18489=CARTESIAN_POINT('Ctrl Pts',(95.9365038151161,0.89067581866469,2.01629900957249));
#18490=CARTESIAN_POINT('Ctrl Pts',(95.9312016022936,0.974021133981133,1.97793971267486));
#18491=CARTESIAN_POINT('Ctrl Pts',(95.9277799541229,1.02559749774177,1.95169457898942));
#18492=CARTESIAN_POINT('Ctrl Pts',(95.9160056719715,1.19772130709342,1.85539963625697));
#18493=CARTESIAN_POINT('Ctrl Pts',(95.9075499420374,1.31264472648618,1.7759541265129));
#18494=CARTESIAN_POINT('Ctrl Pts',(95.8948546686544,1.47884266353129,1.63606184903826));
#18495=CARTESIAN_POINT('Ctrl Pts',(95.8904052116827,1.53569690762821,1.58281744223646));
#18496=CARTESIAN_POINT('Ctrl Pts',(95.884836772622,1.60515496398002,1.51049546387426));
#18497=CARTESIAN_POINT('Ctrl Pts',(95.8836019046699,1.62044284947127,1.49408300602855));
#18498=CARTESIAN_POINT('Ctrl Pts',(95.8816229298707,1.64474782850392,1.46717817867799));
#18499=CARTESIAN_POINT('Ctrl Pts',(95.8808722494358,1.65392105181594,1.45682956929318));
#18500=CARTESIAN_POINT('Ctrl Pts',(95.8794389704193,1.67134302971768,1.43679860675478));
#18501=CARTESIAN_POINT('Ctrl Pts',(95.8787557726136,1.67960653277266,1.42712986929033));
#18502=CARTESIAN_POINT('Ctrl Pts',(95.8771811372737,1.69855321179957,1.40456872547964));
#18503=CARTESIAN_POINT('Ctrl Pts',(95.8762922557781,1.70917416944192,1.3916249485023));
#18504=CARTESIAN_POINT('Ctrl Pts',(95.8734499402949,1.74288091317044,1.34957843215756));
#18505=CARTESIAN_POINT('Ctrl Pts',(95.8715197610336,1.76537940108509,1.32001197042428));
#18506=CARTESIAN_POINT('Ctrl Pts',(95.8637313666677,1.85428498454624,1.19683477041537));
#18507=CARTESIAN_POINT('Ctrl Pts',(95.8581153579943,1.91408239820586,1.0986709879389));
#18508=CARTESIAN_POINT('Ctrl Pts',(95.8457792044542,2.02924036487385,0.871431735969079));
#18509=CARTESIAN_POINT('Ctrl Pts',(95.8391169559389,2.0804708370472,0.740839780797122));
#18510=CARTESIAN_POINT('Ctrl Pts',(95.8303830579762,2.12728246153167,0.577233542046017));
#18511=CARTESIAN_POINT('Ctrl Pts',(95.8288080015182,2.13499663890228,0.548013147820725));
#18512=CARTESIAN_POINT('Ctrl Pts',(95.8266075336666,2.14473689035551,0.507783955018259));
#18513=CARTESIAN_POINT('Ctrl Pts',(95.8260092080454,2.14728382352938,0.496903455824378));
#18514=CARTESIAN_POINT('Ctrl Pts',(95.8250460247891,2.15121999231037,0.479492559427847));
#18515=CARTESIAN_POINT('Ctrl Pts',(95.8246841458569,2.15266251801091,0.472974260372433));
#18516=CARTESIAN_POINT('Ctrl Pts',(95.8239179273568,2.15563984879748,0.459224875658199));
#18517=CARTESIAN_POINT('Ctrl Pts',(95.8235131946761,2.157167919286,0.451992486138058));
#18518=CARTESIAN_POINT('Ctrl Pts',(95.822496695825,2.16089569634518,0.433899281488422));
#18519=CARTESIAN_POINT('Ctrl Pts',(95.8218824355277,2.16304991204809,0.42302938946607));
#18520=CARTESIAN_POINT('Ctrl Pts',(95.8194794057673,2.17110202893434,0.380729082836426));
#18521=CARTESIAN_POINT('Ctrl Pts',(95.8176606780988,2.17639730140451,0.349189384573342));
#18522=CARTESIAN_POINT('Ctrl Pts',(95.8127577551507,2.18864603562437,0.265061653354419));
#18523=CARTESIAN_POINT('Ctrl Pts',(95.8096309306682,2.19439031154624,0.212319829583095));
#18524=CARTESIAN_POINT('Ctrl Pts',(95.7971070184038,2.20960255166768,0.00256671632292191));
#18525=CARTESIAN_POINT('Ctrl Pts',(95.7875393528914,2.20415722066994,-0.15507799154341));
#18526=CARTESIAN_POINT('Ctrl Pts',(95.7743943310034,2.17225322307569,-0.379058427748882));
#18527=CARTESIAN_POINT('Ctrl Pts',(95.7704708080942,2.15933286616092,-0.446824770169614));
#18528=CARTESIAN_POINT('Ctrl Pts',(95.7654504441312,2.13822707356381,-0.534851470617449));
#18529=CARTESIAN_POINT('Ctrl Pts',(95.7642641741997,2.13289100953263,-0.55574913577905));
#18530=CARTESIAN_POINT('Ctrl Pts',(95.7623435676437,2.123679689425,-0.589734460311962));
#18531=CARTESIAN_POINT('Ctrl Pts',(95.7616033493435,2.11998818038015,-0.602870038866647));
#18532=CARTESIAN_POINT('Ctrl Pts',(95.760177175874,2.11260163575163,-0.628246603148619));
#18533=CARTESIAN_POINT('Ctrl Pts',(95.7594907658293,2.10892159730474,-0.640491351779439));
#18534=CARTESIAN_POINT('Ctrl Pts',(95.7578895911733,2.1000444964434,-0.66912226191492));
#18535=CARTESIAN_POINT('Ctrl Pts',(95.756977668929,2.09476182874159,-0.685481138923474));
#18536=CARTESIAN_POINT('Ctrl Pts',(95.7539758941104,2.07662344326546,-0.739481658425887));
#18537=CARTESIAN_POINT('Ctrl Pts',(95.7519132345112,2.06293987069779,-0.776838073883258));
#18538=CARTESIAN_POINT('Ctrl Pts',(95.741922073855,1.99078526391338,-0.958442731523179));
#18539=CARTESIAN_POINT('Ctrl Pts',(95.734474716815,1.91816123209685,-1.0965852934875));
#18540=CARTESIAN_POINT('Ctrl Pts',(95.7261011386309,1.82198430786955,-1.24027704862635));
#18541=CARTESIAN_POINT('Ctrl Pts',(95.7252638884385,1.81221452863861,-1.25450885662443));
#18542=CARTESIAN_POINT('Ctrl Pts',(95.719542317405,1.74451276575315,-1.35068976370314));
#18543=CARTESIAN_POINT('Ctrl Pts',(95.7145881457256,1.68121490013588,-1.42870565251597));
#18544=CARTESIAN_POINT('Ctrl Pts',(95.7085086333395,1.60249588267664,-1.5132259905181));
#18545=CARTESIAN_POINT('Ctrl Pts',(95.707703080167,1.59204681767393,-1.52421548918479));
#18546=CARTESIAN_POINT('Ctrl Pts',(95.7064400485751,1.57565635863231,-1.54110125604584));
#18547=CARTESIAN_POINT('Ctrl Pts',(95.7059883475131,1.56979318012819,-1.54707317500567));
#18548=CARTESIAN_POINT('Ctrl Pts',(95.7051483621836,1.55889164258052,-1.55805111944311));
#18549=CARTESIAN_POINT('Ctrl Pts',(95.7047608123871,1.55386293597412,-1.56306635043527));
#18550=CARTESIAN_POINT('Ctrl Pts',(95.7038620788419,1.54220287107331,-1.57458329405822));
#18551=CARTESIAN_POINT('Ctrl Pts',(95.7033495828948,1.53555459518991,-1.58106746354528));
#18552=CARTESIAN_POINT('Ctrl Pts',(95.7017088200238,1.51426471523994,-1.60157088131654));
#18553=CARTESIAN_POINT('Ctrl Pts',(95.7005693169641,1.49947098748378,-1.61542985417944));
#18554=CARTESIAN_POINT('Ctrl Pts',(95.6943003445732,1.41790414396953,-1.68975701573796));
#18555=CARTESIAN_POINT('Ctrl Pts',(95.6889548297688,1.34766744132494,-1.74628769886602));
#18556=CARTESIAN_POINT('Ctrl Pts',(95.6739828307553,1.14375280433932,-1.89076571931951));
#18557=CARTESIAN_POINT('Ctrl Pts',(95.6643276363342,1.00364508545977,-1.96872390992964));
#18558=CARTESIAN_POINT('Ctrl Pts',(95.6522988591321,0.810118905627756,-2.05032635989805));
#18559=CARTESIAN_POINT('Ctrl Pts',(95.6494747267164,0.763256919178165,-2.06822877608177));
#18560=CARTESIAN_POINT('Ctrl Pts',(95.6456357597286,0.69755139693683,-2.09079201087649));
#18561=CARTESIAN_POINT('Ctrl Pts',(95.6445761751776,0.679198588308657,-2.09682581425617));
#18562=CARTESIAN_POINT('Ctrl Pts',(95.6428789795635,0.649455411325713,-2.106172901717));
#18563=CARTESIAN_POINT('Ctrl Pts',(95.6422364539973,0.638113766044681,-2.10963680583228));
#18564=CARTESIAN_POINT('Ctrl Pts',(95.6409025675322,0.614400945242074,-2.11667032108227));
#18565=CARTESIAN_POINT('Ctrl Pts',(95.6402117675341,0.602025311799606,-2.12022340882817));
#18566=CARTESIAN_POINT('Ctrl Pts',(95.6385780055691,0.572535139050384,-2.12841111472538));
#18567=CARTESIAN_POINT('Ctrl Pts',(95.6376382380577,0.555394275571141,-2.13294809643092));
#18568=CARTESIAN_POINT('Ctrl Pts',(95.6344342076581,0.496367943449949,-2.14781185551503));
#18569=CARTESIAN_POINT('Ctrl Pts',(95.6322026140006,0.454233855180053,-2.15711585862535));
#18570=CARTESIAN_POINT('Ctrl Pts',(95.6267873507527,0.349832029120907,-2.1769747788754));
#18571=CARTESIAN_POINT('Ctrl Pts',(95.623644859853,0.287331454366506,-2.18610223600651));
#18572=CARTESIAN_POINT('Ctrl Pts',(95.6161054336892,0.134532717289035,-2.20174930547751));
#18573=CARTESIAN_POINT('Ctrl Pts',(95.6117634442917,0.044059877445082,-2.20541562124689));
#18574=CARTESIAN_POINT('Ctrl Pts',(95.6058453996764,-0.0780494992300799,
-2.20284533234442));
#18575=CARTESIAN_POINT('Ctrl Pts',(95.6043058133446,-0.109698663752618,
-2.20149618041527));
#18576=CARTESIAN_POINT('Ctrl Pts',(95.5986592491845,-0.2247192225508,-2.19410654689001));
#18577=CARTESIAN_POINT('Ctrl Pts',(95.5944858612555,-0.307751210250835,
-2.1840075083954));
#18578=CARTESIAN_POINT('Ctrl Pts',(95.5892997238766,-0.404670569433291,
-2.16658253927671));
#18579=CARTESIAN_POINT('Ctrl Pts',(95.5885075836227,-0.41931317222477,-2.1637963418094));
#18580=CARTESIAN_POINT('Ctrl Pts',(95.5872612140708,-0.442074753300329,
-2.15922555388672));
#18581=CARTESIAN_POINT('Ctrl Pts',(95.5868125230817,-0.450214061229815,
-2.15754313387671));
#18582=CARTESIAN_POINT('Ctrl Pts',(95.5859787511895,-0.465232241058508,
-2.15435014827385));
#18583=CARTESIAN_POINT('Ctrl Pts',(95.585594400985,-0.472113615061271,-2.1528526028219));
#18584=CARTESIAN_POINT('Ctrl Pts',(95.5846964019476,-0.488096102725699,
-2.14929413314906));
#18585=CARTESIAN_POINT('Ctrl Pts',(95.5841813767188,-0.497191399158086,
-2.14720836958512));
#18586=CARTESIAN_POINT('Ctrl Pts',(95.5825242800639,-0.526240568349298,
-2.14035225542374));
#18587=CARTESIAN_POINT('Ctrl Pts',(95.5813706672503,-0.546140636243568,
-2.13536115372221));
#18588=CARTESIAN_POINT('Ctrl Pts',(95.5749483671129,-0.655360317659839,
-2.10634140111173));
#18589=CARTESIAN_POINT('Ctrl Pts',(95.5694527341025,-0.743162466192057,
-2.07698771908025));
#18590=CARTESIAN_POINT('Ctrl Pts',(95.5539061634405,-0.983485103588377,
-1.97945012509756));
#18591=CARTESIAN_POINT('Ctrl Pts',(95.5438407265759,-1.13051297393192,-1.89932112531321));
#18592=CARTESIAN_POINT('Ctrl Pts',(95.5318979071458,-1.30224624603176,-1.77865576549699));
#18593=CARTESIAN_POINT('Ctrl Pts',(95.5294896912767,-1.33666937037276,-1.75293381917311));
#18594=CARTESIAN_POINT('Ctrl Pts',(95.5261169977226,-1.38456807387419,-1.71491054161252));
#18595=CARTESIAN_POINT('Ctrl Pts',(95.5251208107109,-1.39867547277355,-1.70342415939696));
#18596=CARTESIAN_POINT('Ctrl Pts',(95.5234341090007,-1.42248660896125,-1.68354163184494));
#18597=CARTESIAN_POINT('Ctrl Pts',(95.5227400899828,-1.43226202674004,-1.67523314059028));
#18598=CARTESIAN_POINT('Ctrl Pts',(95.5213337894339,-1.45202172090621,-1.65813924831427));
#18599=CARTESIAN_POINT('Ctrl Pts',(95.5206217978757,-1.46200014760925,-1.64934787835859));
#18600=CARTESIAN_POINT('Ctrl Pts',(95.5188523860982,-1.48672819769768,-1.62716078778031));
#18601=CARTESIAN_POINT('Ctrl Pts',(95.5177996781805,-1.50137704831877,-1.61365422460098));
#18602=CARTESIAN_POINT('Ctrl Pts',(95.5136359095201,-1.55902772957845,-1.55903424355645));
#18603=CARTESIAN_POINT('Ctrl Pts',(95.5105912748449,-1.60054204983427,-1.5163842403494));
#18604=CARTESIAN_POINT('Ctrl Pts',(95.5024446440686,-1.70888344084178,-1.39566555941648));
#18605=CARTESIAN_POINT('Ctrl Pts',(95.4974696147281,-1.7720602108341,-1.31452240006163));
#18606=CARTESIAN_POINT('Ctrl Pts',(95.4858758005733,-1.90584587988259,-1.11542754964171));
#18607=CARTESIAN_POINT('Ctrl Pts',(95.4792935692208,-1.97154078234737,-0.994708786994209));
#18608=CARTESIAN_POINT('Ctrl Pts',(95.4711020069243,-2.03340958794017,-0.850444247370904));
#18609=CARTESIAN_POINT('Ctrl Pts',(95.4700543057658,-2.04098571409772,-0.832098089668565));
#18610=CARTESIAN_POINT('Ctrl Pts',(95.468505241796,-2.05167649511576,-0.805184811190546));
#18611=CARTESIAN_POINT('Ctrl Pts',(95.4680149187935,-2.05498761992263,-0.796696238730226));
#18612=CARTESIAN_POINT('Ctrl Pts',(95.4671369146973,-2.06078521058513,-0.781556608820664));
#18613=CARTESIAN_POINT('Ctrl Pts',(95.4667504611938,-2.06329230078625,-0.774913735121403));
#18614=CARTESIAN_POINT('Ctrl Pts',(95.4659034086266,-2.06868979847421,-0.760400427952536));
#18615=CARTESIAN_POINT('Ctrl Pts',(95.4654421050132,-2.07156737125649,-0.752525690405685));
#18616=CARTESIAN_POINT('Ctrl Pts',(95.4641113287956,-2.07969458913825,-0.729884929413623));
#18617=CARTESIAN_POINT('Ctrl Pts',(95.4632356507201,-2.08483166237382,-0.71507936986997));
#18618=CARTESIAN_POINT('Ctrl Pts',(95.4612172302294,-2.09620773832884,-0.681127446893309));
#18619=CARTESIAN_POINT('Ctrl Pts',(95.4600695911161,-2.10234304626968,-0.661947992250309));
#18620=CARTESIAN_POINT('Ctrl Pts',(95.4561945063687,-2.12199067125946,-0.597497714309787));
#18621=CARTESIAN_POINT('Ctrl Pts',(95.4534214199588,-2.13430960194535,-0.551878597772534));
#18622=CARTESIAN_POINT('Ctrl Pts',(95.4448960935618,-2.1672901412406,-0.41203262207989));
#18623=CARTESIAN_POINT('Ctrl Pts',(95.439062859636,-2.18324229816694,-0.316812846154468));
#18624=CARTESIAN_POINT('Ctrl Pts',(95.4253507254016,-2.2062190450609,-0.0886728181536196));
#18625=CARTESIAN_POINT('Ctrl Pts',(95.4175717140012,-2.20755480215899,0.0444581155629141));
#18626=CARTESIAN_POINT('Ctrl Pts',(95.4088141015528,-2.19493515189288,0.201165496283699));
#18627=CARTESIAN_POINT('Ctrl Pts',(95.407471282794,-2.19258085752587,0.225382182350168));
#18628=CARTESIAN_POINT('Ctrl Pts',(95.4053551211063,-2.18819855392625,0.263836463201095));
#18629=CARTESIAN_POINT('Ctrl Pts',(95.4045736602767,-2.18643140608747,0.278101260277108));
#18630=CARTESIAN_POINT('Ctrl Pts',(95.4031215665938,-2.18286858927177,0.304723853630748));
#18631=CARTESIAN_POINT('Ctrl Pts',(95.4024498823252,-2.18110720594006,0.317085587986598));
#18632=CARTESIAN_POINT('Ctrl Pts',(95.4009410074096,-2.17689393128738,0.344957027060245));
#18633=CARTESIAN_POINT('Ctrl Pts',(95.4001057778675,-2.17438114415292,0.36045692648497));
#18634=CARTESIAN_POINT('Ctrl Pts',(95.397611240752,-2.16633291634213,0.406950713635804));
#18635=CARTESIAN_POINT('Ctrl Pts',(95.3959677169264,-2.16029870135175,0.437854815330427));
#18636=CARTESIAN_POINT('Ctrl Pts',(95.3922146820598,-2.14483321671233,0.508928449400112));
#18637=CARTESIAN_POINT('Ctrl Pts',(95.390119623358,-2.13493198887868,0.548983921417049));
#18638=CARTESIAN_POINT('Ctrl Pts',(95.3825820270884,-2.09477434920969,0.693854952460232));
#18639=CARTESIAN_POINT('Ctrl Pts',(95.3773179076906,-2.05787242978463,0.796666114248553));
#18640=CARTESIAN_POINT('Ctrl Pts',(95.3658907633888,-1.96172497225474,1.01265245630798));
#18641=CARTESIAN_POINT('Ctrl Pts',(95.3597452632532,-1.89996253176276,1.12426208386168));
#18642=CARTESIAN_POINT('Ctrl Pts',(95.3520460566563,-1.81755857001209,1.24680049822258));
#18643=CARTESIAN_POINT('Ctrl Pts',(95.350971943148,-1.80596232214276,1.26353894696805));
#18644=CARTESIAN_POINT('Ctrl Pts',(95.3493909418991,-1.78878998135921,1.28760674525041));
#18645=CARTESIAN_POINT('Ctrl Pts',(95.348895746397,-1.78339693051318,1.29506606393181));
#18646=CARTESIAN_POINT('Ctrl Pts',(95.3480124187299,-1.77375603906876,1.30822630161916));
#18647=CARTESIAN_POINT('Ctrl Pts',(95.3476255735493,-1.7695271201249,1.31394075670797));
#18648=CARTESIAN_POINT('Ctrl Pts',(95.3467818448893,-1.76029024742898,1.32629688646903));
#18649=CARTESIAN_POINT('Ctrl Pts',(95.3463243037234,-1.75527239636436,1.33293060440226));
#18650=CARTESIAN_POINT('Ctrl Pts',(95.3450149921736,-1.74088392023998,1.3517303716658));
#18651=CARTESIAN_POINT('Ctrl Pts',(95.344157312315,-1.73142370736625,1.36382687317468));
#18652=CARTESIAN_POINT('Ctrl Pts',(95.3369273091094,-1.65131025305964,1.46408859531355));
#18653=CARTESIAN_POINT('Ctrl Pts',(95.3301804322812,-1.57410595504838,1.54679239377701));
#18654=CARTESIAN_POINT('Ctrl Pts',(95.3127948679752,-1.3608553742288,1.74266270100023));
#18655=CARTESIAN_POINT('Ctrl Pts',(95.302217609042,-1.21688933528131,1.8460772132719));
#18656=CARTESIAN_POINT('Ctrl Pts',(95.2908520154223,-1.0391345974718,1.94383706267887));
#18657=CARTESIAN_POINT('Ctrl Pts',(95.2893974875975,-1.01593989504199,1.95605967473525));
#18658=CARTESIAN_POINT('Ctrl Pts',(95.2870684537167,-0.978080847492173,
1.97515463042978));
#18659=CARTESIAN_POINT('Ctrl Pts',(95.2861850352415,-0.963549666854866,
1.9822840405858));
#18660=CARTESIAN_POINT('Ctrl Pts',(95.2846212311532,-0.937525699437962,
1.99469835439482));
#18661=CARTESIAN_POINT('Ctrl Pts',(95.283938705088,-0.926063585665992,2.00004555116683));
#18662=CARTESIAN_POINT('Ctrl Pts',(95.2825019375973,-0.901718178386317,
2.01114877970292));
#18663=CARTESIAN_POINT('Ctrl Pts',(95.2817485597674,-0.888824322936559,
2.01688036902577));
#18664=CARTESIAN_POINT('Ctrl Pts',(95.2797389684467,-0.854093952055924,
2.03192100436055));
#18665=CARTESIAN_POINT('Ctrl Pts',(95.2784905193784,-0.832160303015017,
2.04100189483063));
#18666=CARTESIAN_POINT('Ctrl Pts',(95.2715036968061,-0.707489657566127,
2.09027365424749));
#18667=CARTESIAN_POINT('Ctrl Pts',(95.2660175869942,-0.601991578221309,
2.123062732397));
#18668=CARTESIAN_POINT('Ctrl Pts',(95.2525226581781,-0.332278619496873,
2.18515625133316));
#18669=CARTESIAN_POINT('Ctrl Pts',(95.2447107407989,-0.166398251888413,
2.2039999999985));
#18670=CARTESIAN_POINT('Ctrl Pts',(95.2361698906488,-1.99362401587244E-11,
2.204));
#18671=CARTESIAN_POINT('Ctrl Pts',(95.1243866264839,2.95869231892176E-11,
2.204));
#18672=CARTESIAN_POINT('Ctrl Pts',(95.1365232181435,-0.208374310327999,
2.2040000000028));
#18673=CARTESIAN_POINT('Ctrl Pts',(95.1493967605743,-0.41570994031362,2.17445261716368));
#18674=CARTESIAN_POINT('Ctrl Pts',(95.164981094345,-0.67481589797497,2.09905037989901));
#18675=CARTESIAN_POINT('Ctrl Pts',(95.1684599173385,-0.733054288206009,
2.07942815222445));
#18676=CARTESIAN_POINT('Ctrl Pts',(95.1729812526661,-0.809317108816974,
2.05012986019935));
#18677=CARTESIAN_POINT('Ctrl Pts',(95.1740940190293,-0.828132437153745,
2.04260209820613));
#18678=CARTESIAN_POINT('Ctrl Pts',(95.1759314248133,-0.859269290060516,
2.02964368339487));
#18679=CARTESIAN_POINT('Ctrl Pts',(95.1766609000501,-0.871649394051703,
2.02435780916168));
#18680=CARTESIAN_POINT('Ctrl Pts',(95.1780841027412,-0.895834899339802,
2.01376843247683));
#18681=CARTESIAN_POINT('Ctrl Pts',(95.1787780937438,-0.907643533002457,
2.00847372235246));
#18682=CARTESIAN_POINT('Ctrl Pts',(95.1804437470377,-0.936016495251098,
1.99545062484916));
#18683=CARTESIAN_POINT('Ctrl Pts',(95.1814118318033,-0.952532795577292,
1.98761952493749));
#18684=CARTESIAN_POINT('Ctrl Pts',(95.1846193798058,-1.00731505594976,1.96080516139552));
#18685=CARTESIAN_POINT('Ctrl Pts',(95.1868274237,-1.0451274403687,1.94091459021816));
#18686=CARTESIAN_POINT('Ctrl Pts',(95.1975079459947,-1.22781502606079,1.83792682001616));
#18687=CARTESIAN_POINT('Ctrl Pts',(95.2054300586328,-1.36349433174788,1.73965219684265));
#18688=CARTESIAN_POINT('Ctrl Pts',(95.218372533116,-1.5599291579796,1.56014640895244));
#18689=CARTESIAN_POINT('Ctrl Pts',(95.2232619555242,-1.62848229692825,1.48844790720758));
#18690=CARTESIAN_POINT('Ctrl Pts',(95.2293253611694,-1.70245547567915,1.39983176247767));
#18691=CARTESIAN_POINT('Ctrl Pts',(95.230193102341,-1.71279823376751,1.38715744922183));
#18692=CARTESIAN_POINT('Ctrl Pts',(95.2315305488298,-1.72834773036982,1.36766359372778));
#18693=CARTESIAN_POINT('Ctrl Pts',(95.2319932686743,-1.73365753174243,1.36092657417188));
#18694=CARTESIAN_POINT('Ctrl Pts',(95.232847531939,-1.74332881656237,1.34850730306119));
#18695=CARTESIAN_POINT('Ctrl Pts',(95.2332382396786,-1.74770208567038,1.34283458573826));
#18696=CARTESIAN_POINT('Ctrl Pts',(95.2341366496679,-1.75764470248694,1.32980683243689));
#18697=CARTESIAN_POINT('Ctrl Pts',(95.2346455866618,-1.76319556233371,1.32243809476048));
#18698=CARTESIAN_POINT('Ctrl Pts',(95.2362476175645,-1.78042146999106,1.29926953710171));
#18699=CARTESIAN_POINT('Ctrl Pts',(95.2373511489964,-1.79193132926847,1.2833487435218));
#18700=CARTESIAN_POINT('Ctrl Pts',(95.2464557668316,-1.88417171057394,1.15209857621129));
#18701=CARTESIAN_POINT('Ctrl Pts',(95.2549873615087,-1.95389018917339,1.02943786771139));
#18702=CARTESIAN_POINT('Ctrl Pts',(95.2660609338512,-2.02934889534617,0.860976278647757));
#18703=CARTESIAN_POINT('Ctrl Pts',(95.2686815784102,-2.04606950036018,0.820449178914159));
#18704=CARTESIAN_POINT('Ctrl Pts',(95.2755153672847,-2.08682444937102,0.71265617668105));
#18705=CARTESIAN_POINT('Ctrl Pts',(95.2796878499968,-2.10881859467256,0.644670930322019));
#18706=CARTESIAN_POINT('Ctrl Pts',(95.2864528238454,-2.13977971642495,0.530262010079944));
#18707=CARTESIAN_POINT('Ctrl Pts',(95.2890984373194,-2.15062464293121,0.484405982417027));
#18708=CARTESIAN_POINT('Ctrl Pts',(95.2927144408188,-2.16365750662576,0.420169023220054));
#18709=CARTESIAN_POINT('Ctrl Pts',(95.2937241813549,-2.16709614046601,0.402057410326371));
#18710=CARTESIAN_POINT('Ctrl Pts',(95.2954390690828,-2.1725889372381,0.371005260783025));
#18711=CARTESIAN_POINT('Ctrl Pts',(95.2961477585141,-2.17475564646544,0.358085858809067));
#18712=CARTESIAN_POINT('Ctrl Pts',(95.2974918891146,-2.17866657752132,0.333420064421395));
#18713=CARTESIAN_POINT('Ctrl Pts',(95.2981279575773,-2.18043129521987,0.321677431286295));
#18714=CARTESIAN_POINT('Ctrl Pts',(95.2996096601292,-2.18433916622332,0.29416277160753));
#18715=CARTESIAN_POINT('Ctrl Pts',(95.3004528845243,-2.18640655376888,0.278380546663963));
#18716=CARTESIAN_POINT('Ctrl Pts',(95.3033742173839,-2.19301695926417,0.223289782382924));
#18717=CARTESIAN_POINT('Ctrl Pts',(95.3054246690753,-2.19667239832511,0.183881306837095));
#18718=CARTESIAN_POINT('Ctrl Pts',(95.31615093487,-2.21042544835393,-0.0255912422011547));
#18719=CARTESIAN_POINT('Ctrl Pts',(95.3242345960981,-2.20184179492465,-0.196291835706937));
#18720=CARTESIAN_POINT('Ctrl Pts',(95.3370656479402,-2.15821786981221,-0.456579914631635));
#18721=CARTESIAN_POINT('Ctrl Pts',(95.3416745219566,-2.13689435998858,-0.547767171442031));
#18722=CARTESIAN_POINT('Ctrl Pts',(95.3476275518187,-2.10385812124239,-0.657134446949495));
#18723=CARTESIAN_POINT('Ctrl Pts',(95.3487191855103,-2.09759238200129,-0.676868387191782));
#18724=CARTESIAN_POINT('Ctrl Pts',(95.3503296111129,-2.08807260963721,-0.705448459633346));
#18725=CARTESIAN_POINT('Ctrl Pts',(95.3508363710408,-2.08503820220943,-0.714367161264823));
#18726=CARTESIAN_POINT('Ctrl Pts',(95.3517316765413,-2.07961226763106,-0.729985906545175));
#18727=CARTESIAN_POINT('Ctrl Pts',(95.3521187859167,-2.07724534701003,-0.736694220376826));
#18728=CARTESIAN_POINT('Ctrl Pts',(95.3529677444057,-2.07200989516625,-0.751306656927748));
#18729=CARTESIAN_POINT('Ctrl Pts',(95.3534303059727,-2.06912864128166,-0.759205742488429));
#18730=CARTESIAN_POINT('Ctrl Pts',(95.3547315688507,-2.0609409712885,-0.781259773280101));
#18731=CARTESIAN_POINT('Ctrl Pts',(95.3555758612454,-2.05553411646912,-0.79537663452365));
#18732=CARTESIAN_POINT('Ctrl Pts',(95.3613899425521,-2.01762655312087,-0.891381522397193));
#18733=CARTESIAN_POINT('Ctrl Pts',(95.3665884186582,-1.98038890814476,-0.97130573327736));
#18734=CARTESIAN_POINT('Ctrl Pts',(95.3734099528768,-1.9260764533148,-1.0716922058127));
#18735=CARTESIAN_POINT('Ctrl Pts',(95.3749724793129,-1.91327453146763,-1.09438349446007));
#18736=CARTESIAN_POINT('Ctrl Pts',(95.3767810613996,-1.89801236690273,-1.12034887393804));
#18737=CARTESIAN_POINT('Ctrl Pts',(95.3770253481034,-1.895941542512,-1.12384972820635));
#18738=CARTESIAN_POINT('Ctrl Pts',(95.3831769747213,-1.84355640400101,-1.21185312384326));
#18739=CARTESIAN_POINT('Ctrl Pts',(95.3890872447023,-1.78764899766538,-1.29290419625753));
#18740=CARTESIAN_POINT('Ctrl Pts',(95.3998383935142,-1.67370880151235,-1.43649975285407));
#18741=CARTESIAN_POINT('Ctrl Pts',(95.4047075263484,-1.61709787956617,-1.49994326042428));
#18742=CARTESIAN_POINT('Ctrl Pts',(95.4106701402952,-1.54109606968516,-1.57579860014933));
#18743=CARTESIAN_POINT('Ctrl Pts',(95.4119040966367,-1.52499172095209,-1.59138889894475));
#18744=CARTESIAN_POINT('Ctrl Pts',(95.41388687776,-1.49850746550191,-1.61625648210513));
#18745=CARTESIAN_POINT('Ctrl Pts',(95.4146422100684,-1.48827285673878,-1.62568556507322));
#18746=CARTESIAN_POINT('Ctrl Pts',(95.4160879351943,-1.46840538832137,-1.64364446702353));
#18747=CARTESIAN_POINT('Ctrl Pts',(95.416778897694,-1.45878581941757,-1.65218808288144));
#18748=CARTESIAN_POINT('Ctrl Pts',(95.4183612773613,-1.43647285419564,-1.67165852659969));
#18749=CARTESIAN_POINT('Ctrl Pts',(95.4192502146911,-1.42372853349891,-1.68252595051968));
#18750=CARTESIAN_POINT('Ctrl Pts',(95.4221187786421,-1.38193494232217,-1.71734954849029));
#18751=CARTESIAN_POINT('Ctrl Pts',(95.4240743621843,-1.35239467543153,-1.74070747581657));
#18752=CARTESIAN_POINT('Ctrl Pts',(95.4348770846008,-1.18372154576252,-1.86719278265541));
#18753=CARTESIAN_POINT('Ctrl Pts',(95.4430972445935,-1.03341718186852,-1.95439429238572));
#18754=CARTESIAN_POINT('Ctrl Pts',(95.4561059448002,-0.787724484200567,
-2.06059029987708));
#18755=CARTESIAN_POINT('Ctrl Pts',(95.4607569631639,-0.698687068520469,
-2.09245677123985));
#18756=CARTESIAN_POINT('Ctrl Pts',(95.466761642407,-0.587900479160854,-2.1242460998172));
#18757=CARTESIAN_POINT('Ctrl Pts',(95.4678579635149,-0.567831831268026,
-2.12969843300575));
#18758=CARTESIAN_POINT('Ctrl Pts',(95.4694740602982,-0.538548417489966,
-2.13721095499995));
#18759=CARTESIAN_POINT('Ctrl Pts',(95.4699816845928,-0.529392265271298,
-2.13949734448097));
#18760=CARTESIAN_POINT('Ctrl Pts',(95.4708814260211,-0.513244831564596,
-2.1434195329337));
#18761=CARTESIAN_POINT('Ctrl Pts',(95.4712721312545,-0.506259837686835,
-2.14508007462445));
#18762=CARTESIAN_POINT('Ctrl Pts',(95.4721256321703,-0.491061226771371,
-2.14861486603422));
#18763=CARTESIAN_POINT('Ctrl Pts',(95.4725891134535,-0.482845058925799,
-2.15047613686241));
#18764=CARTESIAN_POINT('Ctrl Pts',(95.4738953834714,-0.459785370881456,
-2.15556121130354));
#18765=CARTESIAN_POINT('Ctrl Pts',(95.474743829131,-0.444919174422494,-2.15867867573241));
#18766=CARTESIAN_POINT('Ctrl Pts',(95.4807576018875,-0.340222848533257,
-2.1795062501068));
#18767=CARTESIAN_POINT('Ctrl Pts',(95.4861696692407,-0.249405281304239,
-2.19175568140264));
#18768=CARTESIAN_POINT('Ctrl Pts',(95.4929575523962,-0.13623173004743,-2.19989489871128));
#18769=CARTESIAN_POINT('Ctrl Pts',(95.4942726285816,-0.114342376030421,
-2.20114117179202));
#18770=CARTESIAN_POINT('Ctrl Pts',(95.5008280132533,-0.00526513338524706,
-2.20572002255719));
#18771=CARTESIAN_POINT('Ctrl Pts',(95.5060785569923,0.0820517259273758,
-2.2041998870168));
#18772=CARTESIAN_POINT('Ctrl Pts',(95.5170771629765,0.267674385976381,-2.18992022701718));
#18773=CARTESIAN_POINT('Ctrl Pts',(95.522783604233,0.365684163414786,-2.17570203665381));
#18774=CARTESIAN_POINT('Ctrl Pts',(95.5295808734159,0.485212425378219,-2.15005312158552));
#18775=CARTESIAN_POINT('Ctrl Pts',(95.5308657246521,0.50792865020553,-2.14480023980593));
#18776=CARTESIAN_POINT('Ctrl Pts',(95.532909601277,0.544251894957292,-2.1357914073827));
#18777=CARTESIAN_POINT('Ctrl Pts',(95.5336758879201,0.55791318582489,-2.1322635744938));
#18778=CARTESIAN_POINT('Ctrl Pts',(95.5351297429573,0.583910294686016,-2.12528323457521));
#18779=CARTESIAN_POINT('Ctrl Pts',(95.5358180275369,0.596251687883568,-2.12185390489184));
#18780=CARTESIAN_POINT('Ctrl Pts',(95.5373768491492,0.624274450115005,-2.11380336009496));
#18781=CARTESIAN_POINT('Ctrl Pts',(95.5382451573113,0.639935800518757,-2.10911484392925));
#18782=CARTESIAN_POINT('Ctrl Pts',(95.5405380110859,0.681413869186917,-2.09619306152914));
#18783=CARTESIAN_POINT('Ctrl Pts',(95.5419526883277,0.707133767294113,-2.08765709130422));
#18784=CARTESIAN_POINT('Ctrl Pts',(95.5520602599066,0.891577032631412,-2.02264378667209));
#18785=CARTESIAN_POINT('Ctrl Pts',(95.5601287313344,1.04351679964959,-1.94860846897075));
#18786=CARTESIAN_POINT('Ctrl Pts',(95.5740572533467,1.2860562419468,-1.79384788958586));
#18787=CARTESIAN_POINT('Ctrl Pts',(95.5798691309457,1.38118380651887,-1.72167234543653));
#18788=CARTESIAN_POINT('Ctrl Pts',(95.586957766528,1.48156151362213,-1.63181873150593));
#18789=CARTESIAN_POINT('Ctrl Pts',(95.5877821290291,1.49301576034949,-1.62134536834477));
#18790=CARTESIAN_POINT('Ctrl Pts',(95.5890662297948,1.51049928269737,-1.60501667506057));
#18791=CARTESIAN_POINT('Ctrl Pts',(95.5895198131222,1.51660749695779,-1.59924616794208));
#18792=CARTESIAN_POINT('Ctrl Pts',(95.5903661412603,1.52787566440592,-1.58847837593784));
#18793=CARTESIAN_POINT('Ctrl Pts',(95.5907581744162,1.53304435866003,-1.58349063347602));
#18794=CARTESIAN_POINT('Ctrl Pts',(95.5916628303367,1.54485628919361,-1.57198019149917));
#18795=CARTESIAN_POINT('Ctrl Pts',(95.5921767377798,1.55148266141522,-1.5654405838714));
#18796=CARTESIAN_POINT('Ctrl Pts',(95.593839953109,1.57266889431303,-1.54426511540557));
#18797=CARTESIAN_POINT('Ctrl Pts',(95.5950009904635,1.5870642088126,-1.52946700916441));
#18798=CARTESIAN_POINT('Ctrl Pts',(95.6031589120318,1.68568228183387,-1.42519809137343));
#18799=CARTESIAN_POINT('Ctrl Pts',(95.6105559184847,1.7624960336327,-1.32902883771935));
#18800=CARTESIAN_POINT('Ctrl Pts',(95.6246488207518,1.89309256830612,-1.13415197819525));
#18801=CARTESIAN_POINT('Ctrl Pts',(95.6313274130144,1.94815103679543,-1.03673125079674));
#18802=CARTESIAN_POINT('Ctrl Pts',(95.640207748459,2.01336603397346,-0.897623315262396));
#18803=CARTESIAN_POINT('Ctrl Pts',(95.6425976823674,2.03006154496583,-0.859197791878371));
#18804=CARTESIAN_POINT('Ctrl Pts',(95.6467460481698,2.05752911794181,-0.790701044938781));
#18805=CARTESIAN_POINT('Ctrl Pts',(95.648518844407,2.06876148045784,-0.760828693654273));
#18806=CARTESIAN_POINT('Ctrl Pts',(95.6511415320845,2.08460596864497,-0.715741625604498));
#18807=CARTESIAN_POINT('Ctrl Pts',(95.6520075361149,2.08970835938994,-0.700704724144734));
#18808=CARTESIAN_POINT('Ctrl Pts',(95.6535518824247,2.09857192153973,-0.673625274668912));
#18809=CARTESIAN_POINT('Ctrl Pts',(95.6542321742847,2.10239300148169,-0.661603202148736));
#18810=CARTESIAN_POINT('Ctrl Pts',(95.6556877164406,2.11038696478498,-0.635683407487274));
#18811=CARTESIAN_POINT('Ctrl Pts',(95.6564618405965,2.11452625516245,-0.621775896664761));
#18812=CARTESIAN_POINT('Ctrl Pts',(95.6585334509355,2.12529622520616,-0.584238185542508));
#18813=CARTESIAN_POINT('Ctrl Pts',(95.6598225976398,2.13167015555374,-0.560536094943628));
#18814=CARTESIAN_POINT('Ctrl Pts',(95.6678235601166,2.16911179324852,-0.411416925225732));
#18815=CARTESIAN_POINT('Ctrl Pts',(95.6741801527703,2.18949784149983,-0.283573553024865));
#18816=CARTESIAN_POINT('Ctrl Pts',(95.6850276761911,2.20520178753177,-0.0603466277874939));
#18817=CARTESIAN_POINT('Ctrl Pts',(95.6895563009695,2.20576043389339,0.0343016631780244));
#18818=CARTESIAN_POINT('Ctrl Pts',(95.6966991527222,2.19729268525846,0.179076170279175));
#18819=CARTESIAN_POINT('Ctrl Pts',(95.6992204194252,2.19261590158227,0.229343404499276));
#18820=CARTESIAN_POINT('Ctrl Pts',(95.7028913980054,2.18354545068685,0.300316114566162));
#18821=CARTESIAN_POINT('Ctrl Pts',(95.7039848063516,2.18057284949141,0.321189189266353));
#18822=CARTESIAN_POINT('Ctrl Pts',(95.7059471268011,2.1747766844933,0.358088071407927));
#18823=CARTESIAN_POINT('Ctrl Pts',(95.7068102461365,2.17207418910339,0.37413150152327));
#18824=CARTESIAN_POINT('Ctrl Pts',(95.7081420151513,2.167679232232,0.398567449897152));
#18825=CARTESIAN_POINT('Ctrl Pts',(95.7086037700983,2.16611501767912,0.406982789752063));
#18826=CARTESIAN_POINT('Ctrl Pts',(95.7094571660707,2.16315153019367,0.422424891951736));
#18827=CARTESIAN_POINT('Ctrl Pts',(95.7098479843354,2.16176696820754,0.429454191811165));
#18828=CARTESIAN_POINT('Ctrl Pts',(95.7107478465878,2.15851638915541,0.445542985443602));
#18829=CARTESIAN_POINT('Ctrl Pts',(95.7112581412518,2.15662760200299,0.454597551789988));
#18830=CARTESIAN_POINT('Ctrl Pts',(95.7128687393648,2.15052232360286,0.482970726759335));
#18831=CARTESIAN_POINT('Ctrl Pts',(95.7139796340458,2.14610292427187,0.502244133966514));
#18832=CARTESIAN_POINT('Ctrl Pts',(95.7229895926815,2.10855033481861,0.656458953458616));
#18833=CARTESIAN_POINT('Ctrl Pts',(95.7314048307316,2.06298494827918,0.788042533456589));
#18834=CARTESIAN_POINT('Ctrl Pts',(95.7487479361909,1.94306220184258,1.05102654663725));
#18835=CARTESIAN_POINT('Ctrl Pts',(95.7576054923856,1.86698486334045,1.18090144705656));
#18836=CARTESIAN_POINT('Ctrl Pts',(95.7673861039803,1.76334942018843,1.3224423349996));
#18837=CARTESIAN_POINT('Ctrl Pts',(95.7687820044639,1.74806671521988,1.34257876541355));
#18838=CARTESIAN_POINT('Ctrl Pts',(95.7709589004507,1.72345924121324,1.37386874572588));
#18839=CARTESIAN_POINT('Ctrl Pts',(95.7717489113165,1.71436509842713,1.38520013360085));
#18840=CARTESIAN_POINT('Ctrl Pts',(95.7732228567288,1.69709168361481,1.40629227189789));
#18841=CARTESIAN_POINT('Ctrl Pts',(95.7739078042913,1.68893861664057,1.41607361929557));
#18842=CARTESIAN_POINT('Ctrl Pts',(95.7754409038375,1.67040818160355,1.43791712781092));
#18843=CARTESIAN_POINT('Ctrl Pts',(95.7762870848897,1.65998398318963,1.44993874117821));
#18844=CARTESIAN_POINT('Ctrl Pts',(95.7787680565528,1.62884817561953,1.48506988558187));
#18845=CARTESIAN_POINT('Ctrl Pts',(95.7803878099119,1.60777724573105,1.50785655730095));
#18846=CARTESIAN_POINT('Ctrl Pts',(95.7893344695021,1.4873998114667,1.63264255748545));
#18847=CARTESIAN_POINT('Ctrl Pts',(95.7962413657524,1.37887401218256,1.72528000637141));
#18848=CARTESIAN_POINT('Ctrl Pts',(95.8079801417246,1.1797677045359,1.86436744725722));
#18849=CARTESIAN_POINT('Ctrl Pts',(95.8128201104091,1.09353676705612,1.91621837215105));
#18850=CARTESIAN_POINT('Ctrl Pts',(95.8202718266607,0.961749684533358,1.98366180117435));
#18851=CARTESIAN_POINT('Ctrl Pts',(95.8227128197106,0.918737412880803,2.00394549691982));
#18852=CARTESIAN_POINT('Ctrl Pts',(95.8259065174295,0.863373693755141,2.0278967612562));
#18853=CARTESIAN_POINT('Ctrl Pts',(95.8265887372844,0.851597704004847,2.03287007561598));
#18854=CARTESIAN_POINT('Ctrl Pts',(95.8276974344113,0.832558451105272,2.04071639952598));
#18855=CARTESIAN_POINT('Ctrl Pts',(95.8281201522932,0.82532184801243,2.04365379678735));
#18856=CARTESIAN_POINT('Ctrl Pts',(95.8289420143414,0.811300404204055,2.04925859825603));
#18857=CARTESIAN_POINT('Ctrl Pts',(95.8293408653693,0.804517714741855,2.0519308930117));
#18858=CARTESIAN_POINT('Ctrl Pts',(95.8303281900514,0.787777955806871,2.05843039334748));
#18859=CARTESIAN_POINT('Ctrl Pts',(95.8309188918746,0.777806174994637,2.06221903214667));
#18860=CARTESIAN_POINT('Ctrl Pts',(95.8329892428514,0.742989191283577,2.07515881019842));
#18861=CARTESIAN_POINT('Ctrl Pts',(95.834488632611,0.718007781568828,2.0839341941399));
#18862=CARTESIAN_POINT('Ctrl Pts',(95.8442150073206,0.556976623642962,2.13726155619314));
#18863=CARTESIAN_POINT('Ctrl Pts',(95.852921678368,0.417023127279817,2.16891640321994));
#18864=CARTESIAN_POINT('Ctrl Pts',(95.8669634457191,0.18425917300624,2.19818742617519));
#18865=CARTESIAN_POINT('Ctrl Pts',(95.8723731099742,0.0928936498329579,
2.2039402670841));
#18866=CARTESIAN_POINT('Ctrl Pts',(95.8776583114079,0.000952142118494687,
2.20399984587122));
#18867=CARTESIAN_POINT('Ctrl Pts',(95.8776856739115,0.00047607047170703,
2.204));
#18868=CARTESIAN_POINT('Ctrl Pts',(95.8777130322977,9.44243789243157E-12,
2.204));
#18869=CARTESIAN_POINT('Origin',(66.9212607628943,0.,0.));
#18870=CARTESIAN_POINT('',(96.7328779004031,-1.24027783152639E-11,2.204));
#18871=CARTESIAN_POINT('',(96.6270503826334,2.66056133811156E-11,2.204));
#18872=CARTESIAN_POINT('',(66.9212607628943,-2.69912154532077E-16,2.204));
#18873=CARTESIAN_POINT('Ctrl Pts',(96.7328779004031,-1.24027783152639E-11,
2.204));
#18874=CARTESIAN_POINT('Ctrl Pts',(96.7298587062484,0.0517545618109105,
2.20400000000029));
#18875=CARTESIAN_POINT('Ctrl Pts',(96.7268830575451,0.103495927703961,2.20217705427766));
#18876=CARTESIAN_POINT('Ctrl Pts',(96.7221848298922,0.186495648980921,2.19632059943722));
#18877=CARTESIAN_POINT('Ctrl Pts',(96.720429239674,0.21781298812238,2.1934362192633));
#18878=CARTESIAN_POINT('Ctrl Pts',(96.7179163743073,0.263072049046784,2.18828882936624));
#18879=CARTESIAN_POINT('Ctrl Pts',(96.7171425675157,0.277069637214047,2.18656061725319));
#18880=CARTESIAN_POINT('Ctrl Pts',(96.7157268188338,0.302788217248647,2.18313433596879));
#18881=CARTESIAN_POINT('Ctrl Pts',(96.7150836534011,0.314513889386896,2.18147593488228));
#18882=CARTESIAN_POINT('Ctrl Pts',(96.7137618316973,0.338696114093211,2.17785672957963));
#18883=CARTESIAN_POINT('Ctrl Pts',(96.713083599525,0.351150366810158,2.17588336574876));
#18884=CARTESIAN_POINT('Ctrl Pts',(96.711563271397,0.379167539115507,2.17119725399933));
#18885=CARTESIAN_POINT('Ctrl Pts',(96.7107231352499,0.394719693527861,2.16842383302871));
#18886=CARTESIAN_POINT('Ctrl Pts',(96.7082535827562,0.440626351374217,2.15972702577093));
#18887=CARTESIAN_POINT('Ctrl Pts',(96.7066391420978,0.470888117383112,2.153331584336));
#18888=CARTESIAN_POINT('Ctrl Pts',(96.7003113553379,0.590290881787022,2.12545966350238));
#18889=CARTESIAN_POINT('Ctrl Pts',(96.6957518031178,0.678192929259821,2.09906612257732));
#18890=CARTESIAN_POINT('Ctrl Pts',(96.6867015964908,0.851930830914635,2.03484106666446));
#18891=CARTESIAN_POINT('Ctrl Pts',(96.6822229729324,0.93750659570956,1.99685893689979));
#18892=CARTESIAN_POINT('Ctrl Pts',(96.6731767779031,1.10235572269818,1.91075246792145));
#18893=CARTESIAN_POINT('Ctrl Pts',(96.6686184234022,1.18151960766259,1.86283961259836));
#18894=CARTESIAN_POINT('Ctrl Pts',(96.6627311490356,1.27427958075199,1.79840158965566));
#18895=CARTESIAN_POINT('Ctrl Pts',(96.6616493835604,1.29096063522673,1.7864650308343));
#18896=CARTESIAN_POINT('Ctrl Pts',(96.6600538392141,1.31498356875106,1.76876263951179));
#18897=CARTESIAN_POINT('Ctrl Pts',(96.6595518802614,1.32245970809196,1.76317990435572));
#18898=CARTESIAN_POINT('Ctrl Pts',(96.6586652879418,1.33551601020759,1.75330048302545));
#18899=CARTESIAN_POINT('Ctrl Pts',(96.6582820656044,1.34111135262955,1.74902428107412));
#18900=CARTESIAN_POINT('Ctrl Pts',(96.6574423249083,1.35326615873188,1.73964243244621));
#18901=CARTESIAN_POINT('Ctrl Pts',(96.6569851153289,1.35981716602655,1.73452655196312));
#18902=CARTESIAN_POINT('Ctrl Pts',(96.6557009744709,1.37803640082422,1.72013194849655));
#18903=CARTESIAN_POINT('Ctrl Pts',(96.6548686110781,1.38963944384994,1.71077188238951));
#18904=CARTESIAN_POINT('Ctrl Pts',(96.6493173880117,1.46574206377966,1.64809556865459));
#18905=CARTESIAN_POINT('Ctrl Pts',(96.6443915653548,1.52724993027945,1.59126486937166));
#18906=CARTESIAN_POINT('Ctrl Pts',(96.6374376088515,1.60819359062454,1.50745102446577));
#18907=CARTESIAN_POINT('Ctrl Pts',(96.6354670936563,1.63048349340914,1.48331343521399));
#18908=CARTESIAN_POINT('Ctrl Pts',(96.6279667872646,1.7131364560409,1.38969409152123));
#18909=CARTESIAN_POINT('Ctrl Pts',(96.6224320532924,1.76966914143734,1.31695055541269));
#18910=CARTESIAN_POINT('Ctrl Pts',(96.6115647818015,1.87357327411752,1.16442989091331));
#18911=CARTESIAN_POINT('Ctrl Pts',(96.6062444122136,1.92079611274914,1.08476700431298));
#18912=CARTESIAN_POINT('Ctrl Pts',(96.5998373135974,1.97324066745255,0.982067510776416));
#18913=CARTESIAN_POINT('Ctrl Pts',(96.5985820640037,1.98328968815008,0.961611873570815));
#18914=CARTESIAN_POINT('Ctrl Pts',(96.5965786147738,1.99895715881967,0.928428595108936));
#18915=CARTESIAN_POINT('Ctrl Pts',(96.5958235429508,2.00477534285466,0.915797584706416));
#18916=CARTESIAN_POINT('Ctrl Pts',(96.5943870091824,2.01567584981854,0.891531293400016));
#18917=CARTESIAN_POINT('Ctrl Pts',(96.5937048898292,2.02077792450716,0.879905544831762));
#18918=CARTESIAN_POINT('Ctrl Pts',(96.5921548841836,2.03219976820538,0.853255958858069));
#18919=CARTESIAN_POINT('Ctrl Pts',(96.5912892529352,2.03845395041385,0.838204712786434));
#18920=CARTESIAN_POINT('Ctrl Pts',(96.5889926972575,2.05470533783437,0.797836323920241));
#18921=CARTESIAN_POINT('Ctrl Pts',(96.5875718126063,2.06440164097361,0.772400656605027));
#18922=CARTESIAN_POINT('Ctrl Pts',(96.5775921605438,2.12983699459136,0.59070546889544));
#18923=CARTESIAN_POINT('Ctrl Pts',(96.5696359863537,2.16824727422706,0.428774070994789));
#18924=CARTESIAN_POINT('Ctrl Pts',(96.555715832866,2.20270903089398,0.143202550637772));
#18925=CARTESIAN_POINT('Ctrl Pts',(96.5497911605003,2.2072541266064,0.0213628324410037));
#18926=CARTESIAN_POINT('Ctrl Pts',(96.5425741760836,2.20101873445896,-0.115632143233154));
#18927=CARTESIAN_POINT('Ctrl Pts',(96.5417542281166,2.20015494612941,-0.131043688883808));
#18928=CARTESIAN_POINT('Ctrl Pts',(96.54047827966,2.1985755898818,-0.15476059050655));
#18929=CARTESIAN_POINT('Ctrl Pts',(96.5400283822173,2.19797464339611,-0.163073379662546));
#18930=CARTESIAN_POINT('Ctrl Pts',(96.5391899279623,2.19677393458744,-0.178467895348348));
#18931=CARTESIAN_POINT('Ctrl Pts',(96.538802081181,2.19618705246131,-0.185550358088997));
#18932=CARTESIAN_POINT('Ctrl Pts',(96.5379088132156,2.19476353542312,-0.201775391509915));
#18933=CARTESIAN_POINT('Ctrl Pts',(96.5374021550974,2.19390402140018,-0.210915679265884));
#18934=CARTESIAN_POINT('Ctrl Pts',(96.5357696590319,2.19096774919756,-0.240178134856074));
#18935=CARTESIAN_POINT('Ctrl Pts',(96.5346325734951,2.18867111050859,-0.260276632143668));
#18936=CARTESIAN_POINT('Ctrl Pts',(96.5258988237355,2.16911475275039,-0.412777635752838));
#18937=CARTESIAN_POINT('Ctrl Pts',(96.5178279836494,2.14013273103775,-0.543388703291366));
#18938=CARTESIAN_POINT('Ctrl Pts',(96.5035189610641,2.06761705366597,-0.770432986581292));
#18939=CARTESIAN_POINT('Ctrl Pts',(96.497274181195,2.02863230900659,-0.86790649589299));
#18940=CARTESIAN_POINT('Ctrl Pts',(96.487750334366,1.95656074921,-1.01642159639436));
#18941=CARTESIAN_POINT('Ctrl Pts',(96.4843422138979,1.92805685706703,-1.06950482067662));
#18942=CARTESIAN_POINT('Ctrl Pts',(96.4799031192365,1.88723268634588,-1.13858205323129));
#18943=CARTESIAN_POINT('Ctrl Pts',(96.4788047072727,1.87681886184179,-1.15566747011969));
#18944=CARTESIAN_POINT('Ctrl Pts',(96.4769894666453,1.85908921644074,-1.18388368911044));
#18945=CARTESIAN_POINT('Ctrl Pts',(96.4762679371796,1.85190271705765,-1.19509398856278));
#18946=CARTESIAN_POINT('Ctrl Pts',(96.4748593059076,1.83760027569854,-1.21696569465826));
#18947=CARTESIAN_POINT('Ctrl Pts',(96.4741719545914,1.83049206110129,-1.22763149969902));
#18948=CARTESIAN_POINT('Ctrl Pts',(96.4725209436016,1.81310797930154,-1.25322942380201));
#18949=CARTESIAN_POINT('Ctrl Pts',(96.4715608104923,1.80274007529805,-1.26809809577788));
#18950=CARTESIAN_POINT('Ctrl Pts',(96.4683742223232,1.76747742709525,-1.31736182273613));
#18951=CARTESIAN_POINT('Ctrl Pts',(96.4661788483208,1.74177176961209,-1.35116617594726));
#18952=CARTESIAN_POINT('Ctrl Pts',(96.4554881932676,1.60997993211048,-1.51446295414412));
#18953=CARTESIAN_POINT('Ctrl Pts',(96.4475477520423,1.49036363473989,-1.63231477228739));
#18954=CARTESIAN_POINT('Ctrl Pts',(96.4349001214269,1.2855960016709,-1.79260817523177));
#18955=CARTESIAN_POINT('Ctrl Pts',(96.4303323226413,1.20911321032597,-1.84505914537632));
#18956=CARTESIAN_POINT('Ctrl Pts',(96.4244334792825,1.11193485019172,-1.90306028906805));
#18957=CARTESIAN_POINT('Ctrl Pts',(96.423350653709,1.09415855698485,-1.91333597870521));
#18958=CARTESIAN_POINT('Ctrl Pts',(96.4217538268103,1.06809611167613,-1.9279195592932));
#18959=CARTESIAN_POINT('Ctrl Pts',(96.4212516721216,1.05992155539367,-1.93242578665264));
#18960=CARTESIAN_POINT('Ctrl Pts',(96.4203614126176,1.04547342448672,-1.94027106954058));
#18961=CARTESIAN_POINT('Ctrl Pts',(96.4199746868572,1.03921197453441,-1.94363190320233));
#18962=CARTESIAN_POINT('Ctrl Pts',(96.4191300348318,1.02557000091429,-1.9508694649369));
#18963=CARTESIAN_POINT('Ctrl Pts',(96.4186714376794,1.01818381162755,-1.95473456434584));
#18964=CARTESIAN_POINT('Ctrl Pts',(96.4173797509022,0.997431044739363,-1.96544469033682));
#18965=CARTESIAN_POINT('Ctrl Pts',(96.4165411310799,0.98401641919931,-1.97219501602865));
#18966=CARTESIAN_POINT('Ctrl Pts',(96.410744421575,0.891605491706431,-2.01751926707621));
#18967=CARTESIAN_POINT('Ctrl Pts',(96.4055582108929,0.8104381691074,-2.05147055941209));
#18968=CARTESIAN_POINT('Ctrl Pts',(96.3985615152765,0.699920226692501,-2.09011469096104));
#18969=CARTESIAN_POINT('Ctrl Pts',(96.3968104610436,0.672182761178849,-2.09919938336));
#18970=CARTESIAN_POINT('Ctrl Pts',(96.3894447416618,0.554902356093236,-2.13504867185127));
#18971=CARTESIAN_POINT('Ctrl Pts',(96.3838258973558,0.463880063521639,-2.15665628082435));
#18972=CARTESIAN_POINT('Ctrl Pts',(96.3729995290388,0.282476290138551,-2.18769919487842));
#18973=CARTESIAN_POINT('Ctrl Pts',(96.367794764798,0.192330452159084,-2.1974605338748));
#18974=CARTESIAN_POINT('Ctrl Pts',(96.361502920852,0.0791899529410651,-2.20269349493717));
#18975=CARTESIAN_POINT('Ctrl Pts',(96.3602546855457,0.0565342480874049,
-2.20339138926516));
#18976=CARTESIAN_POINT('Ctrl Pts',(96.3582596583508,0.0199934536269167,
-2.20395301649099));
#18977=CARTESIAN_POINT('Ctrl Pts',(96.3575060976031,0.00611379565499054,
-2.20403522453194));
#18978=CARTESIAN_POINT('Ctrl Pts',(96.3560707000286,-0.0204690278131193,
-2.20394155760186));
#18979=CARTESIAN_POINT('Ctrl Pts',(96.3553882256754,-0.0331716689551365,
-2.20378697250126));
#18980=CARTESIAN_POINT('Ctrl Pts',(96.3538350414583,-0.062221193836304,
-2.20318222583736));
#18981=CARTESIAN_POINT('Ctrl Pts',(96.3529666201739,-0.0785659273935716,
-2.20265994010033));
#18982=CARTESIAN_POINT('Ctrl Pts',(96.3506573723257,-0.122287881182493,
-2.20077553689516));
#18983=CARTESIAN_POINT('Ctrl Pts',(96.3492267672784,-0.14964845323569,-2.19908451777842));
#18984=CARTESIAN_POINT('Ctrl Pts',(96.3393693434932,-0.339835212465662,
-2.18376391691758));
#18985=CARTESIAN_POINT('Ctrl Pts',(96.3315239046375,-0.500734303607521,
-2.15257587248012));
#18986=CARTESIAN_POINT('Ctrl Pts',(96.3194567346258,-0.738832767997645,
-2.07825452945098));
#18987=CARTESIAN_POINT('Ctrl Pts',(96.3152780830522,-0.81937152232122,-2.04783894355926));
#18988=CARTESIAN_POINT('Ctrl Pts',(96.3087323218619,-0.937625363321509,
-1.99508515793927));
#18989=CARTESIAN_POINT('Ctrl Pts',(96.3064923112489,-0.976793923398442,
-1.97620324417918));
#18990=CARTESIAN_POINT('Ctrl Pts',(96.3035343874477,-1.02632970060474,-1.95049113229691));
#18991=CARTESIAN_POINT('Ctrl Pts',(96.302875212988,-1.03723524986854,-1.9447136894284));
#18992=CARTESIAN_POINT('Ctrl Pts',(96.3017976320076,-1.05483302867817,-1.9352007677892));
#18993=CARTESIAN_POINT('Ctrl Pts',(96.3013826695694,-1.06155544978605,-1.93152135722222));
#18994=CARTESIAN_POINT('Ctrl Pts',(96.3005704859288,-1.07460352443904,-1.9242910090979));
#18995=CARTESIAN_POINT('Ctrl Pts',(96.3001734938825,-1.08093105211585,-1.92074378251485));
#18996=CARTESIAN_POINT('Ctrl Pts',(96.2992782748842,-1.09509041342977,-1.91271388845832));
#18997=CARTESIAN_POINT('Ctrl Pts',(96.2987789919525,-1.10291245896627,-1.90821422664363));
#18998=CARTESIAN_POINT('Ctrl Pts',(96.2972685697199,-1.12635969329858,-1.89453378808253));
#18999=CARTESIAN_POINT('Ctrl Pts',(96.2962490116705,-1.14189913779627,-1.88520841012762));
#19000=CARTESIAN_POINT('Ctrl Pts',(96.2875501055493,-1.27225408843843,-1.80477809475657));
#19001=CARTESIAN_POINT('Ctrl Pts',(96.2793825462485,-1.38041768628292,-1.72345484399622));
#19002=CARTESIAN_POINT('Ctrl Pts',(96.2620224217044,-1.59466361771938,-1.52919355031917));
#19003=CARTESIAN_POINT('Ctrl Pts',(96.2529129148622,-1.69771174068804,-1.41392152406733));
#19004=CARTESIAN_POINT('Ctrl Pts',(96.2429294759101,-1.80246924960868,-1.26859842126896));
#19005=CARTESIAN_POINT('Ctrl Pts',(96.2415533500128,-1.81670190309005,-1.24813125014843));
#19006=CARTESIAN_POINT('Ctrl Pts',(96.2394050181618,-1.83858429092446,-1.2154958400654));
#19007=CARTESIAN_POINT('Ctrl Pts',(96.2386240650529,-1.84646717528242,-1.20348714841613));
#19008=CARTESIAN_POINT('Ctrl Pts',(96.2371659376323,-1.8610473007181,-1.18079544781625));
#19009=CARTESIAN_POINT('Ctrl Pts',(96.2364877827042,-1.86777133252527,-1.1701304216466));
#19010=CARTESIAN_POINT('Ctrl Pts',(96.2349686945983,-1.88270170864102,-1.14599263121544));
#19011=CARTESIAN_POINT('Ctrl Pts',(96.2341297072409,-1.89085571056936,-1.13248820473646));
#19012=CARTESIAN_POINT('Ctrl Pts',(96.2316669347595,-1.91450914345224,-1.09234630607763));
#19013=CARTESIAN_POINT('Ctrl Pts',(96.230057999298,-1.92959598805286,-1.06546945438629));
#19014=CARTESIAN_POINT('Ctrl Pts',(96.2208902421419,-2.01327070776364,-0.908794369701065));
#19015=CARTESIAN_POINT('Ctrl Pts',(96.2137825675048,-2.06931817481662,-0.772718120787975));
#19016=CARTESIAN_POINT('Ctrl Pts',(96.2019722323974,-2.13939872201444,-0.538614425396601));
#19017=CARTESIAN_POINT('Ctrl Pts',(96.1972664119603,-2.16113786367353,-0.443411023906599));
#19018=CARTESIAN_POINT('Ctrl Pts',(96.190770106816,-2.18144316652708,-0.316081511794287));
#19019=CARTESIAN_POINT('Ctrl Pts',(96.1891669793782,-2.18572436781954,-0.284974799212456));
#19020=CARTESIAN_POINT('Ctrl Pts',(96.1863915083369,-2.19187086812668,-0.231951235647986));
#19021=CARTESIAN_POINT('Ctrl Pts',(96.1852342482009,-2.19407530070379,-0.210078034978104));
#19022=CARTESIAN_POINT('Ctrl Pts',(96.1835475923921,-2.19677102643225,-0.178619860766554));
#19023=CARTESIAN_POINT('Ctrl Pts',(96.1830319920775,-2.19752753828242,-0.169058300116004));
#19024=CARTESIAN_POINT('Ctrl Pts',(96.1821268192902,-2.19873790515057,-0.152376273290863));
#19025=CARTESIAN_POINT('Ctrl Pts',(96.1817387926847,-2.1992196328568,-0.145258079537501));
#19026=CARTESIAN_POINT('Ctrl Pts',(96.1809018371755,-2.20017923892677,-0.12997754920019));
#19027=CARTESIAN_POINT('Ctrl Pts',(96.1804523526847,-2.20064625762887,-0.121814986954735));
#19028=CARTESIAN_POINT('Ctrl Pts',(96.1792099453642,-2.20180537330854,-0.099366339046418));
#19029=CARTESIAN_POINT('Ctrl Pts',(96.1784121188526,-2.2024038259397,-0.0850760645741195));
#19030=CARTESIAN_POINT('Ctrl Pts',(96.1739629677143,-2.20494451851432,-0.00600443790338455));
#19031=CARTESIAN_POINT('Ctrl Pts',(96.1701874461072,-2.20416748301859,0.0588277015573228));
#19032=CARTESIAN_POINT('Ctrl Pts',(96.1586782428498,-2.19327258113049,0.25291414937311));
#19033=CARTESIAN_POINT('Ctrl Pts',(96.1507986496064,-2.17461207464266,0.381410593607804));
#19034=CARTESIAN_POINT('Ctrl Pts',(96.1389275963061,-2.12848995926026,0.576319375782066));
#19035=CARTESIAN_POINT('Ctrl Pts',(96.1347994120104,-2.10890976081063,0.644293785467398));
#19036=CARTESIAN_POINT('Ctrl Pts',(96.1281014541804,-2.0710249581277,0.755415431289594));
#19037=CARTESIAN_POINT('Ctrl Pts',(96.1254796049882,-2.05455361061072,0.799128760987092));
#19038=CARTESIAN_POINT('Ctrl Pts',(96.1218960358074,-2.0297241599183,0.859167905062853));
#19039=CARTESIAN_POINT('Ctrl Pts',(96.1208956258372,-2.02253376811235,0.875960524036639));
#19040=CARTESIAN_POINT('Ctrl Pts',(96.1191969427666,-2.00988157748188,0.904522141607754));
#19041=CARTESIAN_POINT('Ctrl Pts',(96.1184951864292,-2.00452319096668,0.916335662904017));
#19042=CARTESIAN_POINT('Ctrl Pts',(96.1171645534972,-1.99411260818709,0.938759277380746));
#19043=CARTESIAN_POINT('Ctrl Pts',(96.116535057678,-1.98907925715543,0.949377580905073));
#19044=CARTESIAN_POINT('Ctrl Pts',(96.1149108389728,-1.97581237671403,0.976796541353063));
#19045=CARTESIAN_POINT('Ctrl Pts',(96.1139206487809,-1.96744932289345,0.993533704451851));
#19046=CARTESIAN_POINT('Ctrl Pts',(96.1105119383601,-1.93771430084698,1.05119487221928));
#19047=CARTESIAN_POINT('Ctrl Pts',(96.1081309597193,-1.91526976558125,1.09155370110274));
#19048=CARTESIAN_POINT('Ctrl Pts',(96.0974763412222,-1.80754904164396,1.27168565626526));
#19049=CARTESIAN_POINT('Ctrl Pts',(96.0897122521212,-1.70813519191704,1.40238852894118));
#19050=CARTESIAN_POINT('Ctrl Pts',(96.0772977374628,-1.53208161842689,1.58704068838235));
#19051=CARTESIAN_POINT('Ctrl Pts',(96.0727871653501,-1.46495250369248,1.64920688511033));
#19052=CARTESIAN_POINT('Ctrl Pts',(96.0669584126072,-1.37836034115307,1.71992883688432));
#19053=CARTESIAN_POINT('Ctrl Pts',(96.0658820361031,-1.36237717049087,1.73261675528396));
#19054=CARTESIAN_POINT('Ctrl Pts',(96.0642930129819,-1.33884798798936,1.75076805165262));
#19055=CARTESIAN_POINT('Ctrl Pts',(96.063792050911,-1.33143943644156,1.75640875834419));
#19056=CARTESIAN_POINT('Ctrl Pts',(96.062903092883,-1.31831572276943,1.76627011798733));
#19057=CARTESIAN_POINT('Ctrl Pts',(96.0625164611658,-1.3126155828012,1.77051032329445));
#19058=CARTESIAN_POINT('Ctrl Pts',(96.0616710315912,-1.30016964150332,1.77967543635046));
#19059=CARTESIAN_POINT('Ctrl Pts',(96.0612115518424,-1.29341641468204,1.78458951273183));
#19060=CARTESIAN_POINT('Ctrl Pts',(96.0599150569335,-1.27438604106841,1.79827245982117));
#19061=CARTESIAN_POINT('Ctrl Pts',(96.059072448671,-1.26204677432791,1.80695366161149));
#19062=CARTESIAN_POINT('Ctrl Pts',(96.0530872532332,-1.17451705150402,1.8672006624702));
#19063=CARTESIAN_POINT('Ctrl Pts',(96.0476995364777,-1.09628570846837,1.91417950182016));
#19064=CARTESIAN_POINT('Ctrl Pts',(96.0406855852496,-0.992209795841663,
1.96820150625176));
#19065=CARTESIAN_POINT('Ctrl Pts',(96.0391190826225,-0.968828842654001,
1.97981516871026));
#19066=CARTESIAN_POINT('Ctrl Pts',(96.0318024193023,-0.85878304360612,2.0320602397704));
#19067=CARTESIAN_POINT('Ctrl Pts',(96.0260484077454,-0.769732212170165,
2.06743590041368));
#19068=CARTESIAN_POINT('Ctrl Pts',(96.0169783399809,-0.622860145118887,
2.11497069620432));
#19069=CARTESIAN_POINT('Ctrl Pts',(96.0135832293551,-0.566358424110971,
2.13079674148879));
#19070=CARTESIAN_POINT('Ctrl Pts',(96.0079328538014,-0.469476629841306,
2.15380642984758));
#19071=CARTESIAN_POINT('Ctrl Pts',(96.0056442138879,-0.429406823009307,
2.16215183050514));
#19072=CARTESIAN_POINT('Ctrl Pts',(96.0024339138942,-0.372021230694282,
2.17244520913536));
#19073=CARTESIAN_POINT('Ctrl Pts',(96.0014834649776,-0.354880547292618,
2.17531096727852));
#19074=CARTESIAN_POINT('Ctrl Pts',(95.9998432633233,-0.325043132595704,
2.17993743070849));
#19075=CARTESIAN_POINT('Ctrl Pts',(95.9991506125998,-0.312361790341013,
2.18179063190975));
#19076=CARTESIAN_POINT('Ctrl Pts',(95.9977314513991,-0.286215649674768,
2.1853788890441));
#19077=CARTESIAN_POINT('Ctrl Pts',(95.9970053974418,-0.272749519469492,
2.1871003629818));
#19078=CARTESIAN_POINT('Ctrl Pts',(95.9951530702239,-0.238171515371894,
2.19119639507796));
#19079=CARTESIAN_POINT('Ctrl Pts',(95.9940325028907,-0.217039406713831,
2.19339035519573));
#19080=CARTESIAN_POINT('Ctrl Pts',(95.9895002557444,-0.13075063062194,2.20108965406977));
#19081=CARTESIAN_POINT('Ctrl Pts',(95.9861693214704,-0.065393673492086,
2.20399999999966));
#19082=CARTESIAN_POINT('Ctrl Pts',(95.9829026914895,-1.13898760397551E-11,
2.204));
#19083=CARTESIAN_POINT('Ctrl Pts',(95.8777130322977,9.44243789243157E-12,
2.204));
#19084=CARTESIAN_POINT('Ctrl Pts',(95.8808140072998,-0.0539608801586369,
2.204));
#19085=CARTESIAN_POINT('Ctrl Pts',(95.8838604928531,-0.107906633747905,
2.20201831932735));
#19086=CARTESIAN_POINT('Ctrl Pts',(95.8879545246214,-0.181710970242176,
2.19658793759466));
#19087=CARTESIAN_POINT('Ctrl Pts',(95.889054454545,-0.201672495502803,2.19484525338729));
#19088=CARTESIAN_POINT('Ctrl Pts',(95.8908034985033,-0.233620308559798,
2.19161660005351));
#19089=CARTESIAN_POINT('Ctrl Pts',(95.8914580149408,-0.24562264019355,2.19030392798998));
#19090=CARTESIAN_POINT('Ctrl Pts',(95.8928075722312,-0.270464880329532,
2.18738021103148));
#19091=CARTESIAN_POINT('Ctrl Pts',(95.8935021254901,-0.283302625147236,
2.18575457715834));
#19092=CARTESIAN_POINT('Ctrl Pts',(95.8951287693371,-0.313487137988951,
2.18166193122109));
#19093=CARTESIAN_POINT('Ctrl Pts',(95.8960578569719,-0.330820409300836,
2.17910092663289));
#19094=CARTESIAN_POINT('Ctrl Pts',(95.8991486766197,-0.388770164135528,
2.16983140778018));
#19095=CARTESIAN_POINT('Ctrl Pts',(95.9012810906271,-0.429230043733431,
2.16219158011915));
#19096=CARTESIAN_POINT('Ctrl Pts',(95.9063945699805,-0.527092850754496,
2.14085713156891));
#19097=CARTESIAN_POINT('Ctrl Pts',(95.9093407535116,-0.584206248039353,
2.12598207920902));
#19098=CARTESIAN_POINT('Ctrl Pts',(95.9169361773389,-0.731795172127066,
2.08114503946293));
#19099=CARTESIAN_POINT('Ctrl Pts',(95.9215081523608,-0.821044567312776,
2.04757785988123));
#19100=CARTESIAN_POINT('Ctrl Pts',(95.9274997625985,-0.933767217458664,
1.99662320497921));
#19101=CARTESIAN_POINT('Ctrl Pts',(95.9288813308404,-0.959462567590678,
1.9844034331603));
#19102=CARTESIAN_POINT('Ctrl Pts',(95.9345948085902,-1.06404834285758,1.93215993199128));
#19103=CARTESIAN_POINT('Ctrl Pts',(95.9389961067053,-1.14072385338066,1.88790542542031));
#19104=CARTESIAN_POINT('Ctrl Pts',(95.9444480208715,-1.22714701287942,1.83083450786026));
#19105=CARTESIAN_POINT('Ctrl Pts',(95.9452515965109,-1.23968244628205,1.82236993876386));
#19106=CARTESIAN_POINT('Ctrl Pts',(95.9465148437435,-1.25905057064349,1.80899927914952));
#19107=CARTESIAN_POINT('Ctrl Pts',(95.9469688030385,-1.26594420300091,1.80418180944501));
#19108=CARTESIAN_POINT('Ctrl Pts',(95.9478117333102,-1.27861751833705,1.79521693569682));
#19109=CARTESIAN_POINT('Ctrl Pts',(95.9481999495739,-1.28440489231027,1.79108086708296));
#19110=CARTESIAN_POINT('Ctrl Pts',(95.9491066100489,-1.29780781172753,1.78140382318188));
#19111=CARTESIAN_POINT('Ctrl Pts',(95.9496264523477,-1.30540794408094,1.77584199474724));
#19112=CARTESIAN_POINT('Ctrl Pts',(95.9512981391637,-1.3295888015866,1.75790717326275));
#19113=CARTESIAN_POINT('Ctrl Pts',(95.9524617033262,-1.34603059275926,1.74534970458874));
#19114=CARTESIAN_POINT('Ctrl Pts',(95.9589470349264,-1.43571332049494,1.67483330589692));
#19115=CARTESIAN_POINT('Ctrl Pts',(95.9644994519691,-1.50538450979502,1.61249929258205));
#19116=CARTESIAN_POINT('Ctrl Pts',(95.9802807150614,-1.69001477289618,1.42488983596014));
#19117=CARTESIAN_POINT('Ctrl Pts',(95.9905170917334,-1.794771358605,1.29045441324676));
#19118=CARTESIAN_POINT('Ctrl Pts',(96.0024215117585,-1.90379577757042,1.11120257047076));
#19119=CARTESIAN_POINT('Ctrl Pts',(96.0046548435043,-1.92361006205016,1.07653803296291));
#19120=CARTESIAN_POINT('Ctrl Pts',(96.0077380873227,-1.95004753997535,1.0272232528158));
#19121=CARTESIAN_POINT('Ctrl Pts',(96.0086160212378,-1.95746804891239,1.01301129113437));
#19122=CARTESIAN_POINT('Ctrl Pts',(96.0101361766362,-1.97012612970443,0.988109652339457));
#19123=CARTESIAN_POINT('Ctrl Pts',(96.0107808261438,-1.97543333240648,0.977456295186827));
#19124=CARTESIAN_POINT('Ctrl Pts',(96.0121272015841,-1.98638815493918,0.955012558954213));
#19125=CARTESIAN_POINT('Ctrl Pts',(96.0128282786494,-1.99201770681454,0.943213844126139));
#19126=CARTESIAN_POINT('Ctrl Pts',(96.0145014510036,-2.00526991886247,0.914791222837917));
#19127=CARTESIAN_POINT('Ctrl Pts',(96.0154700332366,-2.01279136540406,0.898121024830673));
#19128=CARTESIAN_POINT('Ctrl Pts',(96.0188564699912,-2.03854251155913,0.839098513972825));
#19129=CARTESIAN_POINT('Ctrl Pts',(96.0212364979097,-2.05565049197974,0.796268377548354));
#19130=CARTESIAN_POINT('Ctrl Pts',(96.0270965374719,-2.09505313372218,0.687867002270776));
#19131=CARTESIAN_POINT('Ctrl Pts',(96.0305255265622,-2.11562543969606,0.621722218277033));
#19132=CARTESIAN_POINT('Ctrl Pts',(96.040354402202,-2.16623990399721,0.427094185954962));
#19133=CARTESIAN_POINT('Ctrl Pts',(96.0466034293222,-2.18790697071944,0.296757947577396));
#19134=CARTESIAN_POINT('Ctrl Pts',(96.0563473765552,-2.20264994410874,0.100705790308834));
#19135=CARTESIAN_POINT('Ctrl Pts',(96.0596238376294,-2.20465730361557,0.0359615739420522));
#19136=CARTESIAN_POINT('Ctrl Pts',(96.0637915706463,-2.20362567794578,-0.0430584218821372));
#19137=CARTESIAN_POINT('Ctrl Pts',(96.0645517356219,-2.20330023253847,-0.0573430045539922));
#19138=CARTESIAN_POINT('Ctrl Pts',(96.0657609964939,-2.20256874633792,-0.0798405720206565));
#19139=CARTESIAN_POINT('Ctrl Pts',(96.0662051346934,-2.20225558529642,-0.0880564128882801));
#19140=CARTESIAN_POINT('Ctrl Pts',(96.0670440285627,-2.20158120712884,-0.103480825864513));
#19141=CARTESIAN_POINT('Ctrl Pts',(96.0674382057513,-2.20123054218426,-0.110689600753901));
#19142=CARTESIAN_POINT('Ctrl Pts',(96.0683705511707,-2.20032190418409,-0.127651698556929));
#19143=CARTESIAN_POINT('Ctrl Pts',(96.0689103133956,-2.1997344827473,-0.137403188475828));
#19144=CARTESIAN_POINT('Ctrl Pts',(96.0707145129141,-2.19756761016867,-0.169785945114205));
#19145=CARTESIAN_POINT('Ctrl Pts',(96.0719933146377,-2.19570361417405,-0.192396011186734));
#19146=CARTESIAN_POINT('Ctrl Pts',(96.0751494655941,-2.19030407636597,-0.247490715104332));
#19147=CARTESIAN_POINT('Ctrl Pts',(96.0770420107452,-2.18639452925789,-0.27993280355363));
#19148=CARTESIAN_POINT('Ctrl Pts',(96.0850848020483,-2.16693521363938,-0.41588904052543));
#19149=CARTESIAN_POINT('Ctrl Pts',(96.0914102969468,-2.14474315292751,-0.518312139079507));
#19150=CARTESIAN_POINT('Ctrl Pts',(96.1058952413664,-2.07694456183987,-0.750092911015594));
#19151=CARTESIAN_POINT('Ctrl Pts',(96.1139762899925,-2.02637978732648,-0.877572031132577));
#19152=CARTESIAN_POINT('Ctrl Pts',(96.1234137563986,-1.95020209235962,-1.02727574259194));
#19153=CARTESIAN_POINT('Ctrl Pts',(96.1251416375877,-1.93550865355848,-1.05469902996348));
#19154=CARTESIAN_POINT('Ctrl Pts',(96.1277232300061,-1.91242170602501,-1.09567918420449));
#19155=CARTESIAN_POINT('Ctrl Pts',(96.1285919526992,-1.90445403989741,-1.10947036241378));
#19156=CARTESIAN_POINT('Ctrl Pts',(96.130145556035,-1.8898478100494,-1.13413113168745));
#19157=CARTESIAN_POINT('Ctrl Pts',(96.1308323533897,-1.8832632545767,-1.14503174299403));
#19158=CARTESIAN_POINT('Ctrl Pts',(96.1322947674607,-1.86897053793888,-1.1682362367599));
#19159=CARTESIAN_POINT('Ctrl Pts',(96.1330693173745,-1.86123450754118,-1.18052229893341));
#19160=CARTESIAN_POINT('Ctrl Pts',(96.1351776295511,-1.83972582079231,-1.21394451122998));
#19161=CARTESIAN_POINT('Ctrl Pts',(96.1365023330773,-1.82571058560372,-1.23492238562563));
#19162=CARTESIAN_POINT('Ctrl Pts',(96.1456196927004,-1.72584096036568,-1.37898866864711));
#19163=CARTESIAN_POINT('Ctrl Pts',(96.1529182045005,-1.62797045813742,-1.49326985766682));
#19164=CARTESIAN_POINT('Ctrl Pts',(96.1668973019706,-1.41845653199072,-1.69261576069878));
#19165=CARTESIAN_POINT('Ctrl Pts',(96.1735656384931,-1.30883669950046,-1.77873683153962));
#19166=CARTESIAN_POINT('Ctrl Pts',(96.1818558632557,-1.17522285060526,-1.86463346195436));
#19167=CARTESIAN_POINT('Ctrl Pts',(96.1828992905372,-1.15845373320334,-1.87509775490868));
#19168=CARTESIAN_POINT('Ctrl Pts',(96.1844512889781,-1.13363570433075,-1.89012476270686));
#19169=CARTESIAN_POINT('Ctrl Pts',(96.1849490231848,-1.12569474982163,-1.89486486397816));
#19170=CARTESIAN_POINT('Ctrl Pts',(96.185838088848,-1.11154951239531,-1.9031881176885));
#19171=CARTESIAN_POINT('Ctrl Pts',(96.1862281328318,-1.105357270884,-1.90679118719994));
#19172=CARTESIAN_POINT('Ctrl Pts',(96.187088608182,-1.09172733147969,-1.91463331154296));
#19173=CARTESIAN_POINT('Ctrl Pts',(96.1875598216945,-1.08428256070421,-1.91885919427631));
#19174=CARTESIAN_POINT('Ctrl Pts',(96.1889344326019,-1.0626135974916,-1.93099280220957));
#19175=CARTESIAN_POINT('Ctrl Pts',(96.1898445889073,-1.04832649274231,-1.93878631944902));
#19176=CARTESIAN_POINT('Ctrl Pts',(96.1919531741744,-1.01532802360984,-1.95631538046725));
#19177=CARTESIAN_POINT('Ctrl Pts',(96.1931570634248,-0.996560749644345,
-1.9659418801496));
#19178=CARTESIAN_POINT('Ctrl Pts',(96.197281655568,-0.932396365078903,-1.99769957127598));
#19179=CARTESIAN_POINT('Ctrl Pts',(96.2002537592485,-0.88637950854176,-2.0185384285643));
#19180=CARTESIAN_POINT('Ctrl Pts',(96.2088773582891,-0.752298370335672,
-2.07378814837831));
#19181=CARTESIAN_POINT('Ctrl Pts',(96.214593284168,-0.662680984395197,-2.1041397484341));
#19182=CARTESIAN_POINT('Ctrl Pts',(96.2279600237636,-0.446629300034757,
-2.16213449407633));
#19183=CARTESIAN_POINT('Ctrl Pts',(96.2355147290957,-0.319149454574453,
-2.18459506137907));
#19184=CARTESIAN_POINT('Ctrl Pts',(96.2440819885446,-0.165969212274163,
-2.19787910195878));
#19185=CARTESIAN_POINT('Ctrl Pts',(96.2454368808827,-0.141484277738279,
-2.19959100611417));
#19186=CARTESIAN_POINT('Ctrl Pts',(96.2475724663737,-0.102485621618808,
-2.20166374280065));
#19187=CARTESIAN_POINT('Ctrl Pts',(96.2483614130916,-0.087988623317635,
-2.2022907517718));
#19188=CARTESIAN_POINT('Ctrl Pts',(96.2498278436583,-0.0608789692863493,
-2.20319515052269));
#19189=CARTESIAN_POINT('Ctrl Pts',(96.2505063936855,-0.0482681430775895,
-2.20350750299152));
#19190=CARTESIAN_POINT('Ctrl Pts',(96.2520314430948,-0.0197791283163416,
-2.20396844350308));
#19191=CARTESIAN_POINT('Ctrl Pts',(96.2528759301563,-0.00390052936315621,
-2.20405374653897));
#19192=CARTESIAN_POINT('Ctrl Pts',(96.2554017270825,0.0438860806456116,
-2.20379404083033));
#19193=CARTESIAN_POINT('Ctrl Pts',(96.2570668024269,0.0757877150087699,
-2.20292771566959));
#19194=CARTESIAN_POINT('Ctrl Pts',(96.2608724208335,0.149494780580092,-2.19932298932911));
#19195=CARTESIAN_POINT('Ctrl Pts',(96.2629980147041,0.191263700756831,-2.196084870073));
#19196=CARTESIAN_POINT('Ctrl Pts',(96.2706937728745,0.344021171097496,-2.17985070030595));
#19197=CARTESIAN_POINT('Ctrl Pts',(96.2760771354235,0.45407090513955,-2.15961125823417));
#19198=CARTESIAN_POINT('Ctrl Pts',(96.2874200957706,0.680940333597782,-2.09977108078821));
#19199=CARTESIAN_POINT('Ctrl Pts',(96.2933659224868,0.79692616242497,-2.05854818734973));
#19200=CARTESIAN_POINT('Ctrl Pts',(96.3008444195426,0.927665345717941,-1.99936968991775));
#19201=CARTESIAN_POINT('Ctrl Pts',(96.3019329185878,0.946350665226227,-1.99059350658646));
#19202=CARTESIAN_POINT('Ctrl Pts',(96.3035342081346,0.973279495494193,-1.97748064379802));
#19203=CARTESIAN_POINT('Ctrl Pts',(96.3040349804591,0.981623649670132,-1.97335188880081));
#19204=CARTESIAN_POINT('Ctrl Pts',(96.3049279156702,0.996358903495227,-1.96594418301159));
#19205=CARTESIAN_POINT('Ctrl Pts',(96.3053187585022,1.00276048425597,-1.96268668031572));
#19206=CARTESIAN_POINT('Ctrl Pts',(96.306171202624,1.01661674971638,-1.9555503053585));
#19207=CARTESIAN_POINT('Ctrl Pts',(96.306633474237,1.02406510020186,-1.95166013392113));
#19208=CARTESIAN_POINT('Ctrl Pts',(96.3079567966919,1.04520746756161,-1.94046341411549));
#19209=CARTESIAN_POINT('Ctrl Pts',(96.3088238816187,1.05884653178706,-1.93305481195917));
#19210=CARTESIAN_POINT('Ctrl Pts',(96.3164216791809,1.17663613228743,-1.86745208267261));
#19211=CARTESIAN_POINT('Ctrl Pts',(96.3235678866878,1.27597173501087,-1.8010388410879));
#19212=CARTESIAN_POINT('Ctrl Pts',(96.3408459085113,1.50134185530338,-1.622322120633));
#19213=CARTESIAN_POINT('Ctrl Pts',(96.3509031747188,1.62085104389143,-1.50293569976867));
#19214=CARTESIAN_POINT('Ctrl Pts',(96.3618694702046,1.74247164399541,-1.3498678633229));
#19215=CARTESIAN_POINT('Ctrl Pts',(96.3633747294411,1.75894098768131,-1.32833631761434));
#19216=CARTESIAN_POINT('Ctrl Pts',(96.365763067906,1.78470144709975,-1.29333833903934));
#19217=CARTESIAN_POINT('Ctrl Pts',(96.366655938807,1.79424675237807,-1.28006325094539));
#19218=CARTESIAN_POINT('Ctrl Pts',(96.3682381492486,1.81100516791609,-1.25620076002369));
#19219=CARTESIAN_POINT('Ctrl Pts',(96.368929654712,1.81827528148879,-1.24565447781577));
#19220=CARTESIAN_POINT('Ctrl Pts',(96.3703754492904,1.83335856899735,-1.22336069177645));
#19221=CARTESIAN_POINT('Ctrl Pts',(96.3711289628327,1.84115173726136,-1.21160031270838));
#19222=CARTESIAN_POINT('Ctrl Pts',(96.3731163048136,1.86151927031364,-1.18021407001997));
#19223=CARTESIAN_POINT('Ctrl Pts',(96.3743427933663,1.87389632399892,-1.16046191943846));
#19224=CARTESIAN_POINT('Ctrl Pts',(96.3807118271914,1.93709054953012,-1.05596396247197));
#19225=CARTESIAN_POINT('Ctrl Pts',(96.3856558484739,1.98248181068108,-0.968064264965195));
#19226=CARTESIAN_POINT('Ctrl Pts',(96.3947783354814,2.05660914507512,-0.79725137336613));
#19227=CARTESIAN_POINT('Ctrl Pts',(96.3989726564833,2.08659704433845,-0.715097128535994));
#19228=CARTESIAN_POINT('Ctrl Pts',(96.4042827625629,2.11798245901127,-0.610129700973389));
#19229=CARTESIAN_POINT('Ctrl Pts',(96.4053603115707,2.12401514866286,-0.58878483374268));
#19230=CARTESIAN_POINT('Ctrl Pts',(96.4108993952927,2.15322794816694,-0.479126040137549));
#19231=CARTESIAN_POINT('Ctrl Pts',(96.4154334085284,2.1712239630383,-0.389532450254598));
#19232=CARTESIAN_POINT('Ctrl Pts',(96.4210374799336,2.1856724516899,-0.284046696415114));
#19233=CARTESIAN_POINT('Ctrl Pts',(96.4218441409211,2.18757755379661,-0.268981435426561));
#19234=CARTESIAN_POINT('Ctrl Pts',(96.4231112213859,2.19029715312867,-0.245530722723418));
#19235=CARTESIAN_POINT('Ctrl Pts',(96.4235658731679,2.1912195330178,-0.237157981412252));
#19236=CARTESIAN_POINT('Ctrl Pts',(96.4244130951769,2.19283919325712,-0.221638955970571));
#19237=CARTESIAN_POINT('Ctrl Pts',(96.4248049390325,2.19354957510567,-0.214494314918458));
#19238=CARTESIAN_POINT('Ctrl Pts',(96.4257164324376,2.19511300854282,-0.197949414526301));
#19239=CARTESIAN_POINT('Ctrl Pts',(96.4262374581256,2.19594059506856,-0.188547042465269));
#19240=CARTESIAN_POINT('Ctrl Pts',(96.4279168218778,2.19839865825663,-0.158404964924212));
#19241=CARTESIAN_POINT('Ctrl Pts',(96.4290870254262,2.19979584702298,-0.137647959640263));
#19242=CARTESIAN_POINT('Ctrl Pts',(96.4356458951889,2.20591318850858,-0.0224510290842082));
#19243=CARTESIAN_POINT('Ctrl Pts',(96.4412705508507,2.20484526854382,0.0721905304386301));
#19244=CARTESIAN_POINT('Ctrl Pts',(96.4573366679125,2.18461053880717,0.3393380691337));
#19245=CARTESIAN_POINT('Ctrl Pts',(96.4677768184736,2.15116111459607,0.51009491960279));
#19246=CARTESIAN_POINT('Ctrl Pts',(96.4796737715376,2.08671260616069,0.710360818463461));
#19247=CARTESIAN_POINT('Ctrl Pts',(96.4817362991761,2.07450677878628,0.745254218678266));
#19248=CARTESIAN_POINT('Ctrl Pts',(96.4846993030599,2.05545316494838,0.795621454311846));
#19249=CARTESIAN_POINT('Ctrl Pts',(96.4856224584723,2.04929625877823,0.811348308700729));
#19250=CARTESIAN_POINT('Ctrl Pts',(96.4872393375641,2.03812348585534,0.838948587555738));
#19251=CARTESIAN_POINT('Ctrl Pts',(96.4879355638596,2.03318315266614,0.850851546235838));
#19252=CARTESIAN_POINT('Ctrl Pts',(96.4893729656495,2.02271547909453,0.875459904383508));
#19253=CARTESIAN_POINT('Ctrl Pts',(96.4901135593119,2.01717215135409,0.888157912412327));
#19254=CARTESIAN_POINT('Ctrl Pts',(96.4920265722969,2.00246491876485,0.920999428082396));
#19255=CARTESIAN_POINT('Ctrl Pts',(96.4931926345052,1.99311660638524,0.941058944934252));
#19256=CARTESIAN_POINT('Ctrl Pts',(96.4985922015641,1.94805562063296,1.03406555191182));
#19257=CARTESIAN_POINT('Ctrl Pts',(96.5026956439856,1.90862895577387,1.10514684782467));
#19258=CARTESIAN_POINT('Ctrl Pts',(96.5156576513813,1.76903981148894,1.32695949385321));
#19259=CARTESIAN_POINT('Ctrl Pts',(96.5240772148112,1.65425205797801,1.46757065035644));
#19260=CARTESIAN_POINT('Ctrl Pts',(96.5354440708961,1.4914669418121,1.62330492191023));
#19261=CARTESIAN_POINT('Ctrl Pts',(96.5377303964993,1.45842186891647,1.65305706402045));
#19262=CARTESIAN_POINT('Ctrl Pts',(96.5407682284135,1.41462075458636,1.69015733325009));
#19263=CARTESIAN_POINT('Ctrl Pts',(96.5414591065936,1.40466612875451,1.69843950172202));
#19264=CARTESIAN_POINT('Ctrl Pts',(96.5425784908134,1.38856340245142,1.71159844806368));
#19265=CARTESIAN_POINT('Ctrl Pts',(96.5430031055143,1.38246108896063,1.71653106689915));
#19266=CARTESIAN_POINT('Ctrl Pts',(96.543830360968,1.37058773378974,1.72602414988892));
#19267=CARTESIAN_POINT('Ctrl Pts',(96.5442327249973,1.364820018347,1.73058845884856));
#19268=CARTESIAN_POINT('Ctrl Pts',(96.5452212693439,1.35066447658931,1.7416757383585));
#19269=CARTESIAN_POINT('Ctrl Pts',(96.5458096101251,1.34225216010275,1.74816705014371));
#19270=CARTESIAN_POINT('Ctrl Pts',(96.5479704986416,1.31138541587505,1.77163104600969));
#19271=CARTESIAN_POINT('Ctrl Pts',(96.5495658966372,1.28865420153447,1.78823333785824));
#19272=CARTESIAN_POINT('Ctrl Pts',(96.5537087194223,1.22958715755054,1.82966328312686));
#19273=CARTESIAN_POINT('Ctrl Pts',(96.556285058024,1.19281498195989,1.85384582252322));
#19274=CARTESIAN_POINT('Ctrl Pts',(96.5655614583133,1.05936529084845,1.93599174657397));
#19275=CARTESIAN_POINT('Ctrl Pts',(96.5723961032028,0.958995110198635,1.98762356678948));
#19276=CARTESIAN_POINT('Ctrl Pts',(96.5847689810228,0.767726715869882,2.06813971887748));
#19277=CARTESIAN_POINT('Ctrl Pts',(96.5903298254906,0.678047697994684,2.09925241391017));
#19278=CARTESIAN_POINT('Ctrl Pts',(96.5980266060704,0.547395846853923,2.13532922936114));
#19279=CARTESIAN_POINT('Ctrl Pts',(96.6003053630503,0.507862131127759,2.14507563875295));
#19280=CARTESIAN_POINT('Ctrl Pts',(96.6034400782898,0.452286697971418,2.15715412658319));
#19281=CARTESIAN_POINT('Ctrl Pts',(96.6043252964105,0.436456653689497,2.16041264394223));
#19282=CARTESIAN_POINT('Ctrl Pts',(96.6058544683153,0.408878107883364,2.16577401668957));
#19283=CARTESIAN_POINT('Ctrl Pts',(96.6065009223488,0.397145862726018,2.16795608120854));
#19284=CARTESIAN_POINT('Ctrl Pts',(96.6078476670213,0.372553150141126,2.17232370969069));
#19285=CARTESIAN_POINT('Ctrl Pts',(96.6085473404807,0.359689810180622,2.17449060699851));
#19286=CARTESIAN_POINT('Ctrl Pts',(96.6099331970021,0.334042858564615,2.17857716164128));
#19287=CARTESIAN_POINT('Ctrl Pts',(96.6106194172299,0.321260097474045,2.18049880531059));
#19288=CARTESIAN_POINT('Ctrl Pts',(96.6122266909798,0.29113005146125,2.18475757354844));
#19289=CARTESIAN_POINT('Ctrl Pts',(96.6131448003547,0.273770243327787,2.18700074047738));
#19290=CARTESIAN_POINT('Ctrl Pts',(96.6185207744709,0.171291457976957,2.19900330011054));
#19291=CARTESIAN_POINT('Ctrl Pts',(96.6228297409556,0.0856854896088731,
2.20399999999897));
#19292=CARTESIAN_POINT('Ctrl Pts',(96.6270503826334,2.66056133811156E-11,
2.204));
#19293=CARTESIAN_POINT('Origin',(66.9212607628943,0.,0.));
#19294=CARTESIAN_POINT('',(97.4861833980632,-2.69730385036004E-13,2.204));
#19295=CARTESIAN_POINT('',(97.3739726165667,2.84962952926334E-13,2.204));
#19296=CARTESIAN_POINT('',(66.9212607628943,-2.69912154532077E-16,2.204));
#19297=CARTESIAN_POINT('',(96.7329774739213,-0.00170103368875552,2.20399915589494));
#19298=CARTESIAN_POINT('Ctrl Pts',(97.4861833980632,7.30595079061364E-14,
2.204));
#19299=CARTESIAN_POINT('Ctrl Pts',(97.4843902495947,0.0314723260755802,
2.204));
#19300=CARTESIAN_POINT('Ctrl Pts',(97.4825693510585,0.0629397455639223,
2.20332587853465));
#19301=CARTESIAN_POINT('Ctrl Pts',(97.4749354119193,0.193342401425828,2.19773659949954));
#19302=CARTESIAN_POINT('Ctrl Pts',(97.4689606176528,0.29190213610691,2.18682858080225));
#19303=CARTESIAN_POINT('Ctrl Pts',(97.454325322464,0.531846115290877,2.14375915178902));
#19304=CARTESIAN_POINT('Ctrl Pts',(97.4457527927398,0.67145579133593,2.10421529188373));
#19305=CARTESIAN_POINT('Ctrl Pts',(97.4358871645072,0.834927485476195,2.03996695847093));
#19306=CARTESIAN_POINT('Ctrl Pts',(97.43417271346,0.863420783249822,2.02807144476291));
#19307=CARTESIAN_POINT('Ctrl Pts',(97.4316120951221,0.906092089037131,2.00919444487641));
#19308=CARTESIAN_POINT('Ctrl Pts',(97.4307511257505,0.920459582804573,2.00265308175134));
#19309=CARTESIAN_POINT('Ctrl Pts',(97.4292120460474,0.946173980405307,1.99061040077821));
#19310=CARTESIAN_POINT('Ctrl Pts',(97.4285320450407,0.957546196822834,1.98516504579467));
#19311=CARTESIAN_POINT('Ctrl Pts',(97.4270849736607,0.981766270993176,1.9733112024035));
#19312=CARTESIAN_POINT('Ctrl Pts',(97.4263189379402,0.9945995425514,1.96687413823958));
#19313=CARTESIAN_POINT('Ctrl Pts',(97.424236575634,1.02950810950492,1.94893525144942));
#19314=CARTESIAN_POINT('Ctrl Pts',(97.4229290503544,1.05145324510039,1.93718396170564));
#19315=CARTESIAN_POINT('Ctrl Pts',(97.4136162113215,1.20777735362995,1.8500355021328));
#19316=CARTESIAN_POINT('Ctrl Pts',(97.4061362544506,1.3341230688445,1.76110170541595));
#19317=CARTESIAN_POINT('Ctrl Pts',(97.3921506410449,1.55202939370889,1.57070603299438));
#19318=CARTESIAN_POINT('Ctrl Pts',(97.3856525328407,1.64546921381575,1.47252692960714));
#19319=CARTESIAN_POINT('Ctrl Pts',(97.3776536859106,1.74053188733054,1.35221755567726));
#19320=CARTESIAN_POINT('Ctrl Pts',(97.3766996672777,1.75157697973595,1.33787952076132));
#19321=CARTESIAN_POINT('Ctrl Pts',(97.3752531158359,1.76785893318571,1.31619607968734));
#19322=CARTESIAN_POINT('Ctrl Pts',(97.3747691965829,1.7732295661026,1.30895157590678));
#19323=CARTESIAN_POINT('Ctrl Pts',(97.3738906425274,1.78283878667285,1.29582192422749));
#19324=CARTESIAN_POINT('Ctrl Pts',(97.3734970762231,1.78709313028584,1.28994834814982));
#19325=CARTESIAN_POINT('Ctrl Pts',(97.3726832838348,1.79578458564452,1.27782334024569));
#19326=CARTESIAN_POINT('Ctrl Pts',(97.372262845165,1.80021817800254,1.27156961068004));
#19327=CARTESIAN_POINT('Ctrl Pts',(97.3711593349858,1.81171037773796,1.25517890735915));
#19328=CARTESIAN_POINT('Ctrl Pts',(97.3704728686715,1.81871645182566,1.24500563680229));
#19329=CARTESIAN_POINT('Ctrl Pts',(97.3673409686397,1.85005898052567,1.19866513108422));
#19330=CARTESIAN_POINT('Ctrl Pts',(97.3648388381958,1.87340326183103,1.16184166105117));
#19331=CARTESIAN_POINT('Ctrl Pts',(97.3572567817081,1.9397248383195,1.05002467342151));
#19332=CARTESIAN_POINT('Ctrl Pts',(97.3520687270945,1.97939913373605,0.97317110919485));
#19333=CARTESIAN_POINT('Ctrl Pts',(97.3370987627309,2.08049131205197,0.745427948223738));
#19334=CARTESIAN_POINT('Ctrl Pts',(97.3273946107137,2.12985372372918,0.589784547703335));
#19335=CARTESIAN_POINT('Ctrl Pts',(97.31671785903,2.16698234211206,0.403183626600176));
#19336=CARTESIAN_POINT('Ctrl Pts',(97.3151929465046,2.17183590057099,0.376162763433086));
#19337=CARTESIAN_POINT('Ctrl Pts',(97.3127844093818,2.17877516558641,0.332900208248145));
#19338=CARTESIAN_POINT('Ctrl Pts',(97.3118906083612,2.18118678657203,0.316714371787064));
#19339=CARTESIAN_POINT('Ctrl Pts',(97.3103129998369,2.18515019370017,0.28791672815055));
#19340=CARTESIAN_POINT('Ctrl Pts',(97.3096269596416,2.18677358248112,0.275315672966913));
#19341=CARTESIAN_POINT('Ctrl Pts',(97.3081989327879,2.18994160626818,0.24892618186986));
#19342=CARTESIAN_POINT('Ctrl Pts',(97.3074576378885,2.19146518876689,0.235135750947186));
#19343=CARTESIAN_POINT('Ctrl Pts',(97.3055173658842,2.19513191861933,0.198807370926436));
#19344=CARTESIAN_POINT('Ctrl Pts',(97.3043252161215,2.19705823481799,0.176248897831331));
#19345=CARTESIAN_POINT('Ctrl Pts',(97.2984351380006,2.20492470471471,0.0636949522456942));
#19346=CARTESIAN_POINT('Ctrl Pts',(97.2939004399123,2.20568488556786,-0.026580008133357));
#19347=CARTESIAN_POINT('Ctrl Pts',(97.284847899904,2.19594817388748,-0.210280821575465));
#19348=CARTESIAN_POINT('Ctrl Pts',(97.2803469483846,2.18501646612491,-0.30349604135809));
#19349=CARTESIAN_POINT('Ctrl Pts',(97.2744798042756,2.16326590799182,-0.422665610385005));
#19350=CARTESIAN_POINT('Ctrl Pts',(97.2731504641328,2.15784857329439,-0.449505407251845));
#19351=CARTESIAN_POINT('Ctrl Pts',(97.2674275094161,2.13253171080127,-0.563902613953819));
#19352=CARTESIAN_POINT('Ctrl Pts',(97.2629636402508,2.10779366050144,-0.650292505246297));
#19353=CARTESIAN_POINT('Ctrl Pts',(97.2574446139191,2.07283845353986,-0.749121852516237));
#19354=CARTESIAN_POINT('Ctrl Pts',(97.2566444572458,2.0676714322159,-0.763267730248926));
#19355=CARTESIAN_POINT('Ctrl Pts',(97.2553881280853,2.05941634871663,-0.785168744517474));
#19356=CARTESIAN_POINT('Ctrl Pts',(97.2549376362427,2.05642841745628,-0.792961420220219));
#19357=CARTESIAN_POINT('Ctrl Pts',(97.2540986803974,2.05081487137384,-0.807356705823696));
#19358=CARTESIAN_POINT('Ctrl Pts',(97.2537109344989,2.0482015056176,-0.813963804443493));
#19359=CARTESIAN_POINT('Ctrl Pts',(97.2528101252096,2.04208622480996,-0.82920849017591));
#19360=CARTESIAN_POINT('Ctrl Pts',(97.2522957276487,2.03856143169631,-0.83783659056455));
#19361=CARTESIAN_POINT('Ctrl Pts',(97.2506426944887,2.02712632023857,-0.865328432133981));
#19362=CARTESIAN_POINT('Ctrl Pts',(97.2494925938245,2.01900829091629,-0.884103994845832));
#19363=CARTESIAN_POINT('Ctrl Pts',(97.2431087330273,1.97299224880633,-0.986590737798431));
#19364=CARTESIAN_POINT('Ctrl Pts',(97.2376507820627,1.93015138320509,-1.06797591797514));
#19365=CARTESIAN_POINT('Ctrl Pts',(97.2222497152123,1.79648599541898,-1.28744310928803));
#19366=CARTESIAN_POINT('Ctrl Pts',(97.2122882202069,1.69502612089247,-1.41836947935311));
#19367=CARTESIAN_POINT('Ctrl Pts',(97.2003226737584,1.54864880413619,-1.56885624138146));
#19368=CARTESIAN_POINT('Ctrl Pts',(97.197808430062,1.51643873872145,-1.60001155831753));
#19369=CARTESIAN_POINT('Ctrl Pts',(97.1943177112892,1.46964547271655,-1.64258910782558));
#19370=CARTESIAN_POINT('Ctrl Pts',(97.1933063696388,1.45583547398155,-1.65484135028619));
#19371=CARTESIAN_POINT('Ctrl Pts',(97.1916018293131,1.43213282904504,-1.67534396762353));
#19372=CARTESIAN_POINT('Ctrl Pts',(97.1909049442883,1.42231899901421,-1.68368361778125));
#19373=CARTESIAN_POINT('Ctrl Pts',(97.1894992233151,1.40227517390827,-1.70041624521519));
#19374=CARTESIAN_POINT('Ctrl Pts',(97.1887906123723,1.39204156156876,-1.70880407646227));
#19375=CARTESIAN_POINT('Ctrl Pts',(97.1870416364104,1.36646519368071,-1.72938512669559));
#19376=CARTESIAN_POINT('Ctrl Pts',(97.1860057473891,1.35103401675011,-1.74146695650532));
#19377=CARTESIAN_POINT('Ctrl Pts',(97.1820021835804,1.29032096800083,-1.78770942244571));
#19378=CARTESIAN_POINT('Ctrl Pts',(97.1790943708904,1.24388663194669,-1.82032412337711));
#19379=CARTESIAN_POINT('Ctrl Pts',(97.171457942478,1.11647080736586,-1.90266393335233));
#19380=CARTESIAN_POINT('Ctrl Pts',(97.1668356300204,1.0334466483486,-1.94900657013373));
#19381=CARTESIAN_POINT('Ctrl Pts',(97.1549936267287,0.812442913708665,-2.05426212987753));
#19382=CARTESIAN_POINT('Ctrl Pts',(97.1478555279512,0.670998777512727,-2.10471048877184));
#19383=CARTESIAN_POINT('Ctrl Pts',(97.1390379246194,0.507175503059395,-2.14493522842281));
#19384=CARTESIAN_POINT('Ctrl Pts',(97.1380377905056,0.4887404530414,-2.14921074983252));
#19385=CARTESIAN_POINT('Ctrl Pts',(97.1365412858173,0.461425898567661,-2.15517604359062));
#19386=CARTESIAN_POINT('Ctrl Pts',(97.136054764761,0.45258692827555,-2.15704953704731));
#19387=CARTESIAN_POINT('Ctrl Pts',(97.1351812347445,0.436797071893396,-2.16029500603582));
#19388=CARTESIAN_POINT('Ctrl Pts',(97.1347954099061,0.429850762167566,-2.16168788570218));
#19389=CARTESIAN_POINT('Ctrl Pts',(97.1339390981143,0.414496263369222,-2.16468984612883));
#19390=CARTESIAN_POINT('Ctrl Pts',(97.1334677839886,0.406085465510928,-2.16628342372901));
#19391=CARTESIAN_POINT('Ctrl Pts',(97.132079139233,0.381414181903443,-2.17080911702656));
#19392=CARTESIAN_POINT('Ctrl Pts',(97.1311547720636,0.365130098671784,-2.17360736529565));
#19393=CARTESIAN_POINT('Ctrl Pts',(97.1237607453317,0.235814081372858,-2.19433483245255));
#19394=CARTESIAN_POINT('Ctrl Pts',(97.1169153173528,0.12158207932078,-2.20361675603818));
#19395=CARTESIAN_POINT('Ctrl Pts',(97.0996910426312,-0.165204304117157,
-2.204548165254));
#19396=CARTESIAN_POINT('Ctrl Pts',(97.0893811162678,-0.337067250979015,
-2.18488659251315));
#19397=CARTESIAN_POINT('Ctrl Pts',(97.0782215230451,-0.530844126399516,
-2.13928280460057));
#19398=CARTESIAN_POINT('Ctrl Pts',(97.0767420311437,-0.556676601624274,
-2.13270664967745));
#19399=CARTESIAN_POINT('Ctrl Pts',(97.0743812852405,-0.598116721889119,
-2.1213529824741));
#19400=CARTESIAN_POINT('Ctrl Pts',(97.0734907216844,-0.613801128296913,
-2.11686803659208));
#19401=CARTESIAN_POINT('Ctrl Pts',(97.0719189369909,-0.641569560307601,
-2.10859309335856));
#19402=CARTESIAN_POINT('Ctrl Pts',(97.0712354956868,-0.653673300649765,
-2.10487233803667));
#19403=CARTESIAN_POINT('Ctrl Pts',(97.0698014477056,-0.679128519827647,
-2.09680651736959));
#19404=CARTESIAN_POINT('Ctrl Pts',(97.0690516546659,-0.692471932264333,
-2.09243775373208));
#19405=CARTESIAN_POINT('Ctrl Pts',(97.0670626270685,-0.727951297086907,
-2.08044490251017));
#19406=CARTESIAN_POINT('Ctrl Pts',(97.0658308738873,-0.750009361629385,
-2.07259501500504));
#19407=CARTESIAN_POINT('Ctrl Pts',(97.0592162345691,-0.86882727410245,-2.02816545960972));
#19408=CARTESIAN_POINT('Ctrl Pts',(97.0540527908047,-0.963049890183291,
-1.98515844605545));
#19409=CARTESIAN_POINT('Ctrl Pts',(97.0421462615306,-1.17691867928918,-1.86871469878127));
#19410=CARTESIAN_POINT('Ctrl Pts',(97.0355255214351,-1.29325484426941,-1.79017330698028));
#19411=CARTESIAN_POINT('Ctrl Pts',(97.025640897626,-1.4464206216406,-1.6639993180996));
#19412=CARTESIAN_POINT('Ctrl Pts',(97.0226711478744,-1.48999761786776,-1.62509458126694));
#19413=CARTESIAN_POINT('Ctrl Pts',(97.0188499845982,-1.54203549182178,-1.57478200638507));
#19414=CARTESIAN_POINT('Ctrl Pts',(97.0181048472828,-1.55200282918893,-1.56495975146903));
#19415=CARTESIAN_POINT('Ctrl Pts',(97.0169211398444,-1.56753818592971,-1.54935613902266));
#19416=CARTESIAN_POINT('Ctrl Pts',(97.0164873571561,-1.57316947394977,-1.54363797956024));
#19417=CARTESIAN_POINT('Ctrl Pts',(97.0156611581329,-1.58377475884756,-1.53275078596568));
#19418=CARTESIAN_POINT('Ctrl Pts',(97.0152692240696,-1.58875490101081,-1.52758807200213));
#19419=CARTESIAN_POINT('Ctrl Pts',(97.0143331121053,-1.60053126483617,-1.51526010963161));
#19420=CARTESIAN_POINT('Ctrl Pts',(97.013787237835,-1.60730464945964,-1.50807336882887));
#19421=CARTESIAN_POINT('Ctrl Pts',(97.011921630882,-1.63014696792455,-1.48350836770117));
#19422=CARTESIAN_POINT('Ctrl Pts',(97.0105860971985,-1.64598365414263,-1.46591743693378));
#19423=CARTESIAN_POINT('Ctrl Pts',(97.0072542851199,-1.68432873688188,-1.42191998914543));
#19424=CARTESIAN_POINT('Ctrl Pts',(97.0052405753113,-1.7065023690532,-1.39523087466689));
#19425=CARTESIAN_POINT('Ctrl Pts',(96.9962662902311,-1.8014176255517,-1.27533814017816));
#19426=CARTESIAN_POINT('Ctrl Pts',(96.9890946346091,-1.86722085702178,-1.17689352755256));
#19427=CARTESIAN_POINT('Ctrl Pts',(96.9741668754745,-1.98885785406354,-0.958825723636734));
#19428=CARTESIAN_POINT('Ctrl Pts',(96.9664720159661,-2.04251020879749,-0.838488811851101));
#19429=CARTESIAN_POINT('Ctrl Pts',(96.9577872296081,-2.09301853508694,-0.691002142353862));
#19430=CARTESIAN_POINT('Ctrl Pts',(96.9564413074771,-2.1005353192608,-0.66780385514399));
#19431=CARTESIAN_POINT('Ctrl Pts',(96.9543213976161,-2.11187238155074,-0.63072814141938));
#19432=CARTESIAN_POINT('Ctrl Pts',(96.9535392432522,-2.115944230563,-0.616930280738423));
#19433=CARTESIAN_POINT('Ctrl Pts',(96.9520865245355,-2.12329703367339,-0.59108508282144));
#19434=CARTESIAN_POINT('Ctrl Pts',(96.9514149004651,-2.12661125467023,-0.579047881231763));
#19435=CARTESIAN_POINT('Ctrl Pts',(96.949907010506,-2.13385775329934,-0.551827029625656));
#19436=CARTESIAN_POINT('Ctrl Pts',(96.9490726946477,-2.13773061909298,-0.536628176097042));
#19437=CARTESIAN_POINT('Ctrl Pts',(96.9465838312718,-2.14886712830983,-0.490888474847003));
#19438=CARTESIAN_POINT('Ctrl Pts',(96.9449449579582,-2.1556410191943,-0.46023185000507));
#19439=CARTESIAN_POINT('Ctrl Pts',(96.9412043435341,-2.16976503490574,-0.389132957326647));
#19440=CARTESIAN_POINT('Ctrl Pts',(96.9391169142962,-2.17664352550493,-0.348608626618659));
#19441=CARTESIAN_POINT('Ctrl Pts',(96.9316231066508,-2.19752021254047,-0.200642120853897));
#19442=CARTESIAN_POINT('Ctrl Pts',(96.9263927060389,-2.2047260212634,-0.0923963498250632));
#19443=CARTESIAN_POINT('Ctrl Pts',(96.9149491386593,-2.20301337828792,0.144365336625957));
#19444=CARTESIAN_POINT('Ctrl Pts',(96.9087549236805,-2.19086155438656,0.272447760188528));
#19445=CARTESIAN_POINT('Ctrl Pts',(96.9009999229888,-2.16395445665159,0.418724895336054));
#19446=CARTESIAN_POINT('Ctrl Pts',(96.8999273359669,-2.15999958350712,0.438669772878307));
#19447=CARTESIAN_POINT('Ctrl Pts',(96.8983481789791,-2.15385548233814,0.46755447876192));
#19448=CARTESIAN_POINT('Ctrl Pts',(96.8978532630552,-2.15188519948143,0.476540356693368));
#19449=CARTESIAN_POINT('Ctrl Pts',(96.8969702426759,-2.14829278082196,0.492447624207584));
#19450=CARTESIAN_POINT('Ctrl Pts',(96.896583421801,-2.14669333460649,0.4993738684383));
#19451=CARTESIAN_POINT('Ctrl Pts',(96.8957395105099,-2.14314878268371,0.514391429695719));
#19452=CARTESIAN_POINT('Ctrl Pts',(96.8952817597846,-2.14119138197548,0.522479385957936));
#19453=CARTESIAN_POINT('Ctrl Pts',(96.8939712565482,-2.13548737806627,0.545477787444204));
#19454=CARTESIAN_POINT('Ctrl Pts',(96.8931125783017,-2.13163057194366,0.560360095056632));
#19455=CARTESIAN_POINT('Ctrl Pts',(96.8857937074348,-2.09772639900901,0.685768814422898));
#19456=CARTESIAN_POINT('Ctrl Pts',(96.8789488925895,-2.05926333488053,0.793829090874947));
#19457=CARTESIAN_POINT('Ctrl Pts',(96.8615781791956,-1.94135202668963,1.05797236852256));
#19458=CARTESIAN_POINT('Ctrl Pts',(96.8511180712936,-1.85138214638012,1.20853500191345));
#19459=CARTESIAN_POINT('Ctrl Pts',(96.8398459112401,-1.72845073171139,1.3677604339701));
#19460=CARTESIAN_POINT('Ctrl Pts',(96.8383834749853,-1.71197201899801,1.38833080630519));
#19461=CARTESIAN_POINT('Ctrl Pts',(96.836044389006,-1.68475791676177,1.42108058475099));
#19462=CARTESIAN_POINT('Ctrl Pts',(96.8351587018626,-1.67425034717578,1.43344517205792));
#19463=CARTESIAN_POINT('Ctrl Pts',(96.8335923690952,-1.65530791671741,1.45524285891229));
#19464=CARTESIAN_POINT('Ctrl Pts',(96.8329095577253,-1.64692664539698,1.46472137676814));
#19465=CARTESIAN_POINT('Ctrl Pts',(96.8315109868719,-1.62950665573687,1.48408335917156));
#19466=CARTESIAN_POINT('Ctrl Pts',(96.8307956659667,-1.62045852628863,1.49395767459595));
#19467=CARTESIAN_POINT('Ctrl Pts',(96.8289102063897,-1.59624614406658,1.51990210682352));
#19468=CARTESIAN_POINT('Ctrl Pts',(96.8277466493144,-1.58092908860251,1.53582792992859));
#19469=CARTESIAN_POINT('Ctrl Pts',(96.8251969752012,-1.54655618885523,1.57050774755632));
#19470=CARTESIAN_POINT('Ctrl Pts',(96.8238156283288,-1.52739326353589,1.58915088181764));
#19471=CARTESIAN_POINT('Ctrl Pts',(96.819655796705,-1.46811351932416,1.64475953931745));
#19472=CARTESIAN_POINT('Ctrl Pts',(96.8169208210087,-1.42695850217705,1.68058953576053));
#19473=CARTESIAN_POINT('Ctrl Pts',(96.807027457737,-1.27125284246115,1.80630074056778));
#19474=CARTESIAN_POINT('Ctrl Pts',(96.80015139719,-1.14921571393859,1.8862946513986));
#19475=CARTESIAN_POINT('Ctrl Pts',(96.789285822506,-0.953514715746994,1.98848759794431));
#19476=CARTESIAN_POINT('Ctrl Pts',(96.7855087122296,-0.885110091611861,
2.01986418848735));
#19477=CARTESIAN_POINT('Ctrl Pts',(96.7807700852478,-0.801544905065273,
2.05313397816844));
#19478=CARTESIAN_POINT('Ctrl Pts',(96.7799863413842,-0.787793198429323,
2.05844971285503));
#19479=CARTESIAN_POINT('Ctrl Pts',(96.7787504074862,-0.766241425292141,
2.06653297989104));
#19480=CARTESIAN_POINT('Ctrl Pts',(96.7783036083793,-0.75847710412266,2.06939531187093));
#19481=CARTESIAN_POINT('Ctrl Pts',(96.7775065015081,-0.744677819527043,
2.07439435261396));
#19482=CARTESIAN_POINT('Ctrl Pts',(96.7771572354373,-0.73864942056618,2.07654858246399));
#19483=CARTESIAN_POINT('Ctrl Pts',(96.776312246932,-0.724107193986955,2.08167386562238));
#19484=CARTESIAN_POINT('Ctrl Pts',(96.7758150313979,-0.715584498214399,
2.08461894149664));
#19485=CARTESIAN_POINT('Ctrl Pts',(96.7742707294686,-0.689210140576254,
2.09355198637103));
#19486=CARTESIAN_POINT('Ctrl Pts',(96.7732141265929,-0.671300079510141,
2.09936340170609));
#19487=CARTESIAN_POINT('Ctrl Pts',(96.7677908761509,-0.579917841186144,
2.12772600150341));
#19488=CARTESIAN_POINT('Ctrl Pts',(96.7632639579809,-0.50538159200088,2.14665091485491));
#19489=CARTESIAN_POINT('Ctrl Pts',(96.7500988493336,-0.288979019454966,
2.18969993523615));
#19490=CARTESIAN_POINT('Ctrl Pts',(96.7413697229979,-0.145521252649599,
2.20388829904848));
#19491=CARTESIAN_POINT('Ctrl Pts',(96.7329771885798,-0.00170172224861046,
2.20399934304468));
#19492=CARTESIAN_POINT('Ctrl Pts',(96.7329771495123,-0.00170105276327685,
2.20399934356149));
#19493=CARTESIAN_POINT('Ctrl Pts',(96.7329440613314,-0.00113403367530617,
2.20399978118839));
#19494=CARTESIAN_POINT('Ctrl Pts',(96.7329109782893,-0.000567016049827459,
2.204));
#19495=CARTESIAN_POINT('Ctrl Pts',(96.7328779004031,-1.24027783152639E-11,
2.204));
#19496=CARTESIAN_POINT('',(96.6271339259349,-0.00170191538198742,2.20399918312151));
#19497=CARTESIAN_POINT('Ctrl Pts',(96.6270503826334,2.66056133811156E-11,
2.204));
#19498=CARTESIAN_POINT('Ctrl Pts',(96.6270783363781,-0.000567503799259821,
2.20400000000001));
#19499=CARTESIAN_POINT('Ctrl Pts',(96.6271062864288,-0.00113501110448395,
2.20399978081177));
#19500=CARTESIAN_POINT('Ctrl Pts',(96.627134232812,-0.00170252176299227,
2.20399934242723));
#19501=CARTESIAN_POINT('Ctrl Pts',(96.6271342022874,-0.00170190189588519,
2.20399934290597));
#19502=CARTESIAN_POINT('Ctrl Pts',(96.632608601421,-0.112871190563222,2.2039134993127));
#19503=CARTESIAN_POINT('Ctrl Pts',(96.6379179252564,-0.223874109134158,
2.19541691506186));
#19504=CARTESIAN_POINT('Ctrl Pts',(96.6478313048556,-0.425361057701924,
2.16454869528108));
#19505=CARTESIAN_POINT('Ctrl Pts',(96.6523990936831,-0.515974735017222,
2.14475406912885));
#19506=CARTESIAN_POINT('Ctrl Pts',(96.6583017855094,-0.624887365886604,
2.11365956383491));
#19507=CARTESIAN_POINT('Ctrl Pts',(96.6593888179286,-0.644629080381249,
2.10772252923118));
#19508=CARTESIAN_POINT('Ctrl Pts',(96.6609936748519,-0.673251137647653,
2.09867514198364));
#19509=CARTESIAN_POINT('Ctrl Pts',(96.6614995840245,-0.682199976442728,
2.0957832978501));
#19510=CARTESIAN_POINT('Ctrl Pts',(96.6623974544973,-0.697944776315688,
2.09058379336497));
#19511=CARTESIAN_POINT('Ctrl Pts',(96.6627880254367,-0.70474836211065,2.08830008677232));
#19512=CARTESIAN_POINT('Ctrl Pts',(96.6636426490523,-0.719535401113837,
2.0832561426042));
#19513=CARTESIAN_POINT('Ctrl Pts',(96.6641074033534,-0.727514065034906,
2.08048326824711));
#19514=CARTESIAN_POINT('Ctrl Pts',(96.6654206156671,-0.74989035794726,2.07256224181435));
#19515=CARTESIAN_POINT('Ctrl Pts',(96.6662748224616,-0.764250368225651,
2.06731012264312));
#19516=CARTESIAN_POINT('Ctrl Pts',(96.6730866049203,-0.877346079311855,
2.02460643001447));
#19517=CARTESIAN_POINT('Ctrl Pts',(96.6793714753231,-0.97332057428682,1.980255095452));
#19518=CARTESIAN_POINT('Ctrl Pts',(96.6926802781187,-1.16750519081809,1.87298291856154));
#19519=CARTESIAN_POINT('Ctrl Pts',(96.6996897043096,-1.26467249081611,1.80879521967758));
#19520=CARTESIAN_POINT('Ctrl Pts',(96.7096058907678,-1.39831625982184,1.70445464433301));
#19521=CARTESIAN_POINT('Ctrl Pts',(96.7126768165444,-1.43910667999149,1.67015765274309));
#19522=CARTESIAN_POINT('Ctrl Pts',(96.7178409275878,-1.50677264015792,1.60894183232749));
#19523=CARTESIAN_POINT('Ctrl Pts',(96.7199607877324,-1.53426705887712,1.58274522680123));
#19524=CARTESIAN_POINT('Ctrl Pts',(96.7228958098586,-1.57191868049542,1.54496723133478));
#19525=CARTESIAN_POINT('Ctrl Pts',(96.7237362899108,-1.58265126217805,1.53397101771918));
#19526=CARTESIAN_POINT('Ctrl Pts',(96.7245977770186,-1.59359891095592,1.52251723803876));
#19527=CARTESIAN_POINT('Ctrl Pts',(96.7246237984946,-1.59392953755357,1.52217110025116));
#19528=CARTESIAN_POINT('Ctrl Pts',(96.7246765545904,-1.59459974951247,1.52146898781758));
#19529=CARTESIAN_POINT('Ctrl Pts',(96.724703288933,-1.59493932850801,1.52111300711513));
#19530=CARTESIAN_POINT('Ctrl Pts',(96.7247576031014,-1.59562911724371,1.52038941655998));
#19531=CARTESIAN_POINT('Ctrl Pts',(96.7247851825895,-1.59597931921882,1.52002179932065));
#19532=CARTESIAN_POINT('Ctrl Pts',(96.7248413363122,-1.59669223828425,1.51927290936653));
#19533=CARTESIAN_POINT('Ctrl Pts',(96.7248699101362,-1.59705494592726,1.51889162767531));
#19534=CARTESIAN_POINT('Ctrl Pts',(96.7249282225963,-1.59779502175202,1.51811309482505));
#19535=CARTESIAN_POINT('Ctrl Pts',(96.7249579607335,-1.59817237844339,1.51771583275533));
#19536=CARTESIAN_POINT('Ctrl Pts',(96.7250187975307,-1.59894421956128,1.51690267035238));
#19537=CARTESIAN_POINT('Ctrl Pts',(96.7250498955828,-1.59933868997506,1.51648675673094));
#19538=CARTESIAN_POINT('Ctrl Pts',(96.7250928023211,-1.59988284951363,1.51591256848462));
#19539=CARTESIAN_POINT('Ctrl Pts',(96.7251046170066,-1.60003267727788,1.51575442572354));
#19540=CARTESIAN_POINT('Ctrl Pts',(96.7251320127,-1.60038007086697,1.51538764391634));
#19541=CARTESIAN_POINT('Ctrl Pts',(96.7251475929585,-1.60057761937088,1.51517898841412));
#19542=CARTESIAN_POINT('Ctrl Pts',(96.7251839639256,-1.60103873885075,1.51469175206577));
#19543=CARTESIAN_POINT('Ctrl Pts',(96.7252047532565,-1.60130227797765,1.51441314099579));
#19544=CARTESIAN_POINT('Ctrl Pts',(96.7259092265188,-1.61023152824141,1.50496828539381));
#19545=CARTESIAN_POINT('Ctrl Pts',(96.7265895026541,-1.61881858344139,1.49572775521251));
#19546=CARTESIAN_POINT('Ctrl Pts',(96.7280451287541,-1.63711293485152,1.47569909868651));
#19547=CARTESIAN_POINT('Ctrl Pts',(96.7288193512651,-1.64679399974583,1.46488775252045));
#19548=CARTESIAN_POINT('Ctrl Pts',(96.7308915050293,-1.67256366980744,1.43553108383457));
#19549=CARTESIAN_POINT('Ctrl Pts',(96.7321810891175,-1.6884505913895,1.41681099170187));
#19550=CARTESIAN_POINT('Ctrl Pts',(96.7401767529182,-1.78589772233918,1.29801816504647));
#19551=CARTESIAN_POINT('Ctrl Pts',(96.7465282937912,-1.85884928113737,1.19120362383043));
#19552=CARTESIAN_POINT('Ctrl Pts',(96.7573557862813,-1.96815903338244,0.996417738584225));
#19553=CARTESIAN_POINT('Ctrl Pts',(96.761869776937,-2.00896108881992,0.911357619124146));
#19554=CARTESIAN_POINT('Ctrl Pts',(96.7690085482016,-2.06315811919891,0.776896571692167));
#19555=CARTESIAN_POINT('Ctrl Pts',(96.7715421473601,-2.08049259709879,0.729204857658749));
#19556=CARTESIAN_POINT('Ctrl Pts',(96.7752295517117,-2.10270124374175,0.660841115319203));
#19557=CARTESIAN_POINT('Ctrl Pts',(96.7763265038397,-2.10894696041381,0.640629503795274));
#19558=CARTESIAN_POINT('Ctrl Pts',(96.7782946067704,-2.11949164736252,0.604679444358499));
#19559=CARTESIAN_POINT('Ctrl Pts',(96.779159915934,-2.12390867252279,0.588977073682936));
#19560=CARTESIAN_POINT('Ctrl Pts',(96.7804943751342,-2.13037936283693,0.564954145421908));
#19561=CARTESIAN_POINT('Ctrl Pts',(96.7809565875128,-2.13255955115943,0.556667918760472));
#19562=CARTESIAN_POINT('Ctrl Pts',(96.7818103938466,-2.13647374436715,0.541430753199892));
#19563=CARTESIAN_POINT('Ctrl Pts',(96.7822011589115,-2.13822224176788,0.534483827163808));
#19564=CARTESIAN_POINT('Ctrl Pts',(96.7831003291304,-2.14214800019384,0.518558857447746));
#19565=CARTESIAN_POINT('Ctrl Pts',(96.7836099773771,-2.1443026982404,0.50957558359606));
#19566=CARTESIAN_POINT('Ctrl Pts',(96.7852164928162,-2.1508779529591,0.481381978685206));
#19567=CARTESIAN_POINT('Ctrl Pts',(96.7863238778525,-2.15509718384751,0.462126228467932));
#19568=CARTESIAN_POINT('Ctrl Pts',(96.7954033472618,-2.1872357871918,0.305427045769771));
#19569=CARTESIAN_POINT('Ctrl Pts',(96.8039015004029,-2.20223396910464,0.165670333820707));
#19570=CARTESIAN_POINT('Ctrl Pts',(96.8212496308491,-2.20557267074338,-0.123476300175564));
#19571=CARTESIAN_POINT('Ctrl Pts',(96.8300336253042,-2.19219320486518,-0.272211415067468));
#19572=CARTESIAN_POINT('Ctrl Pts',(96.8397474961803,-2.15911116626638,-0.443275148117128));
#19573=CARTESIAN_POINT('Ctrl Pts',(96.8411422515811,-2.15388966926638,-0.467988517811588));
#19574=CARTESIAN_POINT('Ctrl Pts',(96.8433177788552,-2.14499806131925,-0.506764519960096));
#19575=CARTESIAN_POINT('Ctrl Pts',(96.8441075472288,-2.14161182432808,-0.520889402720316));
#19576=CARTESIAN_POINT('Ctrl Pts',(96.8455812737711,-2.13499525557279,-0.547332995751281));
#19577=CARTESIAN_POINT('Ctrl Pts',(96.8462662420241,-2.13179732235706,-0.559659124288174));
#19578=CARTESIAN_POINT('Ctrl Pts',(96.8477996890475,-2.12436202988242,-0.587328975223473));
#19579=CARTESIAN_POINT('Ctrl Pts',(96.8486461929131,-2.12006489052959,-0.602655985702586));
#19580=CARTESIAN_POINT('Ctrl Pts',(96.851129068441,-2.10689321662102,-0.647751348012335));
#19581=CARTESIAN_POINT('Ctrl Pts',(96.8527503672805,-2.09755482642524,-0.677380772237077));
#19582=CARTESIAN_POINT('Ctrl Pts',(96.8616122968508,-2.04247638475602,-0.84005865737921));
#19583=CARTESIAN_POINT('Ctrl Pts',(96.8684440770106,-1.98470461317013,-0.968690146620194));
#19584=CARTESIAN_POINT('Ctrl Pts',(96.8801631542396,-1.86469323380246,-1.17935948782349));
#19585=CARTESIAN_POINT('Ctrl Pts',(96.885059729989,-1.80826769929528,-1.26417373357032));
#19586=CARTESIAN_POINT('Ctrl Pts',(96.89179893821,-1.72655025242824,-1.37028328134208));
#19587=CARTESIAN_POINT('Ctrl Pts',(96.8934405196446,-1.70635530487693,-1.39535065326524));
#19588=CARTESIAN_POINT('Ctrl Pts',(96.8962783448656,-1.67116520247631,-1.4371242852469));
#19589=CARTESIAN_POINT('Ctrl Pts',(96.8974586892698,-1.65645022292543,-1.45406049655015));
#19590=CARTESIAN_POINT('Ctrl Pts',(96.8991761491611,-1.63498930339738,-1.47801237445083));
#19591=CARTESIAN_POINT('Ctrl Pts',(96.8996988765888,-1.62845100103476,-1.48521309289721));
#19592=CARTESIAN_POINT('Ctrl Pts',(96.9006153981239,-1.61698203136213,-1.49767724240482));
#19593=CARTESIAN_POINT('Ctrl Pts',(96.9010075909095,-1.61207286349252,-1.5029601105726));
#19594=CARTESIAN_POINT('Ctrl Pts',(96.9018525612768,-1.60149500303637,-1.51423173554284));
#19595=CARTESIAN_POINT('Ctrl Pts',(96.9023058945727,-1.59581869659414,-1.52021270772353));
#19596=CARTESIAN_POINT('Ctrl Pts',(96.9035572835009,-1.5801418718059,-1.53654640484188));
#19597=CARTESIAN_POINT('Ctrl Pts',(96.9043602930301,-1.57007345824655,-1.54683305582083));
#19598=CARTESIAN_POINT('Ctrl Pts',(96.908933751301,-1.51263189462613,-1.60438106099893));
#19599=CARTESIAN_POINT('Ctrl Pts',(96.9128366591611,-1.46322985090542,-1.64956076996027));
#19600=CARTESIAN_POINT('Ctrl Pts',(96.9244021095839,-1.31338961811199,-1.77456084169117));
#19601=CARTESIAN_POINT('Ctrl Pts',(96.9321959358845,-1.20794413543602,-1.84795320428208));
#19602=CARTESIAN_POINT('Ctrl Pts',(96.9460332677269,-1.00536352258569,-1.9641667567872));
#19603=CARTESIAN_POINT('Ctrl Pts',(96.9521263590037,-0.910367205245671,
-2.00996101675701));
#19604=CARTESIAN_POINT('Ctrl Pts',(96.9593017337332,-0.790463425678604,
-2.05750891647851));
#19605=CARTESIAN_POINT('Ctrl Pts',(96.960605655235,-0.768338510283478,-2.06587302705679));
#19606=CARTESIAN_POINT('Ctrl Pts',(96.9626724093394,-0.732738520079864,
-2.07868019947362));
#19607=CARTESIAN_POINT('Ctrl Pts',(96.9634427936861,-0.719348185310399,
-2.08335194146431));
#19608=CARTESIAN_POINT('Ctrl Pts',(96.9648999020293,-0.693795921853906,
-2.0919911181715));
#19609=CARTESIAN_POINT('Ctrl Pts',(96.9655873952018,-0.681642767865331,
-2.09598253004958));
#19610=CARTESIAN_POINT('Ctrl Pts',(96.9671529231258,-0.653750082155866,
-2.10487495022109));
#19611=CARTESIAN_POINT('Ctrl Pts',(96.9680286232363,-0.63798883693985,-2.10970566427644));
#19612=CARTESIAN_POINT('Ctrl Pts',(96.9707535716296,-0.58846174028786,-2.12427958380524));
#19613=CARTESIAN_POINT('Ctrl Pts',(96.9725824343572,-0.554515344022683,
-2.13339257573941));
#19614=CARTESIAN_POINT('Ctrl Pts',(96.9834267738383,-0.349418258915584,
-2.1832248004513));
#19615=CARTESIAN_POINT('Ctrl Pts',(96.9917799621534,-0.174120346396682,
-2.20414351491874));
#19616=CARTESIAN_POINT('Ctrl Pts',(97.0049604920597,0.0971591693623677,
-2.20392107304026));
#19617=CARTESIAN_POINT('Ctrl Pts',(97.0096515444659,0.192397192657645,-2.19765510492763));
#19618=CARTESIAN_POINT('Ctrl Pts',(97.0157052999137,0.307624569032217,-2.18252587211148));
#19619=CARTESIAN_POINT('Ctrl Pts',(97.0168060435193,0.32828844823504,-2.17951340672665));
#19620=CARTESIAN_POINT('Ctrl Pts',(97.0184274893463,0.358239390798993,-2.17471145142811));
#19621=CARTESIAN_POINT('Ctrl Pts',(97.0189359270168,0.367563235036731,-2.17315499210909));
#19622=CARTESIAN_POINT('Ctrl Pts',(97.019833077463,0.383888895198691,-2.17032162811321));
#19623=CARTESIAN_POINT('Ctrl Pts',(97.0202203330934,0.390894957635741,-2.16907071900586));
#19624=CARTESIAN_POINT('Ctrl Pts',(97.0210682396807,0.406144101216154,-2.16627175318586));
#19625=CARTESIAN_POINT('Ctrl Pts',(97.021529587742,0.41438431775802,-2.16471059775278));
#19626=CARTESIAN_POINT('Ctrl Pts',(97.0228242546749,0.4373577393494,-2.16022217468882));
#19627=CARTESIAN_POINT('Ctrl Pts',(97.0236630784208,0.452069957475402,-2.15719131382255));
#19628=CARTESIAN_POINT('Ctrl Pts',(97.0292626515689,0.549243059122469,-2.13613500468892));
#19629=CARTESIAN_POINT('Ctrl Pts',(97.0342335472769,0.630634372245638,-2.11353693434011));
#19630=CARTESIAN_POINT('Ctrl Pts',(97.041116723865,0.739778607725766,-2.07636675175192));
#19631=CARTESIAN_POINT('Ctrl Pts',(97.0429704294909,0.768822906975942,-2.06578860844319));
#19632=CARTESIAN_POINT('Ctrl Pts',(97.0503214017933,0.882932866118027,-2.02148902226851));
#19633=CARTESIAN_POINT('Ctrl Pts',(97.0558255421417,0.96608978979318,-1.98309359730076));
#19634=CARTESIAN_POINT('Ctrl Pts',(97.0667400773437,1.12909288601398,-1.89513775357621));
#19635=CARTESIAN_POINT('Ctrl Pts',(97.0721334573602,1.20864898903318,-1.84541837313117));
#19636=CARTESIAN_POINT('Ctrl Pts',(97.0786212759344,1.30349829395804,-1.77736812486294));
#19637=CARTESIAN_POINT('Ctrl Pts',(97.0798887196036,1.32197992795045,-1.76366504201175));
#19638=CARTESIAN_POINT('Ctrl Pts',(97.0819117049338,1.35139214437696,-1.74113539688895));
#19639=CARTESIAN_POINT('Ctrl Pts',(97.0826742465388,1.36245845850767,-1.73248958434262));
#19640=CARTESIAN_POINT('Ctrl Pts',(97.0841252237058,1.38347280620687,-1.71574575721257));
#19641=CARTESIAN_POINT('Ctrl Pts',(97.0848143262208,1.39343422448967,-1.70766553533358));
#19642=CARTESIAN_POINT('Ctrl Pts',(97.0863807290431,1.41603009739407,-1.68900747670599));
#19643=CARTESIAN_POINT('Ctrl Pts',(97.0872557194261,1.4286176818724,-1.67837392497714));
#19644=CARTESIAN_POINT('Ctrl Pts',(97.0900294886792,1.46839463477093,-1.64399999082385));
#19645=CARTESIAN_POINT('Ctrl Pts',(97.091906452713,1.49512126406873,-1.6197318828176));
#19646=CARTESIAN_POINT('Ctrl Pts',(97.1027342386393,1.64777465345655,-1.4741211198295));
#19647=CARTESIAN_POINT('Ctrl Pts',(97.111036359595,1.7594917697619,-1.33880015054082));
#19648=CARTESIAN_POINT('Ctrl Pts',(97.1241510822338,1.90542219097849,-1.11176029859333));
#19649=CARTESIAN_POINT('Ctrl Pts',(97.1288268912561,1.95157136135416,-1.02859641079584));
#19650=CARTESIAN_POINT('Ctrl Pts',(97.1348619589028,2.00112471832434,-0.923877996788937));
#19651=CARTESIAN_POINT('Ctrl Pts',(97.1359610220495,2.00977445259573,-0.904907331524308));
#19652=CARTESIAN_POINT('Ctrl Pts',(97.1375804355341,2.02195033961223,-0.877167071072994));
#19653=CARTESIAN_POINT('Ctrl Pts',(97.1380885643828,2.02569150324292,-0.868492471769706));
#19654=CARTESIAN_POINT('Ctrl Pts',(97.1389853746996,2.03215290966729,-0.853241581537137));
#19655=CARTESIAN_POINT('Ctrl Pts',(97.1393726028778,2.03489723787633,-0.846675778941045));
#19656=CARTESIAN_POINT('Ctrl Pts',(97.1402207007066,2.04080809714263,-0.83233930320665));
#19657=CARTESIAN_POINT('Ctrl Pts',(97.1406822702671,2.04396202021073,-0.8245639212205));
#19658=CARTESIAN_POINT('Ctrl Pts',(97.141978140253,2.0526445202068,-0.802802986094939));
#19659=CARTESIAN_POINT('Ctrl Pts',(97.1428179612323,2.05807436467379,-0.788778831424574));
#19660=CARTESIAN_POINT('Ctrl Pts',(97.1484550104124,2.09325585346522,-0.695075432104919));
#19661=CARTESIAN_POINT('Ctrl Pts',(97.1534655674885,2.11851480296155,-0.6137933669029));
#19662=CARTESIAN_POINT('Ctrl Pts',(97.1603327832216,2.14623711295988,-0.502175831762616));
#19663=CARTESIAN_POINT('Ctrl Pts',(97.16213035524,2.1528675169356,-0.472943685966584));
#19664=CARTESIAN_POINT('Ctrl Pts',(97.1693631031807,2.17710796390953,-0.354967187465543));
#19665=CARTESIAN_POINT('Ctrl Pts',(97.174805668844,2.18984334957001,-0.265307757864347));
#19666=CARTESIAN_POINT('Ctrl Pts',(97.1838555687657,2.20203854153165,-0.112305641845383));
#19667=CARTESIAN_POINT('Ctrl Pts',(97.1875156020542,2.20434939746418,-0.0493053001917814));
#19668=CARTESIAN_POINT('Ctrl Pts',(97.1935536373236,2.20368886979997,0.0568660252298257));
#19669=CARTESIAN_POINT('Ctrl Pts',(97.1959711269057,2.20215297016257,0.10000521861277));
#19670=CARTESIAN_POINT('Ctrl Pts',(97.1993324559348,2.19819328859719,0.160874041877885));
#19671=CARTESIAN_POINT('Ctrl Pts',(97.200308661995,2.19681925300165,0.178659977188884));
#19672=CARTESIAN_POINT('Ctrl Pts',(97.2019842072095,2.19407144129111,0.209368877241939));
#19673=CARTESIAN_POINT('Ctrl Pts',(97.2026866898402,2.19279903907687,0.222299798888353));
#19674=CARTESIAN_POINT('Ctrl Pts',(97.2041181766385,2.18995881683217,0.248760673481563));
#19675=CARTESIAN_POINT('Ctrl Pts',(97.2048467953177,2.18837977733654,0.262288874490857));
#19676=CARTESIAN_POINT('Ctrl Pts',(97.2066901966621,2.18404461340287,0.296659922797866));
#19677=CARTESIAN_POINT('Ctrl Pts',(97.2077994953409,2.1811154477108,0.31747980634697));
#19678=CARTESIAN_POINT('Ctrl Pts',(97.212184735964,2.16825640628148,0.400274014343198));
#19679=CARTESIAN_POINT('Ctrl Pts',(97.2153869030998,2.15597888599049,0.461856116178701));
#19680=CARTESIAN_POINT('Ctrl Pts',(97.2259518493747,2.10590445597134,0.666918872713687));
#19681=CARTESIAN_POINT('Ctrl Pts',(97.2329834075584,2.05626755979001,0.807080093503427));
#19682=CARTESIAN_POINT('Ctrl Pts',(97.2447858205727,1.95292685016179,1.02589842417721));
#19683=CARTESIAN_POINT('Ctrl Pts',(97.2494320307433,1.90756869800671,1.10795710403447));
#19684=CARTESIAN_POINT('Ctrl Pts',(97.2551597798963,1.84900030694052,1.1996007809649));
#19685=CARTESIAN_POINT('Ctrl Pts',(97.2559626175308,1.84073558702578,1.21224446477707));
#19686=CARTESIAN_POINT('Ctrl Pts',(97.2572202021618,1.82772106692227,1.23171459301282));
#19687=CARTESIAN_POINT('Ctrl Pts',(97.2576691888672,1.82306133985835,1.23860101873783));
#19688=CARTESIAN_POINT('Ctrl Pts',(97.2585117882168,1.81429538068962,1.25139924924421));
#19689=CARTESIAN_POINT('Ctrl Pts',(97.2589047532771,1.81019902687534,1.2573174966686));
#19690=CARTESIAN_POINT('Ctrl Pts',(97.2598178553037,1.80066095528577,1.27095448952557));
#19691=CARTESIAN_POINT('Ctrl Pts',(97.2603393637083,1.79519853552882,1.27865843823917));
#19692=CARTESIAN_POINT('Ctrl Pts',(97.2620080303289,1.77766690001696,1.30305047891928));
#19693=CARTESIAN_POINT('Ctrl Pts',(97.263166725419,1.76541353855386,1.31960415797661));
#19694=CARTESIAN_POINT('Ctrl Pts',(97.2709099317092,1.6828667606546,1.4279129869599));
#19695=CARTESIAN_POINT('Ctrl Pts',(97.2778480086945,1.60568520366668,1.5141819456416));
#19696=CARTESIAN_POINT('Ctrl Pts',(97.2915767065824,1.44041902272347,1.67199443470786));
#19697=CARTESIAN_POINT('Ctrl Pts',(97.2983454381227,1.35285361347675,1.74360639672075));
#19698=CARTESIAN_POINT('Ctrl Pts',(97.3075023826572,1.22332316842911,1.83387963628771));
#19699=CARTESIAN_POINT('Ctrl Pts',(97.3100730656522,1.18568920656398,1.85843363857608));
#19700=CARTESIAN_POINT('Ctrl Pts',(97.3144987477146,1.11859715317977,1.89933904364343));
#19701=CARTESIAN_POINT('Ctrl Pts',(97.3163709276377,1.08946671918313,1.91619697260344));
#19702=CARTESIAN_POINT('Ctrl Pts',(97.3191094371916,1.04574898388846,1.94017725915547));
#19703=CARTESIAN_POINT('Ctrl Pts',(97.3199940472822,1.03145167067706,1.94781575235171));
#19704=CARTESIAN_POINT('Ctrl Pts',(97.32156506603,1.00575029909533,1.96118463513976));
#19705=CARTESIAN_POINT('Ctrl Pts',(97.3222535698145,0.994378393033289,1.96697495110217));
#19706=CARTESIAN_POINT('Ctrl Pts',(97.3237082908929,0.970124217661067,1.97906052477348));
#19707=CARTESIAN_POINT('Ctrl Pts',(97.3244735669585,0.9572294779321,1.98532951881347));
#19708=CARTESIAN_POINT('Ctrl Pts',(97.3265284606674,0.92224640270622,2.00191705413486));
#19709=CARTESIAN_POINT('Ctrl Pts',(97.3278097973551,0.900046213809432,2.01199582363293));
#19710=CARTESIAN_POINT('Ctrl Pts',(97.3346722029672,0.779161736921847,2.06447541421351));
#19711=CARTESIAN_POINT('Ctrl Pts',(97.3400167873889,0.67764152974858,2.09998979031711));
#19712=CARTESIAN_POINT('Ctrl Pts',(97.3520014294974,0.440474355470889,2.16395551373336));
#19713=CARTESIAN_POINT('Ctrl Pts',(97.358541452668,0.303940165817493,2.18731286520492));
#19714=CARTESIAN_POINT('Ctrl Pts',(97.3682155346815,0.110845247889272,2.20190889510372));
#19715=CARTESIAN_POINT('Ctrl Pts',(97.3710429553254,0.0554303166240454,
2.204));
#19716=CARTESIAN_POINT('Ctrl Pts',(97.3739726165667,2.84962952926334E-13,
2.204));
#19717=CARTESIAN_POINT('Origin',(66.9212607628943,0.,0.));
#19718=CARTESIAN_POINT('',(98.2342289786285,-4.90954494829228E-11,2.204));
#19719=CARTESIAN_POINT('',(98.1265335566918,1.10792599586928E-10,2.204));
#19720=CARTESIAN_POINT('',(66.9212607628943,-2.69912154532077E-16,2.204));
#19721=CARTESIAN_POINT('',(98.234131513614,0.00201603627767701,2.20399905814364));
#19722=CARTESIAN_POINT('Ctrl Pts',(98.2342289786285,-4.90954494829228E-11,
2.204));
#19723=CARTESIAN_POINT('Ctrl Pts',(98.2341964771698,0.000672034549184021,
2.20400000000001));
#19724=CARTESIAN_POINT('Ctrl Pts',(98.2341639765587,0.0013440747103176,
2.203999692629));
#19725=CARTESIAN_POINT('Ctrl Pts',(98.234131476736,0.00201612022368431,
2.20399907787169));
#19726=CARTESIAN_POINT('Ctrl Pts',(98.2341314808713,0.00201603471236662,
2.20399907794991));
#19727=CARTESIAN_POINT('Ctrl Pts',(98.2270286940923,0.148890558395576,2.20386472937369));
#19728=CARTESIAN_POINT('Ctrl Pts',(98.2200162894635,0.295367267902672,2.1890492234998));
#19729=CARTESIAN_POINT('Ctrl Pts',(98.2113583876976,0.457622973732756,2.15604922601805));
#19730=CARTESIAN_POINT('Ctrl Pts',(98.2103679273346,0.475934480175369,2.15208117309754));
#19731=CARTESIAN_POINT('Ctrl Pts',(98.2088831959586,0.502962919153579,2.14586236583687));
#19732=CARTESIAN_POINT('Ctrl Pts',(98.2083985523008,0.511720679096874,2.1437907854999));
#19733=CARTESIAN_POINT('Ctrl Pts',(98.2075639974475,0.526684432213262,2.14015430986641));
#19734=CARTESIAN_POINT('Ctrl Pts',(98.2072155996558,0.532896662933989,2.13861593246557));
#19735=CARTESIAN_POINT('Ctrl Pts',(98.2064123666166,0.547138557964507,2.13502320607096));
#19736=CARTESIAN_POINT('Ctrl Pts',(98.2059565152877,0.555163231328493,2.13295064969659));
#19737=CARTESIAN_POINT('Ctrl Pts',(98.2046797457496,0.577485382080972,2.12705093931864));
#19738=CARTESIAN_POINT('Ctrl Pts',(98.2038534904878,0.59175602530952,2.12312501921843));
#19739=CARTESIAN_POINT('Ctrl Pts',(98.198582860931,0.681773656154838,2.09738270870218));
#19740=CARTESIAN_POINT('Ctrl Pts',(98.1939547778149,0.756337961105009,2.07166121677561));
#19741=CARTESIAN_POINT('Ctrl Pts',(98.1842391738421,0.907422718482555,2.01029837012323));
#19742=CARTESIAN_POINT('Ctrl Pts',(98.1791507272464,0.983605511284114,1.97414176607105));
#19743=CARTESIAN_POINT('Ctrl Pts',(98.1687082226919,1.13674177185232,1.89039283539825));
#19744=CARTESIAN_POINT('Ctrl Pts',(98.1633719055042,1.21322135735851,1.84224409854052));
#19745=CARTESIAN_POINT('Ctrl Pts',(98.1550365790212,1.33101780050677,1.75755760689232));
#19746=CARTESIAN_POINT('Ctrl Pts',(98.1519454099199,1.37429313851033,1.72393046208749));
#19747=CARTESIAN_POINT('Ctrl Pts',(98.1478420768162,1.43117574346848,1.67622501018439));
#19748=CARTESIAN_POINT('Ctrl Pts',(98.1467750738386,1.44591254615666,1.66352975224271));
#19749=CARTESIAN_POINT('Ctrl Pts',(98.1449973597383,1.47036678567529,1.64189274862729));
#19750=CARTESIAN_POINT('Ctrl Pts',(98.1442823489422,1.48017520655513,1.63305592401006));
#19751=CARTESIAN_POINT('Ctrl Pts',(98.1428758770113,1.49941151789059,1.61540941231897));
#19752=CARTESIAN_POINT('Ctrl Pts',(98.1421842775774,1.50884260991705,1.60660401395612));
#19753=CARTESIAN_POINT('Ctrl Pts',(98.140504825421,1.53167154123291,1.58491130518202));
#19754=CARTESIAN_POINT('Ctrl Pts',(98.1395208140174,1.54498483002539,1.57193621334693));
#19755=CARTESIAN_POINT('Ctrl Pts',(98.1361524779763,1.59031589444744,1.52662438055568));
#19756=CARTESIAN_POINT('Ctrl Pts',(98.1338045142788,1.62149641931428,1.49346455484011));
#19757=CARTESIAN_POINT('Ctrl Pts',(98.1231149061195,1.76083472979661,1.3357687069836));
#19758=CARTESIAN_POINT('Ctrl Pts',(98.1152950718779,1.85581961493352,1.2003133039549));
#19759=CARTESIAN_POINT('Ctrl Pts',(98.1028316747418,1.97847465183779,0.975483312113148));
#19760=CARTESIAN_POINT('Ctrl Pts',(98.0983318461788,2.01712870580203,0.89281487377718));
#19761=CARTESIAN_POINT('Ctrl Pts',(98.092516249203,2.05802197242458,0.789035504941786));
#19762=CARTESIAN_POINT('Ctrl Pts',(98.0914410903269,2.06523081027701,0.769969550612961));
#19763=CARTESIAN_POINT('Ctrl Pts',(98.0898535410641,2.07534450936516,0.742056461935275));
#19764=CARTESIAN_POINT('Ctrl Pts',(98.0893528047449,2.07845957260975,0.733286045112361));
#19765=CARTESIAN_POINT('Ctrl Pts',(98.0884675542279,2.08383319289476,0.71784732992193));
#19766=CARTESIAN_POINT('Ctrl Pts',(98.0880844359571,2.08611548391388,0.711187564045846));
#19767=CARTESIAN_POINT('Ctrl Pts',(98.0872439175435,2.09102787352245,0.696625999352936));
#19768=CARTESIAN_POINT('Ctrl Pts',(98.0867858150148,2.09364506978451,0.688720311820022));
#19769=CARTESIAN_POINT('Ctrl Pts',(98.0854968197394,2.10084403031279,0.666554354979852));
#19770=CARTESIAN_POINT('Ctrl Pts',(98.0846604318679,2.10532523715449,0.652262193102311));
#19771=CARTESIAN_POINT('Ctrl Pts',(98.0789547604889,2.13465093323776,0.555280303672436));
#19772=CARTESIAN_POINT('Ctrl Pts',(98.0738653228241,2.1547613324381,0.471244809066967));
#19773=CARTESIAN_POINT('Ctrl Pts',(98.0668797545049,2.17525681082835,0.356106148807667));
#19774=CARTESIAN_POINT('Ctrl Pts',(98.0650425495561,2.17999460212193,0.325848556119625));
#19775=CARTESIAN_POINT('Ctrl Pts',(98.0576172487835,2.1965704567011,0.203334049657282));
#19776=CARTESIAN_POINT('Ctrl Pts',(98.0520248087108,2.20319442002864,0.110464420699547));
#19777=CARTESIAN_POINT('Ctrl Pts',(98.0411877751727,2.20465262720684,-0.0736963547790665));
#19778=CARTESIAN_POINT('Ctrl Pts',(98.0359488171857,2.19971949004917,-0.164808255245748));
#19779=CARTESIAN_POINT('Ctrl Pts',(98.0296228387593,2.18652619401912,-0.277911088664449));
#19780=CARTESIAN_POINT('Ctrl Pts',(98.0283725011856,2.18354760031787,-0.300418544628712));
#19781=CARTESIAN_POINT('Ctrl Pts',(98.0263749497759,2.17818727087814,-0.33661412960573));
#19782=CARTESIAN_POINT('Ctrl Pts',(98.0256209361727,2.17602300308047,-0.350332358966968));
#19783=CARTESIAN_POINT('Ctrl Pts',(98.0241851999535,2.17163141200565,-0.37655586892633));
#19784=CARTESIAN_POINT('Ctrl Pts',(98.0235028338366,2.16942537170103,-0.389064105271915));
#19785=CARTESIAN_POINT('Ctrl Pts',(98.0219506110023,2.16413501261388,-0.417615265017852));
#19786=CARTESIAN_POINT('Ctrl Pts',(98.0210830327286,2.16098018493305,-0.433644465119808));
#19787=CARTESIAN_POINT('Ctrl Pts',(98.0187776223919,2.15206735768126,-0.476413901197065));
#19788=CARTESIAN_POINT('Ctrl Pts',(98.0173499567301,2.14598922882145,-0.503084916011854));
#19789=CARTESIAN_POINT('Ctrl Pts',(98.0074517682779,2.09995193375955,-0.689048108089269));
#19790=CARTESIAN_POINT('Ctrl Pts',(97.9995695902075,2.04279620316474,-0.84354845259458));
#19791=CARTESIAN_POINT('Ctrl Pts',(97.985680886833,1.91382144496436,-1.09999389293011));
#19792=CARTESIAN_POINT('Ctrl Pts',(97.9797091064346,1.84957233960686,-1.20489594053515));
#19793=CARTESIAN_POINT('Ctrl Pts',(97.9724274054087,1.76767962971349,-1.31649890443952));
#19794=CARTESIAN_POINT('Ctrl Pts',(97.9715968276835,1.75829272715278,-1.32900989338143));
#19795=CARTESIAN_POINT('Ctrl Pts',(97.9703077986237,1.74367481469261,-1.34806688502856));
#19796=CARTESIAN_POINT('Ctrl Pts',(97.9698556485647,1.73853812279116,-1.35468497327124));
#19797=CARTESIAN_POINT('Ctrl Pts',(97.9690152779514,1.72897786039534,-1.36685843713993));
#19798=CARTESIAN_POINT('Ctrl Pts',(97.9686277979266,1.72456502976831,-1.37242190400762));
#19799=CARTESIAN_POINT('Ctrl Pts',(97.9677382804848,1.71442327904374,-1.38508194719722));
#19800=CARTESIAN_POINT('Ctrl Pts',(97.9672350449682,1.70867713688196,-1.39216436386839));
#19801=CARTESIAN_POINT('Ctrl Pts',(97.9656246944401,1.69025596913404,-1.41458355414198));
#19802=CARTESIAN_POINT('Ctrl Pts',(97.964506739891,1.67741748605676,-1.42978403745721));
#19803=CARTESIAN_POINT('Ctrl Pts',(97.9556166213358,1.57477120516605,-1.54802946627635));
#19804=CARTESIAN_POINT('Ctrl Pts',(97.9473453343271,1.47576520690954,-1.64268430517698));
#19805=CARTESIAN_POINT('Ctrl Pts',(97.9329622909477,1.28792582248012,-1.79149846521664));
#19806=CARTESIAN_POINT('Ctrl Pts',(97.9268343703174,1.20282376070939,-1.84971295152347));
#19807=CARTESIAN_POINT('Ctrl Pts',(97.9174595881689,1.06254300646766,-1.9318821484809));
#19808=CARTESIAN_POINT('Ctrl Pts',(97.9140888186555,1.00992647470567,-1.95990197216647));
#19809=CARTESIAN_POINT('Ctrl Pts',(97.9096896484184,0.938274529594791,-1.99440575040151));
#19810=CARTESIAN_POINT('Ctrl Pts',(97.9085953453793,0.92019692882798,-2.00281078467114));
#19811=CARTESIAN_POINT('Ctrl Pts',(97.9067850201258,0.889871725667172,-2.01641295755481));
#19812=CARTESIAN_POINT('Ctrl Pts',(97.9060643501978,0.877686894505272,-2.02174643059638));
#19813=CARTESIAN_POINT('Ctrl Pts',(97.904656052782,0.853657363335134,-2.03200631040321));
#19814=CARTESIAN_POINT('Ctrl Pts',(97.903968189957,0.841816473414707,-2.03694024806575));
#19815=CARTESIAN_POINT('Ctrl Pts',(97.9023136846849,0.813088726235343,-2.04861741961784));
#19816=CARTESIAN_POINT('Ctrl Pts',(97.9013506072553,0.796160039317716,-2.05525565977577));
#19817=CARTESIAN_POINT('Ctrl Pts',(97.8981383396155,0.739025604811676,-2.07684788467916));
#19818=CARTESIAN_POINT('Ctrl Pts',(97.8959209736701,0.698464758573888,-2.09083793629388));
#19819=CARTESIAN_POINT('Ctrl Pts',(97.8852335567862,0.4981548369933,-2.15344748637794));
#19820=CARTESIAN_POINT('Ctrl Pts',(97.8773131338468,0.33365129859371,-2.18498808745691));
#19821=CARTESIAN_POINT('Ctrl Pts',(97.8646918669091,0.074908841732648,-2.20466867155915));
#19822=CARTESIAN_POINT('Ctrl Pts',(97.860130490703,-0.0176833789133627,
-2.20586931871442));
#19823=CARTESIAN_POINT('Ctrl Pts',(97.8542395149129,-0.130560089371308,
-2.20022522979623));
#19824=CARTESIAN_POINT('Ctrl Pts',(97.8531574100386,-0.151036713195516,
-2.19891447093399));
#19825=CARTESIAN_POINT('Ctrl Pts',(97.8515614550278,-0.18079487221796,-2.19659197339418));
#19826=CARTESIAN_POINT('Ctrl Pts',(97.8510594333584,-0.190093553904758,
-2.19580680338551));
#19827=CARTESIAN_POINT('Ctrl Pts',(97.8501693191745,-0.206464079299201,
-2.19431973175649));
#19828=CARTESIAN_POINT('Ctrl Pts',(97.8497826040625,-0.213537913102688,
-2.1936426462477));
#19829=CARTESIAN_POINT('Ctrl Pts',(97.8489378660569,-0.22890481819751,-2.19209673804386));
#19830=CARTESIAN_POINT('Ctrl Pts',(97.8484791710552,-0.237196150659646,
-2.191215075285));
#19831=CARTESIAN_POINT('Ctrl Pts',(97.8471869515582,-0.260413701318517,
-2.18861290690973));
#19832=CARTESIAN_POINT('Ctrl Pts',(97.8463478899117,-0.275327346641447,
-2.18678681608414));
#19833=CARTESIAN_POINT('Ctrl Pts',(97.8405323299162,-0.377688835355098,
-2.17318954809243));
#19834=CARTESIAN_POINT('Ctrl Pts',(97.8353260417339,-0.464372628511995,
-2.15632948391451));
#19835=CARTESIAN_POINT('Ctrl Pts',(97.8285151252054,-0.574729665139916,
-2.12790139447152));
#19836=CARTESIAN_POINT('Ctrl Pts',(97.8269713737107,-0.599541039995519,
-2.12104433057611));
#19837=CARTESIAN_POINT('Ctrl Pts',(97.8201369658291,-0.708698511495932,
-2.08880833509606));
#19838=CARTESIAN_POINT('Ctrl Pts',(97.8148368380289,-0.791602650909097,
-2.05882010483688));
#19839=CARTESIAN_POINT('Ctrl Pts',(97.8057848284572,-0.932370723110672,
-1.99813728621645));
#19840=CARTESIAN_POINT('Ctrl Pts',(97.8019916761946,-0.991077973277591,
-1.96967847846661));
#19841=CARTESIAN_POINT('Ctrl Pts',(97.7957676258696,-1.08726428822042,-1.91766015675686));
#19842=CARTESIAN_POINT('Ctrl Pts',(97.793293708354,-1.1254502014196,-1.89550160820989));
#19843=CARTESIAN_POINT('Ctrl Pts',(97.7898749869974,-1.17813887378265,-1.86277337311782));
#19844=CARTESIAN_POINT('Ctrl Pts',(97.7888960578268,-1.1932156894578,-1.85315196100542));
#19845=CARTESIAN_POINT('Ctrl Pts',(97.7872226316068,-1.21896499102532,-1.83627525642573));
#19846=CARTESIAN_POINT('Ctrl Pts',(97.786524905561,-1.22969377704381,-1.82910789493519));
#19847=CARTESIAN_POINT('Ctrl Pts',(97.7851944842947,-1.25013398266664,-1.81519168700584));
#19848=CARTESIAN_POINT('Ctrl Pts',(97.7845612457082,-1.2598552059718,-1.80845810089318));
#19849=CARTESIAN_POINT('Ctrl Pts',(97.7829111735733,-1.28516184569802,-1.79062589401322));
#19850=CARTESIAN_POINT('Ctrl Pts',(97.7818991750059,-1.30065793982881,-1.77940187038127));
#19851=CARTESIAN_POINT('Ctrl Pts',(97.7783272911256,-1.35523255419602,-1.73877887372259));
#19852=CARTESIAN_POINT('Ctrl Pts',(97.7758100770669,-1.39347787274922,-1.70828192034592));
#19853=CARTESIAN_POINT('Ctrl Pts',(97.7651787266073,-1.55318945527303,-1.57199140756423));
#19854=CARTESIAN_POINT('Ctrl Pts',(97.7575419554663,-1.66386874066126,-1.45433713338));
#19855=CARTESIAN_POINT('Ctrl Pts',(97.7452968975513,-1.81517521581479,-1.25337333055694));
#19856=CARTESIAN_POINT('Ctrl Pts',(97.7408284892806,-1.86509870164113,-1.1777986378688));
#19857=CARTESIAN_POINT('Ctrl Pts',(97.7350513625245,-1.92036407056261,-1.08177191335072));
#19858=CARTESIAN_POINT('Ctrl Pts',(97.733979776966,-1.93025238694271,-1.06402739665507));
#19859=CARTESIAN_POINT('Ctrl Pts',(97.7323965533995,-1.94430544193075,-1.03796856302757));
#19860=CARTESIAN_POINT('Ctrl Pts',(97.7318964802183,-1.94866533144386,-1.02976007355393));
#19861=CARTESIAN_POINT('Ctrl Pts',(97.7310084897439,-1.95626524409029,-1.01523039139992));
#19862=CARTESIAN_POINT('Ctrl Pts',(97.730621925645,-1.95952681417951,-1.00892076787065));
#19863=CARTESIAN_POINT('Ctrl Pts',(97.7297759055652,-1.96656254990003,-0.99514706902523));
#19864=CARTESIAN_POINT('Ctrl Pts',(97.7293157594011,-1.97032469410964,-0.987677349495753));
#19865=CARTESIAN_POINT('Ctrl Pts',(97.7280156296397,-1.98077735356021,-0.966626242502675));
#19866=CARTESIAN_POINT('Ctrl Pts',(97.7271700051735,-1.98737044889088,-0.952997319026223));
#19867=CARTESIAN_POINT('Ctrl Pts',(97.7209709952405,-2.03426931223523,-0.853446790372424));
#19868=CARTESIAN_POINT('Ctrl Pts',(97.7153522306968,-2.06912490360362,-0.765076349048055));
#19869=CARTESIAN_POINT('Ctrl Pts',(97.7040550325685,-2.12689312019023,-0.585441296467138));
#19870=CARTESIAN_POINT('Ctrl Pts',(97.6983901197412,-2.14988200016011,-0.494392652519302));
#19871=CARTESIAN_POINT('Ctrl Pts',(97.6862797948423,-2.18710615492108,-0.293811698490952));
#19872=CARTESIAN_POINT('Ctrl Pts',(97.6798914887765,-2.19906131384067,-0.184101963131649));
#19873=CARTESIAN_POINT('Ctrl Pts',(97.672438936157,-2.20355541761292,-0.0502266972342789));
#19874=CARTESIAN_POINT('Ctrl Pts',(97.6711304045857,-2.20396851336426,-0.0264963000790465));
#19875=CARTESIAN_POINT('Ctrl Pts',(97.6690630214664,-2.20401595614999,0.0113455247942131));
#19876=CARTESIAN_POINT('Ctrl Pts',(97.668296493327,-2.20389817088405,0.0254542980631437));
#19877=CARTESIAN_POINT('Ctrl Pts',(97.6668508535382,-2.20341788975674,0.0522069995418382));
#19878=CARTESIAN_POINT('Ctrl Pts',(97.6661709378527,-2.20308201225533,0.0648507843412206));
#19879=CARTESIAN_POINT('Ctrl Pts',(97.6646285693699,-2.20206818246986,0.0936682546476339));
#19880=CARTESIAN_POINT('Ctrl Pts',(97.6637683214156,-2.20132084550619,0.109838864833555));
#19881=CARTESIAN_POINT('Ctrl Pts',(97.6615287678349,-2.19889633229499,0.152179219122569));
#19882=CARTESIAN_POINT('Ctrl Pts',(97.660158465896,-2.1969301332216,0.178330200876878));
#19883=CARTESIAN_POINT('Ctrl Pts',(97.6496653700656,-2.17812058866877,0.380234802495082));
#19884=CARTESIAN_POINT('Ctrl Pts',(97.6412413281975,-2.14068174594103,0.553420249749476));
#19885=CARTESIAN_POINT('Ctrl Pts',(97.6272034225631,-2.04603638624366,0.82712017748541));
#19886=CARTESIAN_POINT('Ctrl Pts',(97.6216698916669,-2.00093609665839,0.930935918138566));
#19887=CARTESIAN_POINT('Ctrl Pts',(97.6149133865938,-1.94089879706604,1.04439633208269));
#19888=CARTESIAN_POINT('Ctrl Pts',(97.6140975160856,-1.93357474963509,1.05789437103285));
#19889=CARTESIAN_POINT('Ctrl Pts',(97.6128265871947,-1.9220672861888,1.07858357841687));
#19890=CARTESIAN_POINT('Ctrl Pts',(97.6123775565714,-1.91798306868425,1.08582969746773));
#19891=CARTESIAN_POINT('Ctrl Pts',(97.6115398283888,-1.9103321749431,1.09922587514199));
#19892=CARTESIAN_POINT('Ctrl Pts',(97.6111518290531,-1.90677664794049,1.10538199435749));
#19893=CARTESIAN_POINT('Ctrl Pts',(97.6102570685265,-1.89854935397514,1.11946910413472));
#19894=CARTESIAN_POINT('Ctrl Pts',(97.6097490550458,-1.89385763210844,1.12738812646058));
#19895=CARTESIAN_POINT('Ctrl Pts',(97.6081077340414,-1.87862825246728,1.15273001498408));
#19896=CARTESIAN_POINT('Ctrl Pts',(97.6069630142231,-1.86789899788994,1.17003584206345));
#19897=CARTESIAN_POINT('Ctrl Pts',(97.5985365871519,-1.78801171501633,1.29499078590272));
#19898=CARTESIAN_POINT('Ctrl Pts',(97.5908194350833,-1.70984018335472,1.39657757580317));
#19899=CARTESIAN_POINT('Ctrl Pts',(97.5766110097006,-1.54982539267471,1.57081466211898));
#19900=CARTESIAN_POINT('Ctrl Pts',(97.5701280359214,-1.47052337993432,1.64529091183963));
#19901=CARTESIAN_POINT('Ctrl Pts',(97.5614767918747,-1.35404517101395,1.73950329386397));
#19902=CARTESIAN_POINT('Ctrl Pts',(97.5591302115008,-1.32132406607491,1.76448662523567));
#19903=CARTESIAN_POINT('Ctrl Pts',(97.5550520758503,-1.26241636581344,1.80690583681462));
#19904=CARTESIAN_POINT('Ctrl Pts',(97.5533067126958,-1.23652100993213,1.82472455993171));
#19905=CARTESIAN_POINT('Ctrl Pts',(97.5507213058967,-1.19713865766299,1.85060023894928));
#19906=CARTESIAN_POINT('Ctrl Pts',(97.5498656613931,-1.18393303038082,1.85907633183826));
#19907=CARTESIAN_POINT('Ctrl Pts',(97.5483386098135,-1.16005916731179,1.87404231852859));
#19908=CARTESIAN_POINT('Ctrl Pts',(97.5476653090696,-1.14942426456643,1.88058388599666));
#19909=CARTESIAN_POINT('Ctrl Pts',(97.5462236315818,-1.12642179970852,1.89446476032377));
#19910=CARTESIAN_POINT('Ctrl Pts',(97.545456369417,-1.11403679087701,1.90177412984097));
#19911=CARTESIAN_POINT('Ctrl Pts',(97.5434010150872,-1.08048113071215,1.92113767792088));
#19912=CARTESIAN_POINT('Ctrl Pts',(97.5421211534776,-1.05918039966124,1.93296311254612));
#19913=CARTESIAN_POINT('Ctrl Pts',(97.533905054495,-0.919925260327332,2.00727952436785));
#19914=CARTESIAN_POINT('Ctrl Pts',(97.5273511557389,-0.796693711034568,
2.05930034086876));
#19915=CARTESIAN_POINT('Ctrl Pts',(97.5153898051674,-0.561415042203283,
2.13431467012366));
#19916=CARTESIAN_POINT('Ctrl Pts',(97.5099687605223,-0.450836392335652,
2.16037725357833));
#19917=CARTESIAN_POINT('Ctrl Pts',(97.5015869948797,-0.285289435514515,
2.18612742443964));
#19918=CARTESIAN_POINT('Ctrl Pts',(97.498823830923,-0.231544647041384,2.19247106995145));
#19919=CARTESIAN_POINT('Ctrl Pts',(97.4952641590509,-0.16445539315729,2.19789558458065));
#19920=CARTESIAN_POINT('Ctrl Pts',(97.4945596228558,-0.151276623791019,
2.19884195499415));
#19921=CARTESIAN_POINT('Ctrl Pts',(97.4934260549857,-0.130250957173296,
2.20016190047417));
#19922=CARTESIAN_POINT('Ctrl Pts',(97.4930011542303,-0.122408995833271,
2.2006121271039));
#19923=CARTESIAN_POINT('Ctrl Pts',(97.4921802432662,-0.107338378271166,
2.20139656512652));
#19924=CARTESIAN_POINT('Ctrl Pts',(97.4917845794784,-0.100110263445036,
2.20173710828022));
#19925=CARTESIAN_POINT('Ctrl Pts',(97.4909109000873,-0.0842245746124726,
2.20240715666773));
#19926=CARTESIAN_POINT('Ctrl Pts',(97.4904320531775,-0.0755664671458614,
2.20272121854087));
#19927=CARTESIAN_POINT('Ctrl Pts',(97.4887213868041,-0.0447972006561152,
2.20365571262157));
#19928=CARTESIAN_POINT('Ctrl Pts',(97.4874753344573,-0.0226795084516347,
2.2039942950221));
#19929=CARTESIAN_POINT('Ctrl Pts',(97.4862047194752,-0.000374238760942893,
2.20399997617039));
#19930=CARTESIAN_POINT('Ctrl Pts',(97.4861940592604,-0.000187119293676933,
2.204));
#19931=CARTESIAN_POINT('Ctrl Pts',(97.4861833980632,7.30595079061364E-14,
2.204));
#19932=CARTESIAN_POINT('',(98.1264124210279,0.00202521791090988,2.20399901632153));
#19933=CARTESIAN_POINT('Ctrl Pts',(97.3739726165667,2.84962952926334E-13,
2.204));
#19934=CARTESIAN_POINT('Ctrl Pts',(97.3739819747949,-0.000177061274001931,
2.204));
#19935=CARTESIAN_POINT('Ctrl Pts',(97.3739913340681,-0.000354122705178335,
2.20399997866332));
#19936=CARTESIAN_POINT('Ctrl Pts',(97.3747093145248,-0.0139355771281671,
2.20399670540768));
#19937=CARTESIAN_POINT('Ctrl Pts',(97.3754238522532,-0.0273393297549546,
2.2038711897423));
#19938=CARTESIAN_POINT('Ctrl Pts',(97.3765724525169,-0.0486859079455517,
2.20347653248173));
#19939=CARTESIAN_POINT('Ctrl Pts',(97.3770022540842,-0.0566300679190517,
2.20328667634892));
#19940=CARTESIAN_POINT('Ctrl Pts',(97.3778319623752,-0.0718771134803473,
2.20283977582093));
#19941=CARTESIAN_POINT('Ctrl Pts',(97.3782315074757,-0.0791799748172588,
2.20258936781612));
#19942=CARTESIAN_POINT('Ctrl Pts',(97.3792021658589,-0.0968303197220333,
2.20189626377793));
#19943=CARTESIAN_POINT('Ctrl Pts',(97.3797752608472,-0.107176132191411,
2.20141693806801));
#19944=CARTESIAN_POINT('Ctrl Pts',(97.3818185428568,-0.143814463421693,
2.19946058781237));
#19945=CARTESIAN_POINT('Ctrl Pts',(97.3833085595131,-0.170082525029899,
2.19758533101828));
#19946=CARTESIAN_POINT('Ctrl Pts',(97.3871133075049,-0.236228120220814,
2.19167025761626));
#19947=CARTESIAN_POINT('Ctrl Pts',(97.3894517636776,-0.276040118186444,
2.18701252439136));
#19948=CARTESIAN_POINT('Ctrl Pts',(97.4014905943729,-0.477977128922408,
2.15778568355572));
#19949=CARTESIAN_POINT('Ctrl Pts',(97.4115163510578,-0.63712951839179,2.11626412101436));
#19950=CARTESIAN_POINT('Ctrl Pts',(97.4258180588067,-0.865220482945043,
2.02866096924363));
#19951=CARTESIAN_POINT('Ctrl Pts',(97.4304173668542,-0.938600866347626,
1.99577114704289));
#19952=CARTESIAN_POINT('Ctrl Pts',(97.4361450241761,-1.03023623264672,1.94852412254093));
#19953=CARTESIAN_POINT('Ctrl Pts',(97.4373972753262,-1.05028284493818,1.93779228802723));
#19954=CARTESIAN_POINT('Ctrl Pts',(97.4394020226731,-1.08238611266425,1.91996142736631));
#19955=CARTESIAN_POINT('Ctrl Pts',(97.4401612937447,-1.09454715501363,1.91305465619415));
#19956=CARTESIAN_POINT('Ctrl Pts',(97.4416098387214,-1.11774851771764,1.89958395264468));
#19957=CARTESIAN_POINT('Ctrl Pts',(97.4422997358875,-1.12879878081432,1.89303836836737));
#19958=CARTESIAN_POINT('Ctrl Pts',(97.4438884091429,-1.1542404510714,1.87766609828384));
#19959=CARTESIAN_POINT('Ctrl Pts',(97.444784596387,-1.16858901406738,1.86876984487803));
#19960=CARTESIAN_POINT('Ctrl Pts',(97.4476458532578,-1.21436968482697,1.83965188538493));
#19961=CARTESIAN_POINT('Ctrl Pts',(97.4495874108625,-1.24539095433056,1.81879475893508));
#19962=CARTESIAN_POINT('Ctrl Pts',(97.4574885874725,-1.37109110770589,1.72955563093991));
#19963=CARTESIAN_POINT('Ctrl Pts',(97.4631965762121,-1.46079592978947,1.65448841864075));
#19964=CARTESIAN_POINT('Ctrl Pts',(97.4758452255033,-1.64725260362292,1.47141414430502));
#19965=CARTESIAN_POINT('Ctrl Pts',(97.482724459768,-1.74015249385944,1.36027987710566));
#19966=CARTESIAN_POINT('Ctrl Pts',(97.4914874927377,-1.83556992010327,1.22021460888507));
#19967=CARTESIAN_POINT('Ctrl Pts',(97.4927973148451,-1.84928795568172,1.19932254933254));
#19968=CARTESIAN_POINT('Ctrl Pts',(97.4946853321914,-1.86823069530785,1.16937554361205));
#19969=CARTESIAN_POINT('Ctrl Pts',(97.4952456021945,-1.87375126651548,1.16050905870864));
#19970=CARTESIAN_POINT('Ctrl Pts',(97.4962016895332,-1.88299679633206,1.14542203186685));
#19971=CARTESIAN_POINT('Ctrl Pts',(97.4965954006271,-1.88675453626141,1.13922161372622));
#19972=CARTESIAN_POINT('Ctrl Pts',(97.497421797826,-1.89453711216455,1.12623592895191));
#19973=CARTESIAN_POINT('Ctrl Pts',(97.4978548202945,-1.89855618027697,1.11944748128097));
#19974=CARTESIAN_POINT('Ctrl Pts',(97.4990152505106,-1.90917334749632,1.10129281084416));
#19975=CARTESIAN_POINT('Ctrl Pts',(97.4997466340787,-1.91570627171185,1.08988907198684));
#19976=CARTESIAN_POINT('Ctrl Pts',(97.5034005576062,-1.94758746315883,1.03306560912353));
#19977=CARTESIAN_POINT('Ctrl Pts',(97.5064039727004,-1.97142267587486,0.986819797132146));
#19978=CARTESIAN_POINT('Ctrl Pts',(97.516479817641,-2.04460298224934,0.831578753127164));
#19979=CARTESIAN_POINT('Ctrl Pts',(97.5237387560793,-2.08671379769918,0.719409118755392));
#19980=CARTESIAN_POINT('Ctrl Pts',(97.5386095833968,-2.15495791891663,0.480081561977351));
#19981=CARTESIAN_POINT('Ctrl Pts',(97.5461687191451,-2.17940286109702,0.352893433862224));
#19982=CARTESIAN_POINT('Ctrl Pts',(97.5547399703849,-2.19505632379293,0.199865057164176));
#19983=CARTESIAN_POINT('Ctrl Pts',(97.5560948390168,-2.1971458193073,0.175409871931398));
#19984=CARTESIAN_POINT('Ctrl Pts',(97.5582303958799,-2.19982007954713,0.136448356161442));
#19985=CARTESIAN_POINT('Ctrl Pts',(97.5590193373013,-2.20067071885515,0.121962853453563));
#19986=CARTESIAN_POINT('Ctrl Pts',(97.5604857631126,-2.20199335039197,0.0948704659505365));
#19987=CARTESIAN_POINT('Ctrl Pts',(97.5611643136169,-2.20250027086464,0.0822659498780257));
#19988=CARTESIAN_POINT('Ctrl Pts',(97.562689370637,-2.20340079092127,0.0537872920686311));
#19989=CARTESIAN_POINT('Ctrl Pts',(97.563533864746,-2.203731116609,0.0379117633153341));
#19990=CARTESIAN_POINT('Ctrl Pts',(97.5660597055858,-2.20420886298624,-0.00987401067489685));
#19991=CARTESIAN_POINT('Ctrl Pts',(97.5677248169345,-2.20383490307266,-0.041785924652601));
#19992=CARTESIAN_POINT('Ctrl Pts',(97.5715305317536,-2.20136787091285,-0.115541767656108));
#19993=CARTESIAN_POINT('Ctrl Pts',(97.5736561849177,-2.19877453792642,-0.157356898562891));
#19994=CARTESIAN_POINT('Ctrl Pts',(97.5813522913052,-2.18489850743498,-0.310353805301846));
#19995=CARTESIAN_POINT('Ctrl Pts',(97.5867359227622,-2.16635796577845,-0.420708531048811));
#19996=CARTESIAN_POINT('Ctrl Pts',(97.5980787429663,-2.11002410553565,-0.648470812702674));
#19997=CARTESIAN_POINT('Ctrl Pts',(97.6040241653249,-2.07059829559113,-0.765070218177005));
#19998=CARTESIAN_POINT('Ctrl Pts',(97.611502212167,-2.01344792055741,-0.89669930338991));
#19999=CARTESIAN_POINT('Ctrl Pts',(97.6125907346971,-2.00496095628523,-0.915518253611297));
#20000=CARTESIAN_POINT('Ctrl Pts',(97.6141920526109,-1.99226499833944,-0.942646726437807));
#20001=CARTESIAN_POINT('Ctrl Pts',(97.6146928292216,-1.98826546823607,-0.951053676704099));
#20002=CARTESIAN_POINT('Ctrl Pts',(97.6155857691474,-1.98108600146899,-0.96590157376129));
#20003=CARTESIAN_POINT('Ctrl Pts',(97.615976612355,-1.97792767295364,-0.972352669846697));
#20004=CARTESIAN_POINT('Ctrl Pts',(97.6168290536901,-1.9710060005592,-0.986317371540986));
#20005=CARTESIAN_POINT('Ctrl Pts',(97.6172913221002,-1.96723126175271,-0.993824818377816));
#20006=CARTESIAN_POINT('Ctrl Pts',(97.6186146263424,-1.95636229517063,-1.0151371698018));
#20007=CARTESIAN_POINT('Ctrl Pts',(97.6194816960089,-1.94916518215492,-1.02888870549905));
#20008=CARTESIAN_POINT('Ctrl Pts',(97.6270775724272,-1.88540415336963,-1.14764671996824));
#20009=CARTESIAN_POINT('Ctrl Pts',(97.6342216465019,-1.82055253913967,-1.24796841965663));
#20010=CARTESIAN_POINT('Ctrl Pts',(97.6515000574071,-1.6453413775444,-1.47608329081852));
#20011=CARTESIAN_POINT('Ctrl Pts',(97.6615598903468,-1.52778712644834,-1.5974523571444));
#20012=CARTESIAN_POINT('Ctrl Pts',(97.6725282191723,-1.37658453976377,-1.72144285152621));
#20013=CARTESIAN_POINT('Ctrl Pts',(97.6740332760261,-1.35531239180769,-1.73824017300327));
#20014=CARTESIAN_POINT('Ctrl Pts',(97.6764213586757,-1.32071964089144,-1.76453475785449));
#20015=CARTESIAN_POINT('Ctrl Pts',(97.6773141728215,-1.3075942149623,-1.77428314280375));
#20016=CARTESIAN_POINT('Ctrl Pts',(97.6788963189765,-1.28399406147609,-1.79140707668303));
#20017=CARTESIAN_POINT('Ctrl Pts',(97.6795878162813,-1.27356131723132,-1.79883897145362));
#20018=CARTESIAN_POINT('Ctrl Pts',(97.6810336301148,-1.25150259012361,-1.81426467377766));
#20019=CARTESIAN_POINT('Ctrl Pts',(97.6817871706801,-1.23986341774322,-1.82223866648223));
#20020=CARTESIAN_POINT('Ctrl Pts',(97.6837746678168,-1.20879267812378,-1.8430896941797));
#20021=CARTESIAN_POINT('Ctrl Pts',(97.685001282394,-1.1892317571805,-1.85577133342138));
#20022=CARTESIAN_POINT('Ctrl Pts',(97.6913726989779,-1.08568193615649,-1.9205944530065));
#20023=CARTESIAN_POINT('Ctrl Pts',(97.6963187873895,-0.998452872225329,
-1.96735432699394));
#20024=CARTESIAN_POINT('Ctrl Pts',(97.7054405244625,-0.828809683280653,
-2.04409290292321));
#20025=CARTESIAN_POINT('Ctrl Pts',(97.7096322243475,-0.747178790498817,
-2.07532294885835));
#20026=CARTESIAN_POINT('Ctrl Pts',(97.7149424145905,-0.642706693712112,
-2.10832601612228));
#20027=CARTESIAN_POINT('Ctrl Pts',(97.7160227410944,-0.621402576493553,
-2.11470312471845));
#20028=CARTESIAN_POINT('Ctrl Pts',(97.7215623459013,-0.512197546036285,
-2.14559947968191));
#20029=CARTESIAN_POINT('Ctrl Pts',(97.7260940873225,-0.422939459807675,
-2.16496243376399));
#20030=CARTESIAN_POINT('Ctrl Pts',(97.7316955557646,-0.317738287106051,
-2.18102933171089));
#20031=CARTESIAN_POINT('Ctrl Pts',(97.7325021707979,-0.302705094658855,
-2.18316654545788));
#20032=CARTESIAN_POINT('Ctrl Pts',(97.7337691941737,-0.279300215716118,
-2.18624754796377));
#20033=CARTESIAN_POINT('Ctrl Pts',(97.7342238356476,-0.270942900717031,
-2.18729899447918));
#20034=CARTESIAN_POINT('Ctrl Pts',(97.7350710489905,-0.255450885156529,
-2.18915792028793));
#20035=CARTESIAN_POINT('Ctrl Pts',(97.7354628946299,-0.248318029337369,
-2.18997847164813));
#20036=CARTESIAN_POINT('Ctrl Pts',(97.7363744062227,-0.231798906178504,
-2.19179706259628));
#20037=CARTESIAN_POINT('Ctrl Pts',(97.7368954485079,-0.222410132989806,
-2.19276966929072));
#20038=CARTESIAN_POINT('Ctrl Pts',(97.738574920074,-0.192307671445952,-2.19569274271431));
#20039=CARTESIAN_POINT('Ctrl Pts',(97.7397452168932,-0.171573081793909,
-2.1974101743485));
#20040=CARTESIAN_POINT('Ctrl Pts',(97.7463051244522,-0.0564663164599404,
-2.20530535113382));
#20041=CARTESIAN_POINT('Ctrl Pts',(97.7519308003735,0.0381968605775587,
-2.20569676577638));
#20042=CARTESIAN_POINT('Ctrl Pts',(97.7680024877513,0.305716337298381,-2.18957468754965));
#20043=CARTESIAN_POINT('Ctrl Pts',(97.7784470432829,0.477042010246259,-2.15873763621696));
#20044=CARTESIAN_POINT('Ctrl Pts',(97.7903709925441,0.678740718238237,-2.09721813832766));
#20045=CARTESIAN_POINT('Ctrl Pts',(97.7924562422922,0.714208000318182,-2.08540644843603));
#20046=CARTESIAN_POINT('Ctrl Pts',(97.7954306040527,0.765064723374735,-2.06701980380745));
#20047=CARTESIAN_POINT('Ctrl Pts',(97.7963431909379,0.780705368306805,-2.06116327588443));
#20048=CARTESIAN_POINT('Ctrl Pts',(97.7979478943161,0.808267982826948,-2.05048389474645));
#20049=CARTESIAN_POINT('Ctrl Pts',(97.7986423954203,0.820217006189716,-2.04573346436582));
#20050=CARTESIAN_POINT('Ctrl Pts',(97.8000823258282,0.845029278348068,-2.03561679924722));
#20051=CARTESIAN_POINT('Ctrl Pts',(97.8008271088029,0.857884599671815,-2.03023256316219));
#20052=CARTESIAN_POINT('Ctrl Pts',(97.8027642724922,0.891369193842865,-2.01583326608879));
#20053=CARTESIAN_POINT('Ctrl Pts',(97.8039499826605,0.911913199454301,-2.00662332353375));
#20054=CARTESIAN_POINT('Ctrl Pts',(97.8096332006951,1.01053632718484,-1.96058275225846));
#20055=CARTESIAN_POINT('Ctrl Pts',(97.8139823653554,1.08655065568207,-1.91949945101085));
#20056=CARTESIAN_POINT('Ctrl Pts',(97.8230472533561,1.242866426604,-1.82274647232381));
#20057=CARTESIAN_POINT('Ctrl Pts',(97.827726812465,1.32227331827657,-1.76598851095926));
#20058=CARTESIAN_POINT('Ctrl Pts',(97.8334973248447,1.41440353975956,-1.6904281953571));
#20059=CARTESIAN_POINT('Ctrl Pts',(97.8345480103002,1.43094260181277,-1.67645104721564));
#20060=CARTESIAN_POINT('Ctrl Pts',(97.8402631369872,1.51940550957116,-1.59942815015354));
#20061=CARTESIAN_POINT('Ctrl Pts',(97.844998745795,1.58736650273789,-1.53200109219444));
#20062=CARTESIAN_POINT('Ctrl Pts',(97.8508333955863,1.66082609118795,-1.44896687516706));
#20063=CARTESIAN_POINT('Ctrl Pts',(97.8516429821602,1.67080638286428,-1.43744715237542));
#20064=CARTESIAN_POINT('Ctrl Pts',(97.852913696849,1.68612360862381,-1.41939224429187));
#20065=CARTESIAN_POINT('Ctrl Pts',(97.8533690045229,1.69154403011381,-1.41292814966029));
#20066=CARTESIAN_POINT('Ctrl Pts',(97.8542167800272,1.70150785390662,-1.40090633254908));
#20067=CARTESIAN_POINT('Ctrl Pts',(97.8546085124826,1.70606136886374,-1.39535734866986));
#20068=CARTESIAN_POINT('Ctrl Pts',(97.8555188576842,1.7165278840395,-1.38247486971013));
#20069=CARTESIAN_POINT('Ctrl Pts',(97.8560388343347,1.72242103875097,-1.37512563087084));
#20070=CARTESIAN_POINT('Ctrl Pts',(97.8577113915479,1.74111353889568,-1.35150589956215));
#20071=CARTESIAN_POINT('Ctrl Pts',(97.8588757082453,1.75373047864788,-1.33509321654486));
#20072=CARTESIAN_POINT('Ctrl Pts',(97.8653693414449,1.8220663559535,-1.24355859094771));
#20073=CARTESIAN_POINT('Ctrl Pts',(97.8709299076844,1.87318700428819,-1.16513147935897));
#20074=CARTESIAN_POINT('Ctrl Pts',(97.8867432156117,2.00287201345458,-0.935467617968303));
#20075=CARTESIAN_POINT('Ctrl Pts',(97.8970025351573,2.06913352433295,-0.778009283013917));
#20076=CARTESIAN_POINT('Ctrl Pts',(97.9089101026323,2.12766464329978,-0.57639549512677));
#20077=CARTESIAN_POINT('Ctrl Pts',(97.911128043,2.13769142225382,-0.53801883861719));
#20078=CARTESIAN_POINT('Ctrl Pts',(97.9141905327883,2.15028717083408,-0.483874831859102));
#20079=CARTESIAN_POINT('Ctrl Pts',(97.9150627414692,2.15372842600312,-0.468320035671987));
#20080=CARTESIAN_POINT('Ctrl Pts',(97.9165758244013,2.15944057344553,-0.44110484387122));
#20081=CARTESIAN_POINT('Ctrl Pts',(97.9172190702162,2.16178637500982,-0.429460999503841));
#20082=CARTESIAN_POINT('Ctrl Pts',(97.9185652382825,2.16652051057689,-0.404939976325212));
#20083=CARTESIAN_POINT('Ctrl Pts',(97.9192674861822,2.16888843066598,-0.392059297458112));
#20084=CARTESIAN_POINT('Ctrl Pts',(97.9209485458857,2.1743096034208,-0.361016486117458));
#20085=CARTESIAN_POINT('Ctrl Pts',(97.9219237573924,2.17725032399774,-0.342835542204599));
#20086=CARTESIAN_POINT('Ctrl Pts',(97.9253622284056,2.18688298118481,-0.27814800665365));
#20087=CARTESIAN_POINT('Ctrl Pts',(97.9277860402161,2.19231561007408,-0.231465246782524));
#20088=CARTESIAN_POINT('Ctrl Pts',(97.933782719309,2.20221182180191,-0.113753385568278));
#20089=CARTESIAN_POINT('Ctrl Pts',(97.9373011977993,2.20473618571501,-0.0426147235539901));
#20090=CARTESIAN_POINT('Ctrl Pts',(97.9470994666509,2.20213854181846,0.158079084840689));
#20091=CARTESIAN_POINT('Ctrl Pts',(97.9532441747371,2.18904118587867,0.287226901422236));
#20092=CARTESIAN_POINT('Ctrl Pts',(97.9628429614164,2.15263911371629,0.477345821720939));
#20093=CARTESIAN_POINT('Ctrl Pts',(97.9660841463907,2.13786770859342,0.539661483749271));
#20094=CARTESIAN_POINT('Ctrl Pts',(97.9702116916643,2.11651923553246,0.614951569365691));
#20095=CARTESIAN_POINT('Ctrl Pts',(97.9709699493356,2.11249868263135,0.628624213468353));
#20096=CARTESIAN_POINT('Ctrl Pts',(97.9721768363128,2.10595245589098,0.650113617608666));
#20097=CARTESIAN_POINT('Ctrl Pts',(97.9726205400178,2.10351512626195,0.657957119733583));
#20098=CARTESIAN_POINT('Ctrl Pts',(97.9734591143958,2.09885316962731,0.672668933381644));
#20099=CARTESIAN_POINT('Ctrl Pts',(97.9738534128662,2.0966385709436,0.679540152644493));
#20100=CARTESIAN_POINT('Ctrl Pts',(97.9747867315503,2.0913430721749,0.695698131298487));
#20101=CARTESIAN_POINT('Ctrl Pts',(97.9753273557646,2.08823404048459,0.704975403945903));
#20102=CARTESIAN_POINT('Ctrl Pts',(97.9771374536119,2.07768269338171,0.735778061222619));
#20103=CARTESIAN_POINT('Ctrl Pts',(97.978421415721,2.06996873209409,0.757208092262544));
#20104=CARTESIAN_POINT('Ctrl Pts',(97.9815929731626,2.05032155044888,0.809244421388071));
#20105=CARTESIAN_POINT('Ctrl Pts',(97.9834959449694,2.03803365385381,0.839710442971886));
#20106=CARTESIAN_POINT('Ctrl Pts',(97.9916128052812,1.9833383580868,0.967039103553963));
#20107=CARTESIAN_POINT('Ctrl Pts',(97.9980046678959,1.93467110809167,1.0610570907159));
#20108=CARTESIAN_POINT('Ctrl Pts',(98.0124525349574,1.80882924258046,1.266503319181));
#20109=CARTESIAN_POINT('Ctrl Pts',(98.0204332694513,1.7277461150675,1.37506237726276));
#20110=CARTESIAN_POINT('Ctrl Pts',(98.0297899952272,1.6162777451201,1.49874620159978));
#20111=CARTESIAN_POINT('Ctrl Pts',(98.0315272672179,1.59484941166543,1.52152864643736));
#20112=CARTESIAN_POINT('Ctrl Pts',(98.0341199605864,1.56176280023523,1.55523878899609));
#20113=CARTESIAN_POINT('Ctrl Pts',(98.0349905858811,1.55045931789572,1.5665077904208));
#20114=CARTESIAN_POINT('Ctrl Pts',(98.0365462587481,1.52991661443372,1.58654763365523));
#20115=CARTESIAN_POINT('Ctrl Pts',(98.0372332443933,1.52072195880423,1.59536296010865));
#20116=CARTESIAN_POINT('Ctrl Pts',(98.0386946571425,1.50090143053726,1.61403872584742));
#20117=CARTESIAN_POINT('Ctrl Pts',(98.03946803314,1.49025362431559,1.62387507575358));
#20118=CARTESIAN_POINT('Ctrl Pts',(98.0412544372146,1.46529427071392,1.64648003773815));
#20119=CARTESIAN_POINT('Ctrl Pts',(98.042264092706,1.45091144941154,1.65916840947157));
#20120=CARTESIAN_POINT('Ctrl Pts',(98.0473853072951,1.3765816558494,1.72303557593424));
#20121=CARTESIAN_POINT('Ctrl Pts',(98.0513726957121,1.31408327236977,1.77116217553305));
#20122=CARTESIAN_POINT('Ctrl Pts',(98.0610995782985,1.15228120893595,1.88246753794252));
#20123=CARTESIAN_POINT('Ctrl Pts',(98.0667151949082,1.05025210956043,1.94123852519005));
#20124=CARTESIAN_POINT('Ctrl Pts',(98.0775576072156,0.848496048100299,2.0368715533644));
#20125=CARTESIAN_POINT('Ctrl Pts',(98.0827570055827,0.749846741641844,2.07521475979122));
#20126=CARTESIAN_POINT('Ctrl Pts',(98.0891234648794,0.634225338406635,2.11083113510916));
#20127=CARTESIAN_POINT('Ctrl Pts',(98.0899356809216,0.619564464011215,2.11518077475786));
#20128=CARTESIAN_POINT('Ctrl Pts',(98.0912096615471,0.596736938279598,2.12169563880535));
#20129=CARTESIAN_POINT('Ctrl Pts',(98.0916655581014,0.58860082857942,2.12396714122705));
#20130=CARTESIAN_POINT('Ctrl Pts',(98.0925138336167,0.573528460116436,2.12808190947564));
#20131=CARTESIAN_POINT('Ctrl Pts',(98.0929054691384,0.566596024351771,2.12993813256715));
#20132=CARTESIAN_POINT('Ctrl Pts',(98.0938147971304,0.550559011089369,2.13414835666179));
#20133=CARTESIAN_POINT('Ctrl Pts',(98.0943338426409,0.541448338719758,2.13647797152449));
#20134=CARTESIAN_POINT('Ctrl Pts',(98.0960003736084,0.512322359934135,2.14372727160456));
#20135=CARTESIAN_POINT('Ctrl Pts',(98.0971594812687,0.49225338654142,2.14842438928037));
#20136=CARTESIAN_POINT('Ctrl Pts',(98.1073165602986,0.317703723925351,2.18670350473883));
#20137=CARTESIAN_POINT('Ctrl Pts',(98.116963934652,0.16009919970521,2.20385379994168));
#20138=CARTESIAN_POINT('Ctrl Pts',(98.1264124982452,0.00202546956495211,
2.2039990692995));
#20139=CARTESIAN_POINT('Ctrl Pts',(98.126412512956,0.00202522345453538,
2.20399906952566));
#20140=CARTESIAN_POINT('Ctrl Pts',(98.1264528646512,0.00135014273495122,
2.20399968984775));
#20141=CARTESIAN_POINT('Ctrl Pts',(98.1264932125787,0.000675068216677538,
2.20399999999997));
#20142=CARTESIAN_POINT('Ctrl Pts',(98.1265335566918,1.10792599586928E-10,
2.204));
#20143=CARTESIAN_POINT('Origin',(66.9212607628943,0.,0.));
#20144=CARTESIAN_POINT('',(98.9822063149447,-1.02538676663964E-13,2.204));
#20145=CARTESIAN_POINT('',(98.8779717715633,2.72446158072696E-13,2.204));
#20146=CARTESIAN_POINT('',(66.9212607628943,-2.69912154532077E-16,2.204));
#20147=CARTESIAN_POINT('Ctrl Pts',(98.9822063149447,-3.98666500548274E-14,
2.204));
#20148=CARTESIAN_POINT('Ctrl Pts',(98.981345646301,0.0156268070781291,2.204));
#20149=CARTESIAN_POINT('Ctrl Pts',(98.9804901719241,0.0312534512830711,
2.20383380430557));
#20150=CARTESIAN_POINT('Ctrl Pts',(98.9789994524121,0.0586452158235635,
2.20325107173718));
#20151=CARTESIAN_POINT('Ctrl Pts',(98.9783619850133,0.0704110898098772,
2.20290645112726));
#20152=CARTESIAN_POINT('Ctrl Pts',(98.9770292359948,0.0951173970063678,
2.20198466176993));
#20153=CARTESIAN_POINT('Ctrl Pts',(98.9763346021306,0.108056668706093,2.20138763876887));
#20154=CARTESIAN_POINT('Ctrl Pts',(98.9746744975788,0.139124238152045,2.19967958725385));
#20155=CARTESIAN_POINT('Ctrl Pts',(98.9737125075476,0.15724568744745,2.19845847367306));
#20156=CARTESIAN_POINT('Ctrl Pts',(98.9703388404841,0.221186899601767,2.19335513051738));
#20157=CARTESIAN_POINT('Ctrl Pts',(98.9679648478299,0.266899565887535,2.1882630963279));
#20158=CARTESIAN_POINT('Ctrl Pts',(98.9621148908914,0.380855900092877,2.17194476393601));
#20159=CARTESIAN_POINT('Ctrl Pts',(98.958689960001,0.448793922597031,2.15893032782001));
#20160=CARTESIAN_POINT('Ctrl Pts',(98.9486393791114,0.64868511817622,2.11079295139281));
#20161=CARTESIAN_POINT('Ctrl Pts',(98.9421811202234,0.778097826067429,2.06659136720652));
#20162=CARTESIAN_POINT('Ctrl Pts',(98.9323659404591,0.958245081956869,1.98572518355226));
#20163=CARTESIAN_POINT('Ctrl Pts',(98.9292696643993,1.01283829191085,1.95844212634833));
#20164=CARTESIAN_POINT('Ctrl Pts',(98.9253116145229,1.07848270856545,1.92215691482094));
#20165=CARTESIAN_POINT('Ctrl Pts',(98.9245661459634,1.09067521273145,1.9152649211172));
#20166=CARTESIAN_POINT('Ctrl Pts',(98.9233778120495,1.10982167988839,1.90419998759224));
#20167=CARTESIAN_POINT('Ctrl Pts',(98.9229396872366,1.11681991226482,1.90010395325543));
#20168=CARTESIAN_POINT('Ctrl Pts',(98.9221104562412,1.12994661134344,1.89232338368031));
#20169=CARTESIAN_POINT('Ctrl Pts',(98.9217198954444,1.13607993612788,1.88864753365664));
#20170=CARTESIAN_POINT('Ctrl Pts',(98.9207942401351,1.15050262265826,1.87990799493628));
#20171=CARTESIAN_POINT('Ctrl Pts',(98.9202575550501,1.1587765289605,1.87481927204694));
#20172=CARTESIAN_POINT('Ctrl Pts',(98.9184559665107,1.18626981696341,1.8576584832453));
#20173=CARTESIAN_POINT('Ctrl Pts',(98.9171766422279,1.20533573481716,1.84534462994245));
#20174=CARTESIAN_POINT('Ctrl Pts',(98.914014181379,1.25146232681063,1.81453363643569));
#20175=CARTESIAN_POINT('Ctrl Pts',(98.9121156739281,1.27830667619018,1.79572328718996));
#20176=CARTESIAN_POINT('Ctrl Pts',(98.9040056786087,1.3899168975833,1.71374484695117));
#20177=CARTESIAN_POINT('Ctrl Pts',(98.8976156236718,1.47049830152077,1.64512123859726));
#20178=CARTESIAN_POINT('Ctrl Pts',(98.8831264167054,1.64271100952328,1.47566451683766));
#20179=CARTESIAN_POINT('Ctrl Pts',(98.8751039377492,1.73056789160358,1.37157918215866));
#20180=CARTESIAN_POINT('Ctrl Pts',(98.8657254942883,1.826011501533,1.23460903685701));
#20181=CARTESIAN_POINT('Ctrl Pts',(98.8640033250567,1.84320066659682,1.20879647517741));
#20182=CARTESIAN_POINT('Ctrl Pts',(98.8614335808711,1.86832538288025,1.16928453942366));
#20183=CARTESIAN_POINT('Ctrl Pts',(98.8605710468637,1.87666698684141,1.15584908588181));
#20184=CARTESIAN_POINT('Ctrl Pts',(98.8590302624156,1.89139948332306,1.13154011122728));
#20185=CARTESIAN_POINT('Ctrl Pts',(98.8583501039162,1.89784295323834,1.12069940791132));
#20186=CARTESIAN_POINT('Ctrl Pts',(98.8569038443129,1.91141287493478,1.09741623782729));
#20187=CARTESIAN_POINT('Ctrl Pts',(98.8561387651737,1.91851169009653,1.0849582875642));
#20188=CARTESIAN_POINT('Ctrl Pts',(98.8540619190326,1.9375575178991,1.05076261640857));
#20189=CARTESIAN_POINT('Ctrl Pts',(98.8527588727834,1.94926013840631,1.02889075688289));
#20190=CARTESIAN_POINT('Ctrl Pts',(98.8435389266839,2.03019365084294,0.871288906543657));
#20191=CARTESIAN_POINT('Ctrl Pts',(98.83613463766,2.08555588742027,0.728898700749735));
#20192=CARTESIAN_POINT('Ctrl Pts',(98.8221229188616,2.16209616604372,0.449293680386417));
#20193=CARTESIAN_POINT('Ctrl Pts',(98.8155249362084,2.18590674994476,0.313572565464096));
#20194=CARTESIAN_POINT('Ctrl Pts',(98.8073160820554,2.19850571833654,0.15678421013648));
#20195=CARTESIAN_POINT('Ctrl Pts',(98.8062700504793,2.19982644407811,0.137011839118037));
#20196=CARTESIAN_POINT('Ctrl Pts',(98.8047230093116,2.20136464715042,0.108132336014155));
#20197=CARTESIAN_POINT('Ctrl Pts',(98.8042329990128,2.20179258836586,0.0990368805215006));
#20198=CARTESIAN_POINT('Ctrl Pts',(98.8033553374221,2.20245387701171,0.0828452067917682));
#20199=CARTESIAN_POINT('Ctrl Pts',(98.8029689099464,2.20270931368415,0.0757501581093566));
#20200=CARTESIAN_POINT('Ctrl Pts',(98.8021216457691,2.20319176329827,0.0602695470396744));
#20201=CARTESIAN_POINT('Ctrl Pts',(98.8016601014888,2.20340518513577,0.0518840005104393));
#20202=CARTESIAN_POINT('Ctrl Pts',(98.8003279333011,2.2038804213938,0.0278087158807533));
#20203=CARTESIAN_POINT('Ctrl Pts',(98.7994510843705,2.20402254421296,0.0121174398909252));
#20204=CARTESIAN_POINT('Ctrl Pts',(98.7914864586338,2.20379346064208,-0.129170581206396));
#20205=CARTESIAN_POINT('Ctrl Pts',(98.7839409666155,2.19285431426113,-0.254509704886815));
#20206=CARTESIAN_POINT('Ctrl Pts',(98.7667266210241,2.14368442504197,-0.536784875703963));
#20207=CARTESIAN_POINT('Ctrl Pts',(98.7571364971813,2.09877420949042,-0.691869209440657));
#20208=CARTESIAN_POINT('Ctrl Pts',(98.7465535575009,2.02684995392138,-0.866172581729055));
#20209=CARTESIAN_POINT('Ctrl Pts',(98.7450222478677,2.01585928851699,-0.891452243778885));
#20210=CARTESIAN_POINT('Ctrl Pts',(98.7426056485553,1.99757911271466,-0.931430347331973));
#20211=CARTESIAN_POINT('Ctrl Pts',(98.741710075277,1.99059497061757,-0.946264491007038));
#20212=CARTESIAN_POINT('Ctrl Pts',(98.7401304487696,1.97790419169966,-0.972456955810695));
#20213=CARTESIAN_POINT('Ctrl Pts',(98.7394441432905,1.97226366380188,-0.983846315410408));
#20214=CARTESIAN_POINT('Ctrl Pts',(98.7380166524244,1.9602672850207,-1.00755159973478));
#20215=CARTESIAN_POINT('Ctrl Pts',(98.7372761472998,1.95389313765396,-1.01985767316147));
#20216=CARTESIAN_POINT('Ctrl Pts',(98.7353403857479,1.93683527124759,-1.05204297269706));
#20217=CARTESIAN_POINT('Ctrl Pts',(98.734151897556,1.92596142452687,-1.07181991277337));
#20218=CARTESIAN_POINT('Ctrl Pts',(98.7283206558481,1.8706524570423,-1.16885326568765));
#20219=CARTESIAN_POINT('Ctrl Pts',(98.7238369986669,1.82186170150511,-1.24353558743384));
#20220=CARTESIAN_POINT('Ctrl Pts',(98.7147628431058,1.71190018667459,-1.39142688057461));
#20221=CARTESIAN_POINT('Ctrl Pts',(98.7101953754493,1.65023537590249,-1.46403368771191));
#20222=CARTESIAN_POINT('Ctrl Pts',(98.704172438329,1.56377521791967,-1.55340759365115));
#20223=CARTESIAN_POINT('Ctrl Pts',(98.7027548401676,1.54306468148149,-1.5739820312744));
#20224=CARTESIAN_POINT('Ctrl Pts',(98.6970326377795,1.45840561585191,-1.65480750487543));
#20225=CARTESIAN_POINT('Ctrl Pts',(98.6926589087013,1.39129450000088,-1.71161660630004));
#20226=CARTESIAN_POINT('Ctrl Pts',(98.6872432565518,1.30896017292082,-1.77326387038828));
#20227=CARTESIAN_POINT('Ctrl Pts',(98.6864453676975,1.29684857150853,-1.782140635962));
#20228=CARTESIAN_POINT('Ctrl Pts',(98.6851918584676,1.27787389101413,-1.7957516002806));
#20229=CARTESIAN_POINT('Ctrl Pts',(98.6847418784087,1.27107283762284,-1.80057194470799));
#20230=CARTESIAN_POINT('Ctrl Pts',(98.6839033563689,1.25842339944557,-1.80943003554));
#20231=CARTESIAN_POINT('Ctrl Pts',(98.6835155255657,1.2525826443354,-1.81347821060342));
#20232=CARTESIAN_POINT('Ctrl Pts',(98.6826138300427,1.23902470306247,-1.82277835234845));
#20233=CARTESIAN_POINT('Ctrl Pts',(98.6820986217684,1.23129364758351,-1.82800959612674));
#20234=CARTESIAN_POINT('Ctrl Pts',(98.6804403429749,1.20645052773899,-1.84459067694046));
#20235=CARTESIAN_POINT('Ctrl Pts',(98.6792857088648,1.18921346119645,-1.85575023190175));
#20236=CARTESIAN_POINT('Ctrl Pts',(98.6728522086044,1.0933365106662,-1.91593819433007));
#20237=CARTESIAN_POINT('Ctrl Pts',(98.6673455919456,1.01182606062339,-1.96020639111566));
#20238=CARTESIAN_POINT('Ctrl Pts',(98.6517564085217,0.775927256615732,-2.06968069392965));
#20239=CARTESIAN_POINT('Ctrl Pts',(98.6416605152143,0.616515859598225,-2.12263144981644));
#20240=CARTESIAN_POINT('Ctrl Pts',(98.629725095709,0.41112898613636,-2.16573023022504));
#20241=CARTESIAN_POINT('Ctrl Pts',(98.6273486368494,0.369379979564882,-2.17324026584815));
#20242=CARTESIAN_POINT('Ctrl Pts',(98.6240108274908,0.309520200969144,-2.18223315509295));
#20243=CARTESIAN_POINT('Ctrl Pts',(98.6230186967612,0.291569405075992,-2.18470400917741));
#20244=CARTESIAN_POINT('Ctrl Pts',(98.6213367556113,0.260873037841006,-2.18854415190712));
#20245=CARTESIAN_POINT('Ctrl Pts',(98.6206434892773,0.248142467769818,-2.19002410309161));
#20246=CARTESIAN_POINT('Ctrl Pts',(98.619236957212,0.222158312181555,-2.19281532215628));
#20247=CARTESIAN_POINT('Ctrl Pts',(98.6185239993739,0.208904290057733,-2.19411767256596));
#20248=CARTESIAN_POINT('Ctrl Pts',(98.6167488067306,0.175701857908739,-2.19707658185456));
#20249=CARTESIAN_POINT('Ctrl Pts',(98.6156913515618,0.15574094826306,-2.19858168863068));
#20250=CARTESIAN_POINT('Ctrl Pts',(98.6114810564352,0.0755772956097627,
-2.20352899899307));
#20251=CARTESIAN_POINT('Ctrl Pts',(98.6083966205884,0.0152628608045295,
-2.20477205961372));
#20252=CARTESIAN_POINT('Ctrl Pts',(98.6000963612398,-0.150073761844254,
-2.201393329608));
#20253=CARTESIAN_POINT('Ctrl Pts',(98.595014195561,-0.254833118708533,-2.19173820956238));
#20254=CARTESIAN_POINT('Ctrl Pts',(98.5834992921154,-0.489914183120483,
-2.15298336325006));
#20255=CARTESIAN_POINT('Ctrl Pts',(98.5770940579482,-0.619073572472979,
-2.11945590433883));
#20256=CARTESIAN_POINT('Ctrl Pts',(98.5690944463103,-0.763459170958991,
-2.06764505706151));
#20257=CARTESIAN_POINT('Ctrl Pts',(98.5680262147203,-0.782421649149607,
-2.0605441740682));
#20258=CARTESIAN_POINT('Ctrl Pts',(98.5664523187556,-0.809838650084238,
-2.0498443136061));
#20259=CARTESIAN_POINT('Ctrl Pts',(98.5659581996391,-0.81837326267101,-2.04645194081454));
#20260=CARTESIAN_POINT('Ctrl Pts',(98.5650760520444,-0.833474404425227,
-2.04033990570651));
#20261=CARTESIAN_POINT('Ctrl Pts',(98.5646892974171,-0.84004932778919,-2.037641685651));
#20262=CARTESIAN_POINT('Ctrl Pts',(98.5638448545568,-0.854304212247811,
-2.03171103707455));
#20263=CARTESIAN_POINT('Ctrl Pts',(98.563386498473,-0.861978816997602,-2.0284668938879));
#20264=CARTESIAN_POINT('Ctrl Pts',(98.5620725519888,-0.883807706488205,
-2.01909332415812));
#20265=CARTESIAN_POINT('Ctrl Pts',(98.5612109887713,-0.897916020027165,
-2.01285883939544));
#20266=CARTESIAN_POINT('Ctrl Pts',(98.5535751592214,-1.02129427777264,-1.95678258886938));
#20267=CARTESIAN_POINT('Ctrl Pts',(98.546379264091,-1.12637686932969,-1.89823868162809));
#20268=CARTESIAN_POINT('Ctrl Pts',(98.5290866121702,-1.36558190948279,-1.73808934537798));
#20269=CARTESIAN_POINT('Ctrl Pts',(98.5190655536559,-1.49391390694665,-1.62911233654001));
#20270=CARTESIAN_POINT('Ctrl Pts',(98.5081331374325,-1.62715108873485,-1.48685178877377));
#20271=CARTESIAN_POINT('Ctrl Pts',(98.5066297714836,-1.64529206559808,-1.46675254156257));
#20272=CARTESIAN_POINT('Ctrl Pts',(98.5042484333055,-1.67372687560415,-1.43405670389279));
#20273=CARTESIAN_POINT('Ctrl Pts',(98.5033606414264,-1.68425917841203,-1.42167201703516));
#20274=CARTESIAN_POINT('Ctrl Pts',(98.5017898770111,-1.70276727077507,-1.39941439770102));
#20275=CARTESIAN_POINT('Ctrl Pts',(98.5011047377087,-1.71079654173152,-1.38958707432172));
#20276=CARTESIAN_POINT('Ctrl Pts',(98.4996748593877,-1.72745873617371,-1.3688302568602));
#20277=CARTESIAN_POINT('Ctrl Pts',(98.4989308516205,-1.73607386028385,-1.35788715330779));
#20278=CARTESIAN_POINT('Ctrl Pts',(98.496975007594,-1.75857008982103,-1.32874790009838));
#20279=CARTESIAN_POINT('Ctrl Pts',(98.4957702050007,-1.77227268978393,-1.31041570037055));
#20280=CARTESIAN_POINT('Ctrl Pts',(98.48966729184,-1.84082204429818,-1.21566355332151));
#20281=CARTESIAN_POINT('Ctrl Pts',(98.4849479027376,-1.89102417542894,-1.13599903080722));
#20282=CARTESIAN_POINT('Ctrl Pts',(98.4758414440255,-1.9796466965911,-0.97311889189785));
#20283=CARTESIAN_POINT('Ctrl Pts',(98.4714567605868,-2.01827668827651,-0.89023644646018));
#20284=CARTESIAN_POINT('Ctrl Pts',(98.4654624706985,-2.06347430166398,-0.775072277845698));
#20285=CARTESIAN_POINT('Ctrl Pts',(98.4638895505575,-2.07463180192088,-0.744691922107024));
#20286=CARTESIAN_POINT('Ctrl Pts',(98.458229562875,-2.11205466567206,-0.635416623754059));
#20287=CARTESIAN_POINT('Ctrl Pts',(98.4540767898702,-2.13451790430606,-0.555301615725078));
#20288=CARTESIAN_POINT('Ctrl Pts',(98.4489142210089,-2.15560438419302,-0.459573230050325));
#20289=CARTESIAN_POINT('Ctrl Pts',(98.4481226971001,-2.1586606226162,-0.444996749781833));
#20290=CARTESIAN_POINT('Ctrl Pts',(98.4468770938471,-2.16319133042813,-0.422241996652536));
#20291=CARTESIAN_POINT('Ctrl Pts',(98.4464285419477,-2.1647677248158,-0.414084204940365));
#20292=CARTESIAN_POINT('Ctrl Pts',(98.4455948862398,-2.16759507497236,-0.398995232940917));
#20293=CARTESIAN_POINT('Ctrl Pts',(98.4452105112397,-2.16885897862143,-0.392066743442667));
#20294=CARTESIAN_POINT('Ctrl Pts',(98.4443122653992,-2.17172094330413,-0.375940546699376));
#20295=CARTESIAN_POINT('Ctrl Pts',(98.4437970155783,-2.17329379221109,-0.366738648761557));
#20296=CARTESIAN_POINT('Ctrl Pts',(98.4421384610594,-2.17813973675719,-0.337261173484782));
#20297=CARTESIAN_POINT('Ctrl Pts',(98.4409835875036,-2.18118781046561,-0.316950288812622));
#20298=CARTESIAN_POINT('Ctrl Pts',(98.4345474382195,-2.19642817198285,-0.204731309135863));
#20299=CARTESIAN_POINT('Ctrl Pts',(98.4290382202955,-2.2030946212742,-0.112173498256287));
#20300=CARTESIAN_POINT('Ctrl Pts',(98.4134394400837,-2.20539454711444,0.148037288622614));
#20301=CARTESIAN_POINT('Ctrl Pts',(98.4033368297977,-2.18777093699505,0.315203614232164));
#20302=CARTESIAN_POINT('Ctrl Pts',(98.3914031458814,-2.14218503464559,0.520045485017039));
#20303=CARTESIAN_POINT('Ctrl Pts',(98.3890337785581,-2.13181320348286,0.561049766660444));
#20304=CARTESIAN_POINT('Ctrl Pts',(98.3857038047588,-2.11532527181567,0.619146736375997));
#20305=CARTESIAN_POINT('Ctrl Pts',(98.3847126229588,-2.11016860540951,0.636499938029204));
#20306=CARTESIAN_POINT('Ctrl Pts',(98.3830317990227,-2.10099787342105,0.666024101175495));
#20307=CARTESIAN_POINT('Ctrl Pts',(98.3823387122056,-2.09709044444314,0.678226986338901));
#20308=CARTESIAN_POINT('Ctrl Pts',(98.3809321338001,-2.08890376767203,0.703046598009524));
#20309=CARTESIAN_POINT('Ctrl Pts',(98.380218954289,-2.08461609096221,0.715659998599143));
#20310=CARTESIAN_POINT('Ctrl Pts',(98.3784424177545,-2.07359348359208,0.747146288312893));
#20311=CARTESIAN_POINT('Ctrl Pts',(98.3773838561946,-2.0667149745291,0.765967858754301));
#20312=CARTESIAN_POINT('Ctrl Pts',(98.3731625853744,-2.03804429409815,0.841219637864688));
#20313=CARTESIAN_POINT('Ctrl Pts',(98.3700687526667,-2.01418906691081,0.896837915314152));
#20314=CARTESIAN_POINT('Ctrl Pts',(98.3617318569797,-1.94247682190186,1.04668878335903));
#20315=CARTESIAN_POINT('Ctrl Pts',(98.3566240826993,-1.89008695378227,1.13857212896967));
#20316=CARTESIAN_POINT('Ctrl Pts',(98.3451202830752,-1.75764496482616,1.33634837653496));
#20317=CARTESIAN_POINT('Ctrl Pts',(98.3387500363932,-1.67422775834202,1.43947785070547));
#20318=CARTESIAN_POINT('Ctrl Pts',(98.3307919507877,-1.5679816205828,1.54901885236369));
#20319=CARTESIAN_POINT('Ctrl Pts',(98.3297239989432,-1.55368903399983,1.56335411720036));
#20320=CARTESIAN_POINT('Ctrl Pts',(98.3281504435174,-1.53262879165441,1.58390319062292));
#20321=CARTESIAN_POINT('Ctrl Pts',(98.3276563783816,-1.5260161474922,1.59027514656847));
#20322=CARTESIAN_POINT('Ctrl Pts',(98.3267742919527,-1.514215480365,1.6015049143617));
#20323=CARTESIAN_POINT('Ctrl Pts',(98.3263875438814,-1.50904351327845,1.60637921590838));
#20324=CARTESIAN_POINT('Ctrl Pts',(98.3255430713505,-1.49775622519392,1.61691426052723));
#20325=CARTESIAN_POINT('Ctrl Pts',(98.3250846785528,-1.49163244001975,1.62256528226141));
#20326=CARTESIAN_POINT('Ctrl Pts',(98.3237705218262,-1.4740799326161,1.63857937287407));
#20327=CARTESIAN_POINT('Ctrl Pts',(98.3229087821879,-1.46257446558192,1.64885715397298));
#20328=CARTESIAN_POINT('Ctrl Pts',(98.3194014515235,-1.4157177157993,1.68983777408038));
#20329=CARTESIAN_POINT('Ctrl Pts',(98.3166956872643,-1.3795019278426,1.71952964731155));
#20330=CARTESIAN_POINT('Ctrl Pts',(98.3071287479511,-1.25017169014619,1.81884588628619));
#20331=CARTESIAN_POINT('Ctrl Pts',(98.3000805206949,-1.15251785433927,1.88224104938039));
#20332=CARTESIAN_POINT('Ctrl Pts',(98.2851294875688,-0.932783051509522,
2.00135119430274));
#20333=CARTESIAN_POINT('Ctrl Pts',(98.2772965716504,-0.809676421049263,
2.05424547171919));
#20334=CARTESIAN_POINT('Ctrl Pts',(98.2684789473926,-0.659204908025221,
2.10325129947497));
#20335=CARTESIAN_POINT('Ctrl Pts',(98.2671253969096,-0.635766294878183,
2.11045455444487));
#20336=CARTESIAN_POINT('Ctrl Pts',(98.2649962753974,-0.598363214710584,
2.12126973240286));
#20337=CARTESIAN_POINT('Ctrl Pts',(98.2642124174512,-0.584475578760371,
2.12513814281748));
#20338=CARTESIAN_POINT('Ctrl Pts',(98.2627581545978,-0.558494925302232,
2.1321011235284));
#20339=CARTESIAN_POINT('Ctrl Pts',(98.2620866696422,-0.546411704121667,
2.13522973963945));
#20340=CARTESIAN_POINT('Ctrl Pts',(98.2605811568599,-0.519128057805538,
2.14204731434691));
#20341=CARTESIAN_POINT('Ctrl Pts',(98.2597490522509,-0.503913545915732,
2.14567746706132));
#20342=CARTESIAN_POINT('Ctrl Pts',(98.2580330262032,-0.472266649206409,
2.15287317236696));
#20343=CARTESIAN_POINT('Ctrl Pts',(98.257149951911,-0.455829488286515,2.15641326797312));
#20344=CARTESIAN_POINT('Ctrl Pts',(98.2539901320892,-0.396493389044315,
2.16848379443232));
#20345=CARTESIAN_POINT('Ctrl Pts',(98.2517470004201,-0.353382049824391,
2.17592518692529));
#20346=CARTESIAN_POINT('Ctrl Pts',(98.2442924541097,-0.207365264913901,
2.1966743374597));
#20347=CARTESIAN_POINT('Ctrl Pts',(98.2392465740022,-0.103749118601317,
2.20399999999769));
#20348=CARTESIAN_POINT('Ctrl Pts',(98.2342289786285,-4.90931427454822E-11,
2.204));
#20349=CARTESIAN_POINT('Ctrl Pts',(98.1265335566918,1.1079161893468E-10,
2.204));
#20350=CARTESIAN_POINT('Ctrl Pts',(98.1342675812916,-0.129411528099454,
2.20400000000651));
#20351=CARTESIAN_POINT('Ctrl Pts',(98.1418387474841,-0.258588760702719,
2.1926023181208));
#20352=CARTESIAN_POINT('Ctrl Pts',(98.150067141124,-0.403932858849224,2.16674517480458));
#20353=CARTESIAN_POINT('Ctrl Pts',(98.1510734060491,-0.421789255152345,
2.16334007015691));
#20354=CARTESIAN_POINT('Ctrl Pts',(98.15298752015,-0.455908821504527,2.15639515867179));
#20355=CARTESIAN_POINT('Ctrl Pts',(98.1538964368564,-0.472177959630861,
2.15289129538556));
#20356=CARTESIAN_POINT('Ctrl Pts',(98.1554946094833,-0.500898509638879,
2.14636455447198));
#20357=CARTESIAN_POINT('Ctrl Pts',(98.1561862344795,-0.513366032779234,
2.1434167685539));
#20358=CARTESIAN_POINT('Ctrl Pts',(98.1576317495377,-0.539500125647402,
2.1369965891951));
#20359=CARTESIAN_POINT('Ctrl Pts',(98.1583848697209,-0.553160533742675,
2.13350140482032));
#20360=CARTESIAN_POINT('Ctrl Pts',(98.1603699530106,-0.58927581628369,2.12389067266181));
#20361=CARTESIAN_POINT('Ctrl Pts',(98.1615946068978,-0.611669285116579,
2.117550074312));
#20362=CARTESIAN_POINT('Ctrl Pts',(98.1673981307745,-0.718237965388948,
2.08554403079052));
#20363=CARTESIAN_POINT('Ctrl Pts',(98.1718234480369,-0.800929964921452,
2.05520632162096));
#20364=CARTESIAN_POINT('Ctrl Pts',(98.183017280322,-1.0093104866917,1.96426246989302));
#20365=CARTESIAN_POINT('Ctrl Pts',(98.1896086042554,-1.13144832429597,1.89653827803078));
#20366=CARTESIAN_POINT('Ctrl Pts',(98.2000944872558,-1.30696649579322,1.77619046466001));
#20367=CARTESIAN_POINT('Ctrl Pts',(98.2037891419838,-1.36544079150786,1.73164185762113));
#20368=CARTESIAN_POINT('Ctrl Pts',(98.2084392819634,-1.4328695058533,1.67472964239195));
#20369=CARTESIAN_POINT('Ctrl Pts',(98.2092251628545,-1.44406632968273,1.66508462483534));
#20370=CARTESIAN_POINT('Ctrl Pts',(98.2104618405022,-1.461357408337,1.64988439104084));
#20371=CARTESIAN_POINT('Ctrl Pts',(98.2109071797518,-1.46751910980342,1.64440616532635));
#20372=CARTESIAN_POINT('Ctrl Pts',(98.2117469678895,-1.47901285064892,1.63407129713722));
#20373=CARTESIAN_POINT('Ctrl Pts',(98.2121408210175,-1.48435195829846,1.62922290529164));
#20374=CARTESIAN_POINT('Ctrl Pts',(98.213061270069,-1.49671229760999,1.61788741195389));
#20375=CARTESIAN_POINT('Ctrl Pts',(98.2135893117975,-1.50371523724513,1.61138073028224));
#20376=CARTESIAN_POINT('Ctrl Pts',(98.2153467468011,-1.52674259607246,1.58970435823022));
#20377=CARTESIAN_POINT('Ctrl Pts',(98.2165897252916,-1.54258104587969,1.57434003389174));
#20378=CARTESIAN_POINT('Ctrl Pts',(98.2296109696313,-1.70425064945158,1.41272805708928));
#20379=CARTESIAN_POINT('Ctrl Pts',(98.2424133887902,-1.82906894496877,1.24691060655508));
#20380=CARTESIAN_POINT('Ctrl Pts',(98.2594922207184,-1.96994946183549,0.992011775991571));
#20381=CARTESIAN_POINT('Ctrl Pts',(98.2643457288979,-2.0066128547686,0.915584904883031));
#20382=CARTESIAN_POINT('Ctrl Pts',(98.270292549029,-2.04729595690345,0.816514988206113));
#20383=CARTESIAN_POINT('Ctrl Pts',(98.2715254177405,-2.05548648621096,0.795671300483503));
#20384=CARTESIAN_POINT('Ctrl Pts',(98.2735068928136,-2.06824798181319,0.761682224342442));
#20385=CARTESIAN_POINT('Ctrl Pts',(98.2742619909356,-2.07301447571637,0.748612397101283));
#20386=CARTESIAN_POINT('Ctrl Pts',(98.2757075522665,-2.08195077234184,0.723368879750863));
#20387=CARTESIAN_POINT('Ctrl Pts',(98.2763985819378,-2.08613832529582,0.711202117616855));
#20388=CARTESIAN_POINT('Ctrl Pts',(98.2779815135341,-2.09553368901123,0.68310713666743));
#20389=CARTESIAN_POINT('Ctrl Pts',(98.2788709297653,-2.10066690212705,0.667154696577519));
#20390=CARTESIAN_POINT('Ctrl Pts',(98.2817427909987,-2.11675758819062,0.615121989960742));
#20391=CARTESIAN_POINT('Ctrl Pts',(98.2837011133369,-2.12697152891783,0.578817832961619));
#20392=CARTESIAN_POINT('Ctrl Pts',(98.2945026204928,-2.1788408379171,0.374480164961383));
#20393=CARTESIAN_POINT('Ctrl Pts',(98.3027196356053,-2.20151638021777,0.202264551132464));
#20394=CARTESIAN_POINT('Ctrl Pts',(98.3157245974498,-2.20505702532042,-0.0652950997036932));
#20395=CARTESIAN_POINT('Ctrl Pts',(98.3203750544143,-2.20023264076704,-0.159727814560823));
#20396=CARTESIAN_POINT('Ctrl Pts',(98.3263790455512,-2.18697490316926,-0.274206470406807));
#20397=CARTESIAN_POINT('Ctrl Pts',(98.3274753043682,-2.18429054031064,-0.29482738880053));
#20398=CARTESIAN_POINT('Ctrl Pts',(98.3290913257518,-2.17996439454056,-0.324746514266223));
#20399=CARTESIAN_POINT('Ctrl Pts',(98.3295989385246,-2.17855392680965,-0.334077597861353));
#20400=CARTESIAN_POINT('Ctrl Pts',(98.3304986672856,-2.1759649227379,-0.350491377905123));
#20401=CARTESIAN_POINT('Ctrl Pts',(98.3308893715168,-2.1748116417929,-0.357577784837447));
#20402=CARTESIAN_POINT('Ctrl Pts',(98.3317428795821,-2.1722298504236,-0.372967090180427));
#20403=CARTESIAN_POINT('Ctrl Pts',(98.3322063691222,-2.17078837638064,-0.381267351817282));
#20404=CARTESIAN_POINT('Ctrl Pts',(98.3335126844337,-2.16661449004253,-0.40451006723062));
#20405=CARTESIAN_POINT('Ctrl Pts',(98.3343611677306,-2.16377518387219,-0.41943255773293));
#20406=CARTESIAN_POINT('Ctrl Pts',(98.3403770994855,-2.14273173726806,-0.524124657208725));
#20407=CARTESIAN_POINT('Ctrl Pts',(98.3457914881777,-2.11910256302468,-0.6127047896272));
#20408=CARTESIAN_POINT('Ctrl Pts',(98.3525790651776,-2.08309050824252,-0.720297624474304));
#20409=CARTESIAN_POINT('Ctrl Pts',(98.3538915189407,-2.07583726940177,-0.740941530666156));
#20410=CARTESIAN_POINT('Ctrl Pts',(98.3604467504533,-2.03811916092529,-0.84338960349826));
#20411=CARTESIAN_POINT('Ctrl Pts',(98.3656997813867,-2.00311934991906,-0.923444474573782));
#20412=CARTESIAN_POINT('Ctrl Pts',(98.3766987344221,-1.91854314998671,-1.08930524957409));
#20413=CARTESIAN_POINT('Ctrl Pts',(98.382403215317,-1.86774241272555,-1.17428110053408));
#20414=CARTESIAN_POINT('Ctrl Pts',(98.389198556046,-1.79811950705285,-1.27472572596009));
#20415=CARTESIAN_POINT('Ctrl Pts',(98.3904833038852,-1.78453587655683,-1.29367353004006));
#20416=CARTESIAN_POINT('Ctrl Pts',(98.3925270563952,-1.76225270172871,-1.32373730972213));
#20417=CARTESIAN_POINT('Ctrl Pts',(98.3932933207587,-1.75374282170363,-1.33499107796208));
#20418=CARTESIAN_POINT('Ctrl Pts',(98.3947471583142,-1.73730202930718,-1.35630443517149));
#20419=CARTESIAN_POINT('Ctrl Pts',(98.3954354474019,-1.72939036060438,-1.36637807804118));
#20420=CARTESIAN_POINT('Ctrl Pts',(98.3969943124829,-1.7111819669325,-1.38915065226837));
#20421=CARTESIAN_POINT('Ctrl Pts',(98.3978626591386,-1.70083080304664,-1.40180521382827));
#20422=CARTESIAN_POINT('Ctrl Pts',(98.400155687419,-1.67294973430274,-1.43512701230067));
#20423=CARTESIAN_POINT('Ctrl Pts',(98.4015704982026,-1.6551775752626,-1.45558841459629));
#20424=CARTESIAN_POINT('Ctrl Pts',(98.4116766108309,-1.52425221736762,-1.60082557113283));
#20425=CARTESIAN_POINT('Ctrl Pts',(98.4197437546766,-1.39750499458331,-1.7125921598198));
#20426=CARTESIAN_POINT('Ctrl Pts',(98.4336719667384,-1.16138494391914,-1.87697146363944));
#20427=CARTESIAN_POINT('Ctrl Pts',(98.4394849649576,-1.05815698673902,-1.93704262093118));
#20428=CARTESIAN_POINT('Ctrl Pts',(98.4465749215195,-0.936589367455986,
-1.99515845338046));
#20429=CARTESIAN_POINT('Ctrl Pts',(98.4473992943453,-0.922516402084734,
-2.00170436333038));
#20430=CARTESIAN_POINT('Ctrl Pts',(98.4486834078557,-0.900719733283858,
-2.01156421051943));
#20431=CARTESIAN_POINT('Ctrl Pts',(98.4491369934123,-0.893043975208039,
-2.01498363878429));
#20432=CARTESIAN_POINT('Ctrl Pts',(98.4499833236967,-0.878770921557868,
-2.02124448400393));
#20433=CARTESIAN_POINT('Ctrl Pts',(98.4503753567422,-0.872179073368367,
-2.02409763991019));
#20434=CARTESIAN_POINT('Ctrl Pts',(98.451280009738,-0.857011455726024,-2.0305748054557));
#20435=CARTESIAN_POINT('Ctrl Pts',(98.4517939143316,-0.848426563812317,
-2.03417674630099));
#20436=CARTESIAN_POINT('Ctrl Pts',(98.4534571093831,-0.820732479924208,
-2.04559047256281));
#20437=CARTESIAN_POINT('Ctrl Pts',(98.4546181289027,-0.801536799408227,
-2.05318798005866));
#20438=CARTESIAN_POINT('Ctrl Pts',(98.4627764661831,-0.667354874914458,
-2.10412778066878));
#20439=CARTESIAN_POINT('Ctrl Pts',(98.470173957133,-0.549034050412121,-2.13805365291387));
#20440=CARTESIAN_POINT('Ctrl Pts',(98.4842669946737,-0.318918408600111,
-2.18366435939356));
#20441=CARTESIAN_POINT('Ctrl Pts',(98.4909452494111,-0.207821346029025,
-2.19702372319374));
#20442=CARTESIAN_POINT('Ctrl Pts',(98.4998252001992,-0.0543381810846674,
-2.20372813043171));
#20443=CARTESIAN_POINT('Ctrl Pts',(98.5022150687436,-0.0124482554290852,
-2.20436287184061));
#20444=CARTESIAN_POINT('Ctrl Pts',(98.5063633339066,0.0613422884274224,
-2.20337724793752));
#20445=CARTESIAN_POINT('Ctrl Pts',(98.5081360938787,0.0932363403105149,
-2.20225822926894));
#20446=CARTESIAN_POINT('Ctrl Pts',(98.5107587395572,0.140948626565379,-2.19954577131933));
#20447=CARTESIAN_POINT('Ctrl Pts',(98.5116247370679,0.156791253346352,-2.19847325135941));
#20448=CARTESIAN_POINT('Ctrl Pts',(98.5131690767354,0.185196754578092,-2.19624162664492));
#20449=CARTESIAN_POINT('Ctrl Pts',(98.5138493683941,0.197763766157444,-2.19514569505861));
#20450=CARTESIAN_POINT('Ctrl Pts',(98.5153049155017,0.224764591735997,-2.19255727789587));
#20451=CARTESIAN_POINT('Ctrl Pts',(98.5160790447494,0.239194523060699,-2.19103001632704));
#20452=CARTESIAN_POINT('Ctrl Pts',(98.5181506815756,0.277987802607225,-2.18653632580843));
#20453=CARTESIAN_POINT('Ctrl Pts',(98.5194398493154,0.302318776571269,-2.18330523365501));
#20454=CARTESIAN_POINT('Ctrl Pts',(98.5274372040842,0.454300813346942,-2.16053295161724));
#20455=CARTESIAN_POINT('Ctrl Pts',(98.533790594079,0.580086093700449,-2.13021052558156));
#20456=CARTESIAN_POINT('Ctrl Pts',(98.5446281566084,0.7919950490614,-2.05894978114176));
#20457=CARTESIAN_POINT('Ctrl Pts',(98.5491501803657,0.879457511349592,-2.02313714585559));
#20458=CARTESIAN_POINT('Ctrl Pts',(98.5562919479058,1.00985654916164,-1.95968537288833));
#20459=CARTESIAN_POINT('Ctrl Pts',(98.5588195989674,1.05458323501026,-1.93598312938727));
#20460=CARTESIAN_POINT('Ctrl Pts',(98.5624990818,1.11676209727599,-1.9002380042372));
#20461=CARTESIAN_POINT('Ctrl Pts',(98.563594325884,1.13491932265903,-1.88944968940844));
#20462=CARTESIAN_POINT('Ctrl Pts',(98.565559642031,1.16680275306233,-1.86988040901389));
#20463=CARTESIAN_POINT('Ctrl Pts',(98.5664238960406,1.18059206995939,-1.86120491668689));
#20464=CARTESIAN_POINT('Ctrl Pts',(98.5677570591446,1.20148133404075,-1.84773698012256));
#20465=CARTESIAN_POINT('Ctrl Pts',(98.568219051284,1.20865189770259,-1.84305451057076));
#20466=CARTESIAN_POINT('Ctrl Pts',(98.5690726596788,1.22177046123197,-1.83437844136985));
#20467=CARTESIAN_POINT('Ctrl Pts',(98.569463449992,1.22772649176283,-1.8303974932565));
#20468=CARTESIAN_POINT('Ctrl Pts',(98.5703629520683,1.24132292718394,-1.82121356104591));
#20469=CARTESIAN_POINT('Ctrl Pts',(98.5708729105653,1.2489500661958,-1.81599151163634));
#20470=CARTESIAN_POINT('Ctrl Pts',(98.5724813864516,1.2727629960148,-1.79946661263661));
#20471=CARTESIAN_POINT('Ctrl Pts',(98.5735904569145,1.28882948430159,-1.78799447401757));
#20472=CARTESIAN_POINT('Ctrl Pts',(98.5826342482094,1.41723715804116,-1.69367610750241));
#20473=CARTESIAN_POINT('Ctrl Pts',(98.5910899860241,1.52162320203072,-1.60054921876053));
#20474=CARTESIAN_POINT('Ctrl Pts',(98.6084357380205,1.71814274201587,-1.38851083312785));
#20475=CARTESIAN_POINT('Ctrl Pts',(98.6172575115556,1.80837930788489,-1.26876086808271));
#20476=CARTESIAN_POINT('Ctrl Pts',(98.6270056699343,1.89887843463933,-1.11915821190153));
#20477=CARTESIAN_POINT('Ctrl Pts',(98.6284010166433,1.91158402809286,-1.0973153563946));
#20478=CARTESIAN_POINT('Ctrl Pts',(98.630577250089,1.93099870624075,-1.06257753712468));
#20479=CARTESIAN_POINT('Ctrl Pts',(98.6313671430813,1.9379603876628,-1.04982692667709));
#20480=CARTESIAN_POINT('Ctrl Pts',(98.6328409811135,1.95078688807377,-1.02577222605599));
#20481=CARTESIAN_POINT('Ctrl Pts',(98.6335259377552,1.95668075776525,-1.01448438335463));
#20482=CARTESIAN_POINT('Ctrl Pts',(98.6350592026763,1.96971977815122,-0.988975859477251));
#20483=CARTESIAN_POINT('Ctrl Pts',(98.6359055381135,1.97680943560853,-0.974727514930891));
#20484=CARTESIAN_POINT('Ctrl Pts',(98.6383874232418,1.99727270343902,-0.932459972355329));
#20485=CARTESIAN_POINT('Ctrl Pts',(98.6400079185816,2.01020960063278,-0.904233011257104));
#20486=CARTESIAN_POINT('Ctrl Pts',(98.6489161915457,2.07880822623853,-0.745802763263234));
#20487=CARTESIAN_POINT('Ctrl Pts',(98.6557890423879,2.12241915957824,-0.61074300159894));
#20488=CARTESIAN_POINT('Ctrl Pts',(98.6675187849966,2.17443774992763,-0.373700150524359));
#20489=CARTESIAN_POINT('Ctrl Pts',(98.6723843592178,2.18928440543749,-0.273610662932377));
#20490=CARTESIAN_POINT('Ctrl Pts',(98.6790845909202,2.19972608287166,-0.140889251224202));
#20491=CARTESIAN_POINT('Ctrl Pts',(98.6807205305533,2.20154323439667,-0.108866139005686));
#20492=CARTESIAN_POINT('Ctrl Pts',(98.6835495221358,2.20344080942994,-0.0544542376564715));
#20493=CARTESIAN_POINT('Ctrl Pts',(98.6847268049499,2.20388005529775,-0.032082558129561));
#20494=CARTESIAN_POINT('Ctrl Pts',(98.6864405806421,2.20402141575721,6.99580985433863E-6));
#20495=CARTESIAN_POINT('Ctrl Pts',(98.6869627701434,2.20399996797403,0.00972292075741761));
#20496=CARTESIAN_POINT('Ctrl Pts',(98.6878786850192,2.20385068625488,0.0266485667196372));
#20497=CARTESIAN_POINT('Ctrl Pts',(98.688270815811,2.20375171214969,0.0338582872283345));
#20498=CARTESIAN_POINT('Ctrl Pts',(98.6891160501953,2.20346360134124,0.049317817146144));
#20499=CARTESIAN_POINT('Ctrl Pts',(98.6895697138049,2.20326351817185,0.0575669562826086));
#20500=CARTESIAN_POINT('Ctrl Pts',(98.6908228789141,2.20258652479216,0.0802279942411993));
#20501=CARTESIAN_POINT('Ctrl Pts',(98.6916273564445,2.20201450063624,0.0946363922203018));
#20502=CARTESIAN_POINT('Ctrl Pts',(98.6962328716195,2.19796389806364,0.176411710906731));
#20503=CARTESIAN_POINT('Ctrl Pts',(98.7001685095041,2.19153553469335,0.243591567500691));
#20504=CARTESIAN_POINT('Ctrl Pts',(98.7120803409204,2.16324177352094,0.442512598869018));
#20505=CARTESIAN_POINT('Ctrl Pts',(98.7201986022711,2.13247999570725,0.572681161522842));
#20506=CARTESIAN_POINT('Ctrl Pts',(98.7320161394143,2.0690473074637,0.762282136242877));
#20507=CARTESIAN_POINT('Ctrl Pts',(98.735885247166,2.04512656337665,0.824311401617631));
#20508=CARTESIAN_POINT('Ctrl Pts',(98.7422221416428,2.00044362563261,0.926201235584311));
#20509=CARTESIAN_POINT('Ctrl Pts',(98.7447347374067,1.98120151032895,0.966676996040508));
#20510=CARTESIAN_POINT('Ctrl Pts',(98.7482026347796,1.95247538404131,1.02263541791487));
#20511=CARTESIAN_POINT('Ctrl Pts',(98.7491931368884,1.94401491551415,1.03862859535656));
#20512=CARTESIAN_POINT('Ctrl Pts',(98.7508854067987,1.92912050406717,1.06596437707166));
#20513=CARTESIAN_POINT('Ctrl Pts',(98.7515904868767,1.92278116495564,1.0773572175992));
#20514=CARTESIAN_POINT('Ctrl Pts',(98.7530205606184,1.90965181112561,1.10046778410405));
#20515=CARTESIAN_POINT('Ctrl Pts',(98.7537452384513,1.90285413595174,1.11218053037046));
#20516=CARTESIAN_POINT('Ctrl Pts',(98.755565429487,1.88541736165545,1.14159710582605));
#20517=CARTESIAN_POINT('Ctrl Pts',(98.7566557402799,1.87463643993571,1.15921561248863));
#20518=CARTESIAN_POINT('Ctrl Pts',(98.7608459184468,1.83191954736191,1.22687000297117));
#20519=CARTESIAN_POINT('Ctrl Pts',(98.7638805107272,1.79821388078437,1.27576128015598));
#20520=CARTESIAN_POINT('Ctrl Pts',(98.7744506251936,1.67175074234055,1.44421250114368));
#20521=CARTESIAN_POINT('Ctrl Pts',(98.7816221031447,1.56871747569274,1.55551476246047));
#20522=CARTESIAN_POINT('Ctrl Pts',(98.7936205643539,1.38385176687156,1.71801273736785));
#20523=CARTESIAN_POINT('Ctrl Pts',(98.7983214930345,1.30864610294954,1.7759659805567));
#20524=CARTESIAN_POINT('Ctrl Pts',(98.8041125989796,1.21739220972108,1.83733537185422));
#20525=CARTESIAN_POINT('Ctrl Pts',(98.8049169659176,1.20474699581101,1.84565156838166));
#20526=CARTESIAN_POINT('Ctrl Pts',(98.8061764357197,1.18501835980409,1.85833708695035));
#20527=CARTESIAN_POINT('Ctrl Pts',(98.8066257506477,1.17799391539236,1.86279778089008));
#20528=CARTESIAN_POINT('Ctrl Pts',(98.8074686121048,1.16484744764102,1.87104201365884));
#20529=CARTESIAN_POINT('Ctrl Pts',(98.8078615064587,1.15873195854906,1.87483546913788));
#20530=CARTESIAN_POINT('Ctrl Pts',(98.8087739847425,1.14455672275558,1.88353256211609));
#20531=CARTESIAN_POINT('Ctrl Pts',(98.8092949337136,1.13648395243948,1.88841447339648));
#20532=CARTESIAN_POINT('Ctrl Pts',(98.81096009368,1.11073387245209,1.90376161125347));
#20533=CARTESIAN_POINT('Ctrl Pts',(98.8121157764305,1.09294195659972,1.91403130216732));
#20534=CARTESIAN_POINT('Ctrl Pts',(98.8197015382937,0.976467970602844,1.97910790887207));
#20535=CARTESIAN_POINT('Ctrl Pts',(98.8264692785218,0.873849565938286,2.02650950660868));
#20536=CARTESIAN_POINT('Ctrl Pts',(98.8401539050951,0.660335626333366,2.10589222575151));
#20537=CARTESIAN_POINT('Ctrl Pts',(98.8470479344221,0.549632627971197,2.13745950361733));
#20538=CARTESIAN_POINT('Ctrl Pts',(98.8563490584958,0.392518121763679,2.16923995105505));
#20539=CARTESIAN_POINT('Ctrl Pts',(98.8589450720198,0.347801460762961,2.17685713454391));
#20540=CARTESIAN_POINT('Ctrl Pts',(98.8634093806414,0.269309786197768,2.18774697928226));
#20541=CARTESIAN_POINT('Ctrl Pts',(98.8652952713311,0.235636061696432,2.19162962945356));
#20542=CARTESIAN_POINT('Ctrl Pts',(98.8680497044701,0.185699217557624,2.19622311945774));
#20543=CARTESIAN_POINT('Ctrl Pts',(98.8689368360128,0.169497363816221,2.1975329015674));
#20544=CARTESIAN_POINT('Ctrl Pts',(98.8705106482872,0.140547595467022,2.19955116591884));
#20545=CARTESIAN_POINT('Ctrl Pts',(98.8711994524446,0.127805347448724,2.20032833023113));
#20546=CARTESIAN_POINT('Ctrl Pts',(98.8726530943252,0.100765636899738,2.20174182956284));
#20547=CARTESIAN_POINT('Ctrl Pts',(98.8734170096334,0.0864672385194966,
2.20234970599652));
#20548=CARTESIAN_POINT('Ctrl Pts',(98.8754536893319,0.0481177909160257,
2.20360602294779));
#20549=CARTESIAN_POINT('Ctrl Pts',(98.8767184847374,0.0240600261670358,
2.204));
#20550=CARTESIAN_POINT('Ctrl Pts',(98.8779717715633,2.72446158072696E-13,
2.204));
#20551=CARTESIAN_POINT('Origin',(66.9212607628943,0.,0.));
#20552=CARTESIAN_POINT('',(99.7342548474101,-0.00178926204916046,2.20399927371615));
#20553=CARTESIAN_POINT('',(99.6260484068026,-0.00167252030352779,2.20399936539824));
#20554=CARTESIAN_POINT('',(66.9212607628943,-2.69912154532077E-16,2.204));
#20555=CARTESIAN_POINT('Ctrl Pts',(99.7351509568116,-0.00173560988551529,
2.2039993166193));
#20556=CARTESIAN_POINT('Ctrl Pts',(99.7325859424291,0.0411057575387971,
2.20403305342686));
#20557=CARTESIAN_POINT('Ctrl Pts',(99.7300092536942,0.0839392511825805,
2.20281765734755));
#20558=CARTESIAN_POINT('Ctrl Pts',(99.7179214914535,0.284885301152986,2.19124591586051));
#20559=CARTESIAN_POINT('Ctrl Pts',(99.7085400364541,0.44164106551191,2.16510665179586));
#20560=CARTESIAN_POINT('Ctrl Pts',(99.6982903113705,0.618661119182372,2.11554169667784));
#20561=CARTESIAN_POINT('Ctrl Pts',(99.6968906911373,0.642946224384297,2.10828804457973));
#20562=CARTESIAN_POINT('Ctrl Pts',(99.6947133307707,0.680892380503623,2.09623732762893));
#20563=CARTESIAN_POINT('Ctrl Pts',(99.6939264832767,0.694639956523387,2.09172194911354));
#20564=CARTESIAN_POINT('Ctrl Pts',(99.6924615589777,0.720295338562194,2.08301463219413));
#20565=CARTESIAN_POINT('Ctrl Pts',(99.6917824474597,0.732213468258517,2.07885516060639));
#20566=CARTESIAN_POINT('Ctrl Pts',(99.6902665539754,0.758867791840349,2.06929504226411));
#20567=CARTESIAN_POINT('Ctrl Pts',(99.6894316516828,0.773583436864061,2.06383889411998));
#20568=CARTESIAN_POINT('Ctrl Pts',(99.6869973639709,0.81657854801253,2.04737303495592));
#20569=CARTESIAN_POINT('Ctrl Pts',(99.6854122392978,0.844690948101202,2.03593570341873));
#20570=CARTESIAN_POINT('Ctrl Pts',(99.675702382682,1.01732104502677,1.96151088162598));
#20571=CARTESIAN_POINT('Ctrl Pts',(99.6681082105479,1.1549697772068,1.88375071690905));
#20572=CARTESIAN_POINT('Ctrl Pts',(99.6561640965481,1.35566529463431,1.74004067616937));
#20573=CARTESIAN_POINT('Ctrl Pts',(99.6518383342577,1.42495465145616,1.68376731047383));
#20574=CARTESIAN_POINT('Ctrl Pts',(99.6458244657953,1.51264713864155,1.60324896397048));
#20575=CARTESIAN_POINT('Ctrl Pts',(99.6442955464792,1.53424003292068,1.58259785971806));
#20576=CARTESIAN_POINT('Ctrl Pts',(99.6416563138614,1.57014997311557,1.54682841870791));
#20577=CARTESIAN_POINT('Ctrl Pts',(99.6405598584906,1.58468506746144,1.53193415998323));
#20578=CARTESIAN_POINT('Ctrl Pts',(99.6389614448569,1.60527763874894,1.5102260531971));
#20579=CARTESIAN_POINT('Ctrl Pts',(99.6384717809574,1.61150755697306,1.50357654183861));
#20580=CARTESIAN_POINT('Ctrl Pts',(99.6379747759479,1.61774924879298,1.49683111077629));
#20581=CARTESIAN_POINT('Ctrl Pts',(99.6379705318936,1.61780254224925,1.49677351007088));
#20582=CARTESIAN_POINT('Ctrl Pts',(99.6379620191038,1.6179094271203,1.49665797424254));
#20583=CARTESIAN_POINT('Ctrl Pts',(99.6379577503651,1.61796301850719,1.49660003907912));
#20584=CARTESIAN_POINT('Ctrl Pts',(99.6379491869644,1.61807051462472,1.49648381748856));
#20585=CARTESIAN_POINT('Ctrl Pts',(99.6379448922994,1.61812441931998,1.49642553102498));
#20586=CARTESIAN_POINT('Ctrl Pts',(99.637936275772,1.61823255782403,1.49630858955632));
#20587=CARTESIAN_POINT('Ctrl Pts',(99.6379319539071,1.61828679158838,1.4962499345204));
#20588=CARTESIAN_POINT('Ctrl Pts',(99.637539784944,1.62320743882082,1.49092756337933));
#20589=CARTESIAN_POINT('Ctrl Pts',(99.637150012691,1.62804807099266,1.48564022107006));
#20590=CARTESIAN_POINT('Ctrl Pts',(99.6363142056768,1.63831997983979,1.47430989186838));
#20591=CARTESIAN_POINT('Ctrl Pts',(99.6358676563816,1.64374368295239,1.46826043807011));
#20592=CARTESIAN_POINT('Ctrl Pts',(99.6346422525498,1.65845689987352,1.45166600940023));
#20593=CARTESIAN_POINT('Ctrl Pts',(99.6338587137178,1.66767904862106,1.44106212964295));
#20594=CARTESIAN_POINT('Ctrl Pts',(99.6295997589348,1.71685551986327,1.38341341505241));
#20595=CARTESIAN_POINT('Ctrl Pts',(99.6260115858911,1.7549188385564,1.33479743461425));
#20596=CARTESIAN_POINT('Ctrl Pts',(99.6145804532381,1.86766792043124,1.17761794910495));
#20597=CARTESIAN_POINT('Ctrl Pts',(99.6065678819278,1.93469709288563,1.06391543316853));
#20598=CARTESIAN_POINT('Ctrl Pts',(99.5936239071278,2.02828823111083,0.866693440372134));
#20599=CARTESIAN_POINT('Ctrl Pts',(99.5885840933124,2.06076594912135,0.786356740338615));
#20600=CARTESIAN_POINT('Ctrl Pts',(99.5816406607288,2.10005003095095,0.66987076894729));
#20601=CARTESIAN_POINT('Ctrl Pts',(99.5796144997086,2.11081131029522,0.635147867206938));
#20602=CARTESIAN_POINT('Ctrl Pts',(99.5767031442401,2.12523160905694,0.58419380240255));
#20603=CARTESIAN_POINT('Ctrl Pts',(99.5757960109156,2.12957319782394,0.568163539225504));
#20604=CARTESIAN_POINT('Ctrl Pts',(99.5742052488167,2.13691580318684,0.539785391838033));
#20605=CARTESIAN_POINT('Ctrl Pts',(99.5735192186002,2.1399919603836,0.527457901715318));
#20606=CARTESIAN_POINT('Ctrl Pts',(99.5720896931292,2.14621056620963,0.50158696302041));
#20607=CARTESIAN_POINT('Ctrl Pts',(99.5713469061111,2.14933181663506,0.488038963727046));
#20608=CARTESIAN_POINT('Ctrl Pts',(99.5693992846938,2.1572222753737,0.45224510658668));
#20609=CARTESIAN_POINT('Ctrl Pts',(99.5682013655059,2.16177565547391,0.429953076746752));
#20610=CARTESIAN_POINT('Ctrl Pts',(99.5627707661021,2.18101627712602,0.327707053304118));
#20611=CARTESIAN_POINT('Ctrl Pts',(99.5586674260433,2.19161907236155,0.247045592254468));
#20612=CARTESIAN_POINT('Ctrl Pts',(99.5478517573652,2.20809860871596,0.028835408900884));
#20613=CARTESIAN_POINT('Ctrl Pts',(99.5413358282679,2.20559643271538,-0.108969296794327));
#20614=CARTESIAN_POINT('Ctrl Pts',(99.5308421279577,2.18173498617732,-0.321731440484667));
#20615=CARTESIAN_POINT('Ctrl Pts',(99.5270215361818,2.16924261694441,-0.397319970989235));
#20616=CARTESIAN_POINT('Ctrl Pts',(99.5220360869912,2.14881799093012,-0.490459572740548));
#20617=CARTESIAN_POINT('Ctrl Pts',(99.5210424522371,2.14455692231191,-0.508768032697666));
#20618=CARTESIAN_POINT('Ctrl Pts',(99.5195538313485,2.13790748154261,-0.535769362885681));
#20619=CARTESIAN_POINT('Ctrl Pts',(99.5190685437826,2.13569901322567,-0.544506133096103));
#20620=CARTESIAN_POINT('Ctrl Pts',(99.5182333465882,2.13183059202771,-0.559424067266786));
#20621=CARTESIAN_POINT('Ctrl Pts',(99.5178849587174,2.13019720260091,-0.565611913809608));
#20622=CARTESIAN_POINT('Ctrl Pts',(99.5170825168608,2.12639032416238,-0.579783275036138));
#20623=CARTESIAN_POINT('Ctrl Pts',(99.5166274553018,2.12419886150868,-0.587761557840866));
#20624=CARTESIAN_POINT('Ctrl Pts',(99.5153542301126,2.1179753360343,-0.609929571303033));
#20625=CARTESIAN_POINT('Ctrl Pts',(99.51453076822,2.11384572960998,-0.624091189950439));
#20626=CARTESIAN_POINT('Ctrl Pts',(99.5094516320481,2.08771792367807,-0.710455490058696));
#20627=CARTESIAN_POINT('Ctrl Pts',(99.5050275497542,2.06216643813587,-0.781524596915789));
#20628=CARTESIAN_POINT('Ctrl Pts',(99.4927915936766,1.98275900860031,-0.971197098370056));
#20629=CARTESIAN_POINT('Ctrl Pts',(99.4848859747996,1.92195472645178,-1.08657711892708));
#20630=CARTESIAN_POINT('Ctrl Pts',(99.4715815235569,1.79954400286778,-1.27607354707506));
#20631=CARTESIAN_POINT('Ctrl Pts',(99.4660857781109,1.74260860657966,-1.35279017281286));
#20632=CARTESIAN_POINT('Ctrl Pts',(99.4595053801944,1.66602298811145,-1.44309059293132));
#20633=CARTESIAN_POINT('Ctrl Pts',(99.4582405833393,1.65090054788253,-1.46036656141583));
#20634=CARTESIAN_POINT('Ctrl Pts',(99.456226049229,1.62616902483565,-1.48774477199782));
#20635=CARTESIAN_POINT('Ctrl Pts',(99.4554692888896,1.61672951037853,-1.49799729865023));
#20636=CARTESIAN_POINT('Ctrl Pts',(99.4540321275149,1.59851979729358,-1.51740275432467));
#20637=CARTESIAN_POINT('Ctrl Pts',(99.4533510398692,1.58976666534688,-1.52657086970617));
#20638=CARTESIAN_POINT('Ctrl Pts',(99.4518068856642,1.56964290794713,-1.54728788009442));
#20639=CARTESIAN_POINT('Ctrl Pts',(99.4509460232576,1.55822294587838,-1.55878796257449));
#20640=CARTESIAN_POINT('Ctrl Pts',(99.4486699080619,1.52750173988276,-1.58904968357083));
#20641=CARTESIAN_POINT('Ctrl Pts',(99.4472644233843,1.50798161170357,-1.60758576842676));
#20642=CARTESIAN_POINT('Ctrl Pts',(99.4371017744592,1.3629690998057,-1.74032178334487));
#20643=CARTESIAN_POINT('Ctrl Pts',(99.4289805642944,1.22500446514931,-1.84004715217366));
#20644=CARTESIAN_POINT('Ctrl Pts',(99.4151158764487,0.975127467042809,-1.97999080591622));
#20645=CARTESIAN_POINT('Ctrl Pts',(99.4094249065928,0.868941510257868,-2.02883507148214));
#20646=CARTESIAN_POINT('Ctrl Pts',(99.4024281938829,0.743835251543739,-2.0747530252302));
#20647=CARTESIAN_POINT('Ctrl Pts',(99.4015488858329,0.728204136935626,-2.08029077281181));
#20648=CARTESIAN_POINT('Ctrl Pts',(99.4002002192111,0.704404071468602,-2.08842149092379));
#20649=CARTESIAN_POINT('Ctrl Pts',(99.3997381165754,0.696279703642808,-2.09114418176732));
#20650=CARTESIAN_POINT('Ctrl Pts',(99.3988889887552,0.681412270372782,-2.09603040677843));
#20651=CARTESIAN_POINT('Ctrl Pts',(99.398502838266,0.674674410855502,-2.09820889900794));
#20652=CARTESIAN_POINT('Ctrl Pts',(99.3976206321168,0.659333266612976,-2.10308747985607));
#20653=CARTESIAN_POINT('Ctrl Pts',(99.3971234397088,0.650723865382452,-2.1057672591113));
#20654=CARTESIAN_POINT('Ctrl Pts',(99.3955793774784,0.624089670264132,-2.1138785390297));
#20655=CARTESIAN_POINT('Ctrl Pts',(99.3945229962931,0.60601199571494,-2.11913185220807));
#20656=CARTESIAN_POINT('Ctrl Pts',(99.3849132823995,0.442608285957629,-2.16435464434205));
#20657=CARTESIAN_POINT('Ctrl Pts',(99.3757467496148,0.293615410072287,-2.18954746617142));
#20658=CARTESIAN_POINT('Ctrl Pts',(99.3595079860396,0.0231141936463182,
-2.20716342558941));
#20659=CARTESIAN_POINT('Ctrl Pts',(99.3524078570309,-0.097451368274999,
-2.2051336192787));
#20660=CARTESIAN_POINT('Ctrl Pts',(99.3434857745974,-0.25447353019184,-2.18957932716182));
#20661=CARTESIAN_POINT('Ctrl Pts',(99.3413994803973,-0.291588307739401,
-2.18494643120161));
#20662=CARTESIAN_POINT('Ctrl Pts',(99.3384192771659,-0.345170152402561,
-2.17686826236887));
#20663=CARTESIAN_POINT('Ctrl Pts',(99.3375019289786,-0.361742573993451,
-2.17417575140373));
#20664=CARTESIAN_POINT('Ctrl Pts',(99.335899682225,-0.390821999819147,-2.16910953265496));
#20665=CARTESIAN_POINT('Ctrl Pts',(99.335212265111,-0.403342074745187,-2.16681636979938));
#20666=CARTESIAN_POINT('Ctrl Pts',(99.3337859539989,-0.429407694041341,
-2.16180846973057));
#20667=CARTESIAN_POINT('Ctrl Pts',(99.333047703711,-0.442949019142456,-2.15907457162863));
#20668=CARTESIAN_POINT('Ctrl Pts',(99.3311255769567,-0.478328193106123,
-2.15158490610087));
#20669=CARTESIAN_POINT('Ctrl Pts',(99.3299482848148,-0.500121258145158,
-2.14662391770354));
#20670=CARTESIAN_POINT('Ctrl Pts',(99.3247868326121,-0.59613760328773,-2.1232250487795));
#20671=CARTESIAN_POINT('Ctrl Pts',(99.320915995835,-0.669450502817471,-2.10126204626879));
#20672=CARTESIAN_POINT('Ctrl Pts',(99.3101837649922,-0.873322604034533,
-2.02842919451307));
#20673=CARTESIAN_POINT('Ctrl Pts',(99.303549796962,-1.00037455557691,-1.96887464541769));
#20674=CARTESIAN_POINT('Ctrl Pts',(99.2928327941451,-1.18887844144873,-1.85752902671119));
#20675=CARTESIAN_POINT('Ctrl Pts',(99.2889014011253,-1.25462763201251,-1.81376773803157));
#20676=CARTESIAN_POINT('Ctrl Pts',(99.2837807718046,-1.33316726324129,-1.75517654410181));
#20677=CARTESIAN_POINT('Ctrl Pts',(99.2827731359424,-1.34830310705554,-1.74357630628449));
#20678=CARTESIAN_POINT('Ctrl Pts',(99.281267386904,-1.3704091346105,-1.72617408912786));
#20679=CARTESIAN_POINT('Ctrl Pts',(99.2807792906664,-1.37749746539367,-1.72052285924018));
#20680=CARTESIAN_POINT('Ctrl Pts',(99.2799408277803,-1.38953696003429,-1.71080218288318));
#20681=CARTESIAN_POINT('Ctrl Pts',(99.2795920142805,-1.39450554428029,-1.7067546274031));
#20682=CARTESIAN_POINT('Ctrl Pts',(99.2787907594888,-1.40582647840209,-1.69744982244778));
#20683=CARTESIAN_POINT('Ctrl Pts',(99.2783373331855,-1.41216689311513,-1.69217866921574));
#20684=CARTESIAN_POINT('Ctrl Pts',(99.2770738312634,-1.42965802081289,-1.67747051803249));
#20685=CARTESIAN_POINT('Ctrl Pts',(99.2762585891127,-1.44074451834345,-1.6679582143597));
#20686=CARTESIAN_POINT('Ctrl Pts',(99.2713608120757,-1.50623281984018,-1.61062867296098));
#20687=CARTESIAN_POINT('Ctrl Pts',(99.2671231367401,-1.55834096298168,-1.56026717074403));
#20688=CARTESIAN_POINT('Ctrl Pts',(99.2549147374783,-1.69885828811758,-1.41038783220531));
#20689=CARTESIAN_POINT('Ctrl Pts',(99.246829017045,-1.78087797261919,-1.30529296890879));
#20690=CARTESIAN_POINT('Ctrl Pts',(99.2333319654,-1.90478768401034,-1.11291306086762));
#20691=CARTESIAN_POINT('Ctrl Pts',(99.2278145692006,-1.95135609746673,-1.02907954563236));
#20692=CARTESIAN_POINT('Ctrl Pts',(99.2212119786078,-2.00215682157566,-0.921690084339665));
#20693=CARTESIAN_POINT('Ctrl Pts',(99.2199453502669,-2.01166234687263,-0.900754799320084));
#20694=CARTESIAN_POINT('Ctrl Pts',(99.2179282217553,-2.02640652601918,-0.866883605633653));
#20695=CARTESIAN_POINT('Ctrl Pts',(99.2171706810794,-2.03185275045717,-0.854040401531174));
#20696=CARTESIAN_POINT('Ctrl Pts',(99.2157322232877,-2.04201775899832,-0.829421707925496));
#20697=CARTESIAN_POINT('Ctrl Pts',(99.2150506169327,-2.04675751725235,-0.817655534157717));
#20698=CARTESIAN_POINT('Ctrl Pts',(99.2135055197959,-2.05732375478196,-0.790757772653534));
#20699=CARTESIAN_POINT('Ctrl Pts',(99.2126442316379,-2.06308540058328,-0.775601402710669));
#20700=CARTESIAN_POINT('Ctrl Pts',(99.2103674460596,-2.07796668217005,-0.735115728443673));
#20701=CARTESIAN_POINT('Ctrl Pts',(99.2089617078953,-2.08679053812886,-0.709680208431343));
#20702=CARTESIAN_POINT('Ctrl Pts',(99.1988018417313,-2.14778940594839,-0.522860037950963));
#20703=CARTESIAN_POINT('Ctrl Pts',(99.1906825728083,-2.18164661973111,-0.356096556944589));
#20704=CARTESIAN_POINT('Ctrl Pts',(99.1767829080258,-2.20601560498352,-0.0700547651467955));
#20705=CARTESIAN_POINT('Ctrl Pts',(99.1710545462894,-2.20661340458709,0.0475770978464523));
#20706=CARTESIAN_POINT('Ctrl Pts',(99.1640363669841,-2.19663506640115,0.180748442571447));
#20707=CARTESIAN_POINT('Ctrl Pts',(99.1631813709976,-2.19525502677082,0.196801808456324));
#20708=CARTESIAN_POINT('Ctrl Pts',(99.1618623298947,-2.19288063577909,0.221274394690537));
#20709=CARTESIAN_POINT('Ctrl Pts',(99.1614050523952,-2.19201348431048,0.229705725366978));
#20710=CARTESIAN_POINT('Ctrl Pts',(99.1605601976457,-2.19033163130044,0.245180793585658));
#20711=CARTESIAN_POINT('Ctrl Pts',(99.160173429736,-2.18953154718281,0.252225844131779));
#20712=CARTESIAN_POINT('Ctrl Pts',(99.1592837022149,-2.18762229695979,0.268343484563493));
#20713=CARTESIAN_POINT('Ctrl Pts',(99.1587795265824,-2.18649068291347,0.277413098639144));
#20714=CARTESIAN_POINT('Ctrl Pts',(99.1571916195139,-2.18277069590441,0.305790062629107));
#20715=CARTESIAN_POINT('Ctrl Pts',(99.1560976103145,-2.17998280893129,0.325069796837474));
#20716=CARTESIAN_POINT('Ctrl Pts',(99.1468469086964,-2.15451272359991,0.486107664511512));
#20717=CARTESIAN_POINT('Ctrl Pts',(99.1381376724428,-2.11828658929199,0.625366029687957));
#20718=CARTESIAN_POINT('Ctrl Pts',(99.1236133749904,-2.03475895023049,0.852704278170789));
#20719=CARTESIAN_POINT('Ctrl Pts',(99.117755606344,-1.99455432184662,0.942923458206203));
#20720=CARTESIAN_POINT('Ctrl Pts',(99.1087284352821,-1.92129838437821,1.08148029920268));
#20721=CARTESIAN_POINT('Ctrl Pts',(99.1054466027748,-1.89214124788498,1.13171970782923));
#20722=CARTESIAN_POINT('Ctrl Pts',(99.1011428327917,-1.8504478453537,1.19743437449569));
#20723=CARTESIAN_POINT('Ctrl Pts',(99.1000585745337,-1.83963974155745,1.2139736268965));
#20724=CARTESIAN_POINT('Ctrl Pts',(99.0982603048778,-1.82120646433082,1.24136977684593));
#20725=CARTESIAN_POINT('Ctrl Pts',(99.0975417738708,-1.81370318082044,1.25230694769892));
#20726=CARTESIAN_POINT('Ctrl Pts',(99.09613435482,-1.79873561743709,1.27370771933775));
#20727=CARTESIAN_POINT('Ctrl Pts',(99.0954452661879,-1.79127764125888,1.28417506490551));
#20728=CARTESIAN_POINT('Ctrl Pts',(99.0937821950766,-1.7729657063493,1.3094061060183));
#20729=CARTESIAN_POINT('Ctrl Pts',(99.092811873513,-1.76201827139775,1.32410097227892));
#20730=CARTESIAN_POINT('Ctrl Pts',(99.0895380501984,-1.72419963885128,1.37356559870361));
#20731=CARTESIAN_POINT('Ctrl Pts',(99.0872681817162,-1.69647166083457,1.40766867156201));
#20732=CARTESIAN_POINT('Ctrl Pts',(99.0765884854177,-1.55923038431939,1.56651351028985));
#20733=CARTESIAN_POINT('Ctrl Pts',(99.0687159327872,-1.43688426599198,1.67944314635297));
#20734=CARTESIAN_POINT('Ctrl Pts',(99.0561576897297,-1.22866877651398,1.8320717624898));
#20735=CARTESIAN_POINT('Ctrl Pts',(99.0516116482838,-1.15098080309927,1.88184855655554));
#20736=CARTESIAN_POINT('Ctrl Pts',(99.0457394544012,-1.05250742363309,1.93655976450964));
#20737=CARTESIAN_POINT('Ctrl Pts',(99.0446591073866,-1.03446419689044,1.94625778467098));
#20738=CARTESIAN_POINT('Ctrl Pts',(99.0430653062757,-1.00801449624914,1.96000248297032));
#20739=CARTESIAN_POINT('Ctrl Pts',(99.0425636380636,-0.999712865630564,
1.96424976462608));
#20740=CARTESIAN_POINT('Ctrl Pts',(99.0416773830374,-0.985095607952631,
1.97161158148471));
#20741=CARTESIAN_POINT('Ctrl Pts',(99.0412942039352,-0.978791649243712,
1.97474871592414));
#20742=CARTESIAN_POINT('Ctrl Pts',(99.0404543305542,-0.965010640260082,
1.98152456600385));
#20743=CARTESIAN_POINT('Ctrl Pts',(99.039996942569,-0.957528111401297,1.98515114102489));
#20744=CARTESIAN_POINT('Ctrl Pts',(99.0387118491751,-0.936561190004355,
1.99516710842875));
#20745=CARTESIAN_POINT('Ctrl Pts',(99.0378786994663,-0.923032412544451,
2.00146191413888));
#20746=CARTESIAN_POINT('Ctrl Pts',(99.0322980937603,-0.832754303357346,
2.0423574425992));
#20747=CARTESIAN_POINT('Ctrl Pts',(99.0273411984425,-0.754146644769432,
2.07267071416765));
#20748=CARTESIAN_POINT('Ctrl Pts',(99.0203784033333,-0.643087408717639,
2.10834276080852));
#20749=CARTESIAN_POINT('Ctrl Pts',(99.0184303972988,-0.611953003980711,
2.11758921622595));
#20750=CARTESIAN_POINT('Ctrl Pts',(99.0109245910529,-0.491393010644367,
2.15051279165374));
#20751=CARTESIAN_POINT('Ctrl Pts',(99.0053620417862,-0.400710246579317,
2.16924068346033));
#20752=CARTESIAN_POINT('Ctrl Pts',(98.9963212997439,-0.248652954517391,
2.19077996224226));
#20753=CARTESIAN_POINT('Ctrl Pts',(98.9927797481123,-0.187856803092223,
2.19682859171664));
#20754=CARTESIAN_POINT('Ctrl Pts',(98.9869169066235,-0.0848271257078374,
2.20276985289966));
#20755=CARTESIAN_POINT('Ctrl Pts',(98.9845588362986,-0.0427074822583268,
2.20398890193156));
#20756=CARTESIAN_POINT('Ctrl Pts',(98.9822274881864,-0.000384419624161417,
2.20399997485622));
#20757=CARTESIAN_POINT('Ctrl Pts',(98.982216901173,-0.000192209799753219,
2.204));
#20758=CARTESIAN_POINT('Ctrl Pts',(98.9822063149447,-3.98666500548274E-14,
2.204));
#20759=CARTESIAN_POINT('Ctrl Pts',(98.8779717715633,2.72446158072696E-13,
2.204));
#20760=CARTESIAN_POINT('Ctrl Pts',(98.8779819576879,-0.000195548552893731,
2.204));
#20761=CARTESIAN_POINT('Ctrl Pts',(98.8779921430541,-0.000391097255348482,
2.20399997397511));
#20762=CARTESIAN_POINT('Ctrl Pts',(98.8842321210603,-0.120201351076194,
2.20396808367526));
#20763=CARTESIAN_POINT('Ctrl Pts',(98.8901497521798,-0.239620005710135,
2.19419922271989));
#20764=CARTESIAN_POINT('Ctrl Pts',(98.8996566185453,-0.432634550292262,
2.16245589655867));
#20765=CARTESIAN_POINT('Ctrl Pts',(98.903304935187,-0.506913965546811,2.14625867285324));
#20766=CARTESIAN_POINT('Ctrl Pts',(98.9119661043065,-0.678794290353091,
2.09935638758593));
#20767=CARTESIAN_POINT('Ctrl Pts',(98.9170040688667,-0.775380083419822,
2.06563312797774));
#20768=CARTESIAN_POINT('Ctrl Pts',(98.9231841836035,-0.883295505522182,
2.019316246659));
#20769=CARTESIAN_POINT('Ctrl Pts',(98.9239950325058,-0.897260777253245,
2.01314980216912));
#20770=CARTESIAN_POINT('Ctrl Pts',(98.9252673157792,-0.918846802374575,
2.00334914883852));
#20771=CARTESIAN_POINT('Ctrl Pts',(98.92572290691,-0.926512888221899,1.9998152718533));
#20772=CARTESIAN_POINT('Ctrl Pts',(98.9265709205397,-0.940659383164747,
1.99319528479629));
#20773=CARTESIAN_POINT('Ctrl Pts',(98.9269626037561,-0.947145236154838,
1.9901214574628));
#20774=CARTESIAN_POINT('Ctrl Pts',(98.9278724512557,-0.962101596949523,
1.98294354646419));
#20775=CARTESIAN_POINT('Ctrl Pts',(98.9283919741667,-0.970560919166227,
1.9788168401509));
#20776=CARTESIAN_POINT('Ctrl Pts',(98.9300616107466,-0.997501306033836,
1.96546022223597));
#20777=CARTESIAN_POINT('Ctrl Pts',(98.9312234054895,-1.01587863170852,1.95602486780533));
#20778=CARTESIAN_POINT('Ctrl Pts',(98.9376892954594,-1.11632936092291,1.90265368074079));
#20779=CARTESIAN_POINT('Ctrl Pts',(98.9432226407972,-1.1956824255753,1.85381309047381));
#20780=CARTESIAN_POINT('Ctrl Pts',(98.9589291016104,-1.40966150824606,1.70264552509731));
#20781=CARTESIAN_POINT('Ctrl Pts',(98.9691119368599,-1.53598059806489,1.5896308996929));
#20782=CARTESIAN_POINT('Ctrl Pts',(98.9810240701708,-1.67524180850678,1.43277538891879));
#20783=CARTESIAN_POINT('Ctrl Pts',(98.9833079878426,-1.70147696633201,1.40151948841479));
#20784=CARTESIAN_POINT('Ctrl Pts',(98.9864485502119,-1.73688220248456,1.35687798770791));
#20785=CARTESIAN_POINT('Ctrl Pts',(98.9873345971617,-1.74679413978557,1.34409371390439));
#20786=CARTESIAN_POINT('Ctrl Pts',(98.9888647915214,-1.76377424421074,1.32168789717984));
#20787=CARTESIAN_POINT('Ctrl Pts',(98.9895114474958,-1.77090655545369,1.31211602452172));
#20788=CARTESIAN_POINT('Ctrl Pts',(98.9908582271073,-1.78566753173705,1.29196653580043));
#20789=CARTESIAN_POINT('Ctrl Pts',(98.9915577371709,-1.79328080062611,1.28137818138705));
#20790=CARTESIAN_POINT('Ctrl Pts',(98.9932202075996,-1.81124245128677,1.25592389799731));
#20791=CARTESIAN_POINT('Ctrl Pts',(98.9941797726967,-1.82150252313242,1.24099663149863));
#20792=CARTESIAN_POINT('Ctrl Pts',(98.9974966396391,-1.8565740887023,1.18859922961264));
#20793=CARTESIAN_POINT('Ctrl Pts',(98.9998182233471,-1.88042351248254,1.15049695738275));
#20794=CARTESIAN_POINT('Ctrl Pts',(99.0054981585673,-1.93675014652145,1.05407191048516));
#20795=CARTESIAN_POINT('Ctrl Pts',(99.0088097243281,-1.96777520661731,0.994952393247454));
#20796=CARTESIAN_POINT('Ctrl Pts',(99.0188405630806,-2.0546537273671,0.809384478300428));
#20797=CARTESIAN_POINT('Ctrl Pts',(99.0253749846822,-2.10133742770108,0.679031032695808));
#20798=CARTESIAN_POINT('Ctrl Pts',(99.0353464024369,-2.15103009635578,0.48437818857596));
#20799=CARTESIAN_POINT('Ctrl Pts',(99.0385261031426,-2.16394569212151,0.422954470608338));
#20800=CARTESIAN_POINT('Ctrl Pts',(99.0425836191876,-2.17654692845008,0.347074506286445));
#20801=CARTESIAN_POINT('Ctrl Pts',(99.0433384786084,-2.17873572578328,0.333058344683618));
#20802=CARTESIAN_POINT('Ctrl Pts',(99.0445411329203,-2.18197573696531,0.310910116796425));
#20803=CARTESIAN_POINT('Ctrl Pts',(99.0449840590829,-2.18311716929175,0.302791410289721));
#20804=CARTESIAN_POINT('Ctrl Pts',(99.0458220622702,-2.18517895953167,0.287508413564723));
#20805=CARTESIAN_POINT('Ctrl Pts',(99.0462165783078,-2.18610942786841,0.280345745517549));
#20806=CARTESIAN_POINT('Ctrl Pts',(99.0471516433973,-2.18822079192894,0.263442661046369));
#20807=CARTESIAN_POINT('Ctrl Pts',(99.0476938144531,-2.18937187214884,0.253698773852814));
#20808=CARTESIAN_POINT('Ctrl Pts',(99.0495145460236,-2.19299657066233,0.221151843992155));
#20809=CARTESIAN_POINT('Ctrl Pts',(99.0508078202551,-2.19517920330723,0.19831862700156));
#20810=CARTESIAN_POINT('Ctrl Pts',(99.0540072349077,-2.19964503383976,0.142399042751306));
#20811=CARTESIAN_POINT('Ctrl Pts',(99.0559290812575,-2.20153850050353,0.109287679370813));
#20812=CARTESIAN_POINT('Ctrl Pts',(99.0641816120771,-2.20640466801385,-0.0314732378845199));
#20813=CARTESIAN_POINT('Ctrl Pts',(99.0706952879823,-2.20223274059584,-0.139218919484558));
#20814=CARTESIAN_POINT('Ctrl Pts',(99.0851133559994,-2.17536224171632,-0.378235751407745));
#20815=CARTESIAN_POINT('Ctrl Pts',(99.0929473820982,-2.14861512900064,-0.508650222839978));
#20816=CARTESIAN_POINT('Ctrl Pts',(99.102166015032,-2.10128187895847,-0.665734914531923));
#20817=CARTESIAN_POINT('Ctrl Pts',(99.1038983440931,-2.09165165097905,-0.69540062029428));
#20818=CARTESIAN_POINT('Ctrl Pts',(99.1064851959957,-2.07615150258665,-0.739908849775325));
#20819=CARTESIAN_POINT('Ctrl Pts',(99.1073548213281,-2.07074497912298,-0.754907555892946));
#20820=CARTESIAN_POINT('Ctrl Pts',(99.1089094067156,-2.06072749829178,-0.781780263840039));
#20821=CARTESIAN_POINT('Ctrl Pts',(99.109596293608,-2.05617549147496,-0.793675349811464));
#20822=CARTESIAN_POINT('Ctrl Pts',(99.1110582322353,-2.04621836449682,-0.819034105401334));
#20823=CARTESIAN_POINT('Ctrl Pts',(99.1118322246287,-2.04078288271679,-0.832485255348903));
#20824=CARTESIAN_POINT('Ctrl Pts',(99.1139373156913,-2.02555278680329,-0.86912927747891));
#20825=CARTESIAN_POINT('Ctrl Pts',(99.1152594034335,-2.01549282940701,-0.892209905891794));
#20826=CARTESIAN_POINT('Ctrl Pts',(99.1244799731463,-1.94188981603775,-1.05347612791501));
#20827=CARTESIAN_POINT('Ctrl Pts',(99.1318691014482,-1.86458794870026,-1.18493281352967));
#20828=CARTESIAN_POINT('Ctrl Pts',(99.1458398045079,-1.69312843659415,-1.41763293459058));
#20829=CARTESIAN_POINT('Ctrl Pts',(99.1524119494182,-1.60181207777976,-1.52005152776948));
#20830=CARTESIAN_POINT('Ctrl Pts',(99.1605947889176,-1.48701358716537,-1.62689999990013));
#20831=CARTESIAN_POINT('Ctrl Pts',(99.1616464037074,-1.47224536783317,-1.64027636091257));
#20832=CARTESIAN_POINT('Ctrl Pts',(99.1632083426155,-1.45033801598461,-1.65958480320958));
#20833=CARTESIAN_POINT('Ctrl Pts',(99.1637076312617,-1.44333914665913,-1.66567529281758));
#20834=CARTESIAN_POINT('Ctrl Pts',(99.1645983681987,-1.43086618238342,-1.67639175945168));
#20835=CARTESIAN_POINT('Ctrl Pts',(99.1649885095893,-1.42540769294651,-1.68103547555347));
#20836=CARTESIAN_POINT('Ctrl Pts',(99.1658478541629,-1.41339597419302,-1.69115366830288));
#20837=CARTESIAN_POINT('Ctrl Pts',(99.1663178239071,-1.406833633168,-1.69661664298097));
#20838=CARTESIAN_POINT('Ctrl Pts',(99.1676851706642,-1.38775448027841,-1.71231273126592));
#20839=CARTESIAN_POINT('Ctrl Pts',(99.1685892007942,-1.3751568593507,-1.72244621630854));
#20840=CARTESIAN_POINT('Ctrl Pts',(99.1765817214468,-1.26380584234128,-1.81001641985096));
#20841=CARTESIAN_POINT('Ctrl Pts',(99.1841231591728,-1.15872518919438,-1.87901975974689));
#20842=CARTESIAN_POINT('Ctrl Pts',(99.2012714431274,-0.907653207599422,
-2.01478731211538));
#20843=CARTESIAN_POINT('Ctrl Pts',(99.210799976273,-0.75906405892106,-2.07534069296284));
#20844=CARTESIAN_POINT('Ctrl Pts',(99.2213374367414,-0.578569263933788,
-2.12688534314843));
#20845=CARTESIAN_POINT('Ctrl Pts',(99.2228770172868,-0.551785818500878,
-2.13399066658404));
#20846=CARTESIAN_POINT('Ctrl Pts',(99.2253087049501,-0.508829510245894,
-2.1445235959848));
#20847=CARTESIAN_POINT('Ctrl Pts',(99.2262111736437,-0.492740372365689,
-2.14827741938747));
#20848=CARTESIAN_POINT('Ctrl Pts',(99.2278043178493,-0.46408128644873,-2.15462507986063));
#20849=CARTESIAN_POINT('Ctrl Pts',(99.2284972652143,-0.451528165025448,
-2.15729066217659));
#20850=CARTESIAN_POINT('Ctrl Pts',(99.2299400761059,-0.425210908550469,
-2.16263919968189));
#20851=CARTESIAN_POINT('Ctrl Pts',(99.2306892282524,-0.41144297862788,-2.16530074413299));
#20852=CARTESIAN_POINT('Ctrl Pts',(99.2326514265378,-0.375117604198007,
-2.17196399415345));
#20853=CARTESIAN_POINT('Ctrl Pts',(99.2338574720032,-0.35252124637108,-2.17574576451316));
#20854=CARTESIAN_POINT('Ctrl Pts',(99.2398629922906,-0.238735833485533,
-2.19296986908662));
#20855=CARTESIAN_POINT('Ctrl Pts',(99.2444916252348,-0.146821960262342,
-2.20103552636029));
#20856=CARTESIAN_POINT('Ctrl Pts',(99.2535541043797,0.0374940970157028,
-2.20560848221647));
#20857=CARTESIAN_POINT('Ctrl Pts',(99.2579794673787,0.12970755991788,-2.2021105504077));
#20858=CARTESIAN_POINT('Ctrl Pts',(99.2639834222332,0.253022134079523,-2.18965841913081));
#20859=CARTESIAN_POINT('Ctrl Pts',(99.2655261100552,0.284540510739411,-2.18578609166718));
#20860=CARTESIAN_POINT('Ctrl Pts',(99.2712230416771,0.399692601715817,-2.16910567812424));
#20861=CARTESIAN_POINT('Ctrl Pts',(99.2754437726786,0.482645989649669,-2.15216721563663));
#20862=CARTESIAN_POINT('Ctrl Pts',(99.2806886967422,0.578937725767128,-2.12665768714003));
#20863=CARTESIAN_POINT('Ctrl Pts',(99.2814871561207,0.593423439896998,-2.12266116113004));
#20864=CARTESIAN_POINT('Ctrl Pts',(99.2827440493808,0.615929641385201,-2.11620344938766));
#20865=CARTESIAN_POINT('Ctrl Pts',(99.2831968624445,0.623979118265158,-2.11384399083369));
#20866=CARTESIAN_POINT('Ctrl Pts',(99.2840388188358,0.638832492234408,-2.10939794549622));
#20867=CARTESIAN_POINT('Ctrl Pts',(99.2844272230258,0.64563998150957,-2.10732428810101));
#20868=CARTESIAN_POINT('Ctrl Pts',(99.2853358729685,0.66146378946655,-2.10242026217501));
#20869=CARTESIAN_POINT('Ctrl Pts',(99.2858575381223,0.670472045502456,-2.09956484373857));
#20870=CARTESIAN_POINT('Ctrl Pts',(99.2875412215263,0.699314028067557,-2.09021802805107));
#20871=CARTESIAN_POINT('Ctrl Pts',(99.2887151898155,0.719073464730478,-2.08350301228916));
#20872=CARTESIAN_POINT('Ctrl Pts',(99.295316449121,0.828450962499218,-2.04459113268242));
#20873=CARTESIAN_POINT('Ctrl Pts',(99.3009828637042,0.915998318586846,-2.00689512132065));
#20874=CARTESIAN_POINT('Ctrl Pts',(99.3172181314714,1.15717691270074,-1.88397276347889));
#20875=CARTESIAN_POINT('Ctrl Pts',(99.3277801425298,1.30347842475317,-1.7858819131866));
#20876=CARTESIAN_POINT('Ctrl Pts',(99.3396657381627,1.46319571246208,-1.64860662951125));
#20877=CARTESIAN_POINT('Ctrl Pts',(99.341619693369,1.4892395080735,-1.62511888747566));
#20878=CARTESIAN_POINT('Ctrl Pts',(99.3444567846536,1.52672317447922,-1.58965584656953));
#20879=CARTESIAN_POINT('Ctrl Pts',(99.3453599997491,1.53860545699172,-1.57815798663196));
#20880=CARTESIAN_POINT('Ctrl Pts',(99.3469539204563,1.55947877360995,-1.55750012597765));
#20881=CARTESIAN_POINT('Ctrl Pts',(99.3476469072359,1.56852119369887,-1.54839334873592));
#20882=CARTESIAN_POINT('Ctrl Pts',(99.3490892662852,1.58726989598803,-1.52917841962006));
#20883=CARTESIAN_POINT('Ctrl Pts',(99.3498379329853,1.5969603733939,-1.51905560792957));
#20884=CARTESIAN_POINT('Ctrl Pts',(99.3517976503572,1.62221077610405,-1.49216998298958));
#20885=CARTESIAN_POINT('Ctrl Pts',(99.3530017309911,1.63760767651869,-1.47525598113192));
#20886=CARTESIAN_POINT('Ctrl Pts',(99.358976117133,1.71334395391468,-1.38941010806373));
#20887=CARTESIAN_POINT('Ctrl Pts',(99.363577808431,1.76961037487185,-1.31700017842805));
#20888=CARTESIAN_POINT('Ctrl Pts',(99.3726313178278,1.87331675995762,-1.16484322800207));
#20889=CARTESIAN_POINT('Ctrl Pts',(99.3770725948651,1.92055784933156,-1.08518815601464));
#20890=CARTESIAN_POINT('Ctrl Pts',(99.3830480279422,1.97668631848116,-0.975335051929698));
#20891=CARTESIAN_POINT('Ctrl Pts',(99.3845462431251,1.9901411877012,-0.947578636071126));
#20892=CARTESIAN_POINT('Ctrl Pts',(99.3902522214846,2.03879171915261,-0.841605588752568));
#20893=CARTESIAN_POINT('Ctrl Pts',(99.3945274541168,2.06999107473806,-0.761646736059623));
#20894=CARTESIAN_POINT('Ctrl Pts',(99.3998348007729,2.10109643283176,-0.665760092312499));
#20895=CARTESIAN_POINT('Ctrl Pts',(99.4006348303378,2.10559558692611,-0.651390758415191));
#20896=CARTESIAN_POINT('Ctrl Pts',(99.4018936496943,2.11237312583705,-0.62894057343521));
#20897=CARTESIAN_POINT('Ctrl Pts',(99.4023467897566,2.11475324358211,-0.620890635859239));
#20898=CARTESIAN_POINT('Ctrl Pts',(99.4031890129687,2.11906576994465,-0.60599248641347));
#20899=CARTESIAN_POINT('Ctrl Pts',(99.4035773523723,2.12101107036898,-0.599148283538529));
#20900=CARTESIAN_POINT('Ctrl Pts',(99.4044853688258,2.12546003187099,-0.583202164515569));
#20901=CARTESIAN_POINT('Ctrl Pts',(99.4050064587185,2.12793838633418,-0.574093484588346));
#20902=CARTESIAN_POINT('Ctrl Pts',(99.4066862787295,2.13569264993574,-0.544854095496048));
#20903=CARTESIAN_POINT('Ctrl Pts',(99.4078568838098,2.14074183689371,-0.52466503972739));
#20904=CARTESIAN_POINT('Ctrl Pts',(99.4144201731322,2.16716039172308,-0.412293530731154));
#20905=CARTESIAN_POINT('Ctrl Pts',(99.4200491857681,2.1828601388763,-0.318886838354072));
#20906=CARTESIAN_POINT('Ctrl Pts',(99.4361336124783,2.21021298531451,-0.0520739424175816));
#20907=CARTESIAN_POINT('Ctrl Pts',(99.4465872133594,2.20745394026298,0.122138351323359));
#20908=CARTESIAN_POINT('Ctrl Pts',(99.4585115445208,2.17929807565128,0.331155146551179));
#20909=CARTESIAN_POINT('Ctrl Pts',(99.4605898495478,2.17338922909748,0.367944738699607));
#20910=CARTESIAN_POINT('Ctrl Pts',(99.4635562891413,2.16348856676216,0.42096488780234));
#20911=CARTESIAN_POINT('Ctrl Pts',(99.464467723569,2.16024071916095,0.437326276531178));
#20912=CARTESIAN_POINT('Ctrl Pts',(99.4660711257746,2.15416131875394,0.466229856064673));
#20913=CARTESIAN_POINT('Ctrl Pts',(99.4667654650416,2.151405198076,0.478786956148474));
#20914=CARTESIAN_POINT('Ctrl Pts',(99.4682057617156,2.14543025095464,0.504915394254023));
#20915=CARTESIAN_POINT('Ctrl Pts',(99.4689510653189,2.14219214557338,0.518481765128088));
#20916=CARTESIAN_POINT('Ctrl Pts',(99.4708911349949,2.13338026716489,0.553907475462395));
#20917=CARTESIAN_POINT('Ctrl Pts',(99.4720791932562,2.12759922226144,0.575713865483944));
#20918=CARTESIAN_POINT('Ctrl Pts',(99.4777977009217,2.09791120601089,0.68113684055803));
#20919=CARTESIAN_POINT('Ctrl Pts',(99.4821774472969,2.0694033087223,0.763381215537553));
#20920=CARTESIAN_POINT('Ctrl Pts',(99.4912235733024,1.99914849607456,0.932921154614271));
#20921=CARTESIAN_POINT('Ctrl Pts',(99.4958580202553,1.95636899547256,1.01958688724714));
#20922=CARTESIAN_POINT('Ctrl Pts',(99.5058109138713,1.85350152980109,1.19750692642425));
#20923=CARTESIAN_POINT('Ctrl Pts',(99.5111277827863,1.79204179445364,1.28766154482144));
#20924=CARTESIAN_POINT('Ctrl Pts',(99.5178745450657,1.71137199444857,1.38897242947922));
#20925=CARTESIAN_POINT('Ctrl Pts',(99.5189579953094,1.69834413657979,1.40487211067572));
#20926=CARTESIAN_POINT('Ctrl Pts',(99.5205606481797,1.67901355583851,1.42780199591138));
#20927=CARTESIAN_POINT('Ctrl Pts',(99.52106807592,1.67288466564146,1.4349780308815));
#20928=CARTESIAN_POINT('Ctrl Pts',(99.5219684751114,1.66199987406497,1.44755802557908));
#20929=CARTESIAN_POINT('Ctrl Pts',(99.5223600459261,1.65726330998197,1.45297836838577));
#20930=CARTESIAN_POINT('Ctrl Pts',(99.5231793752735,1.64734794823736,1.46421356525199));
#20931=CARTESIAN_POINT('Ctrl Pts',(99.5236074163515,1.64216494102976,1.47002412560153));
#20932=CARTESIAN_POINT('Ctrl Pts',(99.5247752621424,1.62801226807455,1.48572213813831));
#20933=CARTESIAN_POINT('Ctrl Pts',(99.5255192598734,1.61898352231481,1.49555560019222));
#20934=CARTESIAN_POINT('Ctrl Pts',(99.5272304205214,1.59817406593917,1.51781050192986));
#20935=CARTESIAN_POINT('Ctrl Pts',(99.5282012129174,1.58633693607812,1.5301778185648));
#20936=CARTESIAN_POINT('Ctrl Pts',(99.5312920955836,1.54850703200064,1.5687913870468));
#20937=CARTESIAN_POINT('Ctrl Pts',(99.5334409204209,1.52199870138607,1.59452191586549));
#20938=CARTESIAN_POINT('Ctrl Pts',(99.5433514506028,1.39819764812139,1.70878966785774));
#20939=CARTESIAN_POINT('Ctrl Pts',(99.5513545933414,1.2937457944548,1.78917329854906));
#20940=CARTESIAN_POINT('Ctrl Pts',(99.5659789050298,1.0862732507725,1.92111907342853));
#20941=CARTESIAN_POINT('Ctrl Pts',(99.5726243078922,0.985159774363577,1.97488086049082));
#20942=CARTESIAN_POINT('Ctrl Pts',(99.5803630711005,0.857787132007931,2.03037465604049));
#20943=CARTESIAN_POINT('Ctrl Pts',(99.5817193351804,0.835092880834106,2.03981370648384));
#20944=CARTESIAN_POINT('Ctrl Pts',(99.5838489547668,0.798874975052813,2.05417176014373));
#20945=CARTESIAN_POINT('Ctrl Pts',(99.5846306781474,0.785453347338186,2.05934113222772));
#20946=CARTESIAN_POINT('Ctrl Pts',(99.5860285485871,0.761227520663636,2.06840046675538));
#20947=CARTESIAN_POINT('Ctrl Pts',(99.5866462688971,0.750441789841577,2.07233804097646));
#20948=CARTESIAN_POINT('Ctrl Pts',(99.5880924270923,0.725005104672771,2.08139964592174));
#20949=CARTESIAN_POINT('Ctrl Pts',(99.5889185159181,0.710329718981657,2.08645359280059));
#20950=CARTESIAN_POINT('Ctrl Pts',(99.5913304252522,0.667067653094773,2.10084293183861));
#20951=CARTESIAN_POINT('Ctrl Pts',(99.5929021761282,0.638341314950516,2.10974897988092));
#20952=CARTESIAN_POINT('Ctrl Pts',(99.6001030646095,0.504450129678244,2.14827412387405));
#20953=CARTESIAN_POINT('Ctrl Pts',(99.6054993738531,0.397352364815328,2.17063722383543));
#20954=CARTESIAN_POINT('Ctrl Pts',(99.6155366188792,0.192633336516848,2.19771779147581));
#20955=CARTESIAN_POINT('Ctrl Pts',(99.6201868564507,0.0955024069012108,
2.20407547326078));
#20956=CARTESIAN_POINT('Ctrl Pts',(99.6249543031017,-0.00172616788486746,
2.20399932403448));
#20957=CARTESIAN_POINT('Origin',(88.3562164250559,0.,0.));
#20958=CARTESIAN_POINT('',(90.9367078804582,1.77561363837197,-0.0475422940912709));
#20959=CARTESIAN_POINT('',(90.7899230490922,1.77530581490221,-0.0474953858958096));
#20960=CARTESIAN_POINT('',(88.3562164250559,1.77561363837197,-0.0475422940912398));
#20961=CARTESIAN_POINT('',(90.3498698986825,0.408169026503128,1.72871689651704));
#20962=CARTESIAN_POINT('Ctrl Pts',(90.9367078804582,1.77561363837197,-0.047542294091302));
#20963=CARTESIAN_POINT('Ctrl Pts',(90.9366940428792,1.77560821463806,-0.0477448601658868));
#20964=CARTESIAN_POINT('Ctrl Pts',(90.9366802071354,1.77560275623504,-0.0479474255107499));
#20965=CARTESIAN_POINT('Ctrl Pts',(90.9362063763554,1.77541461075793,-0.0548855493489321));
#20966=CARTESIAN_POINT('Ctrl Pts',(90.9357484215827,1.77519362986983,-0.0616201586282712));
#20967=CARTESIAN_POINT('Ctrl Pts',(90.9347807730013,1.77464311481225,-0.0759153772536121));
#20968=CARTESIAN_POINT('Ctrl Pts',(90.9342716652679,1.7743035754535,-0.0834754835775824));
#20969=CARTESIAN_POINT('Ctrl Pts',(90.932978732698,1.77331355919584,-0.102767374601682));
#20970=CARTESIAN_POINT('Ctrl Pts',(90.9321985825354,1.77259496333718,-0.114495532509192));
#20971=CARTESIAN_POINT('Ctrl Pts',(90.9288988399027,1.76903793233093,-0.164427403387343));
#20972=CARTESIAN_POINT('Ctrl Pts',(90.9264340184423,1.7650801781021,-0.202543892264564));
#20973=CARTESIAN_POINT('Ctrl Pts',(90.9192199515912,1.74966032069272,-0.315378249871152));
#20974=CARTESIAN_POINT('Ctrl Pts',(90.9145852724228,1.73465992769765,-0.389526819189099));
#20975=CARTESIAN_POINT('Ctrl Pts',(90.9028862768841,1.68503073000851,-0.573555756497857));
#20976=CARTESIAN_POINT('Ctrl Pts',(90.8958291998014,1.64436791040717,-0.681428770470135));
#20977=CARTESIAN_POINT('Ctrl Pts',(90.8868376996582,1.58270848745254,-0.806661080887335));
#20978=CARTESIAN_POINT('Ctrl Pts',(90.8852404037542,1.57139468000783,-0.828484713853723));
#20979=CARTESIAN_POINT('Ctrl Pts',(90.8825958288061,1.55210832501898,-0.863869763436651));
#20980=CARTESIAN_POINT('Ctrl Pts',(90.8815579058604,1.54440182282406,-0.877572905187356));
#20981=CARTESIAN_POINT('Ctrl Pts',(90.8796680124858,1.53013030331544,-0.902179163976264));
#20982=CARTESIAN_POINT('Ctrl Pts',(90.8788183517933,1.52362800428167,-0.913117560401485));
#20983=CARTESIAN_POINT('Ctrl Pts',(90.8769740530915,1.50933286759471,-0.936587477618503));
#20984=CARTESIAN_POINT('Ctrl Pts',(90.8759780003516,1.50150031625262,-0.949093560091067));
#20985=CARTESIAN_POINT('Ctrl Pts',(90.8731702394157,1.4791150708671,-0.983864903332042));
#20986=CARTESIAN_POINT('Ctrl Pts',(90.8713458334132,1.46421727113885,-1.00590217735028));
#20987=CARTESIAN_POINT('Ctrl Pts',(90.8632888076155,1.39693299671862,-1.10076783838728));
#20988=CARTESIAN_POINT('Ctrl Pts',(90.8568711993163,1.33957393479257,-1.16989277485529));
#20989=CARTESIAN_POINT('Ctrl Pts',(90.8432711798739,1.2096014097248,-1.3043788266945));
#20990=CARTESIAN_POINT('Ctrl Pts',(90.836092083392,1.13631510233555,-1.36869572950234));
#20991=CARTESIAN_POINT('Ctrl Pts',(90.8261172152295,1.02488054766708,-1.4513432959085));
#20992=CARTESIAN_POINT('Ctrl Pts',(90.8231783695936,0.990778324178097,-1.47483436488725));
#20993=CARTESIAN_POINT('Ctrl Pts',(90.819443397059,0.945419562447986,-1.50379521432319));
#20994=CARTESIAN_POINT('Ctrl Pts',(90.8185877636448,0.934885400320164,-1.51036667927128));
#20995=CARTESIAN_POINT('Ctrl Pts',(90.8172114317362,0.917693747247497,-1.52084245919051));
#20996=CARTESIAN_POINT('Ctrl Pts',(90.8166865660631,0.9110784080089,-1.5248146574681));
#20997=CARTESIAN_POINT('Ctrl Pts',(90.8156532864398,0.897933082823401,-1.53259171090727));
#20998=CARTESIAN_POINT('Ctrl Pts',(90.8151447789665,0.891404313136447,-1.53639823241275));
#20999=CARTESIAN_POINT('Ctrl Pts',(90.8138604974275,0.874769983140016,-1.54595495362762));
#21000=CARTESIAN_POINT('Ctrl Pts',(90.8130882675209,0.864631687947918,-1.55164793176589));
#21001=CARTESIAN_POINT('Ctrl Pts',(90.8098865072588,0.822065033990778,-1.57500369930661));
#21002=CARTESIAN_POINT('Ctrl Pts',(90.8075075202307,0.789143504051327,-1.59175391999361));
#21003=CARTESIAN_POINT('Ctrl Pts',(90.8006704748321,0.691624943064671,-1.63760048905792));
#21004=CARTESIAN_POINT('Ctrl Pts',(90.7963129016204,0.62577931754347,-1.6638756026224));
#21005=CARTESIAN_POINT('Ctrl Pts',(90.7845341755375,0.443767916978714,-1.72416683095149));
#21006=CARTESIAN_POINT('Ctrl Pts',(90.7771354360945,0.32543061719361,-1.75036346409506));
#21007=CARTESIAN_POINT('Ctrl Pts',(90.7677757053837,0.181156153830908,-1.76715592626368));
#21008=CARTESIAN_POINT('Ctrl Pts',(90.7661920588337,0.156902094767095,-1.7694742893946));
#21009=CARTESIAN_POINT('Ctrl Pts',(90.7635647029708,0.116984098866945,-1.77246277443643));
#21010=CARTESIAN_POINT('Ctrl Pts',(90.7625300976698,0.101344908574899,-1.77342571015882));
#21011=CARTESIAN_POINT('Ctrl Pts',(90.7606425602253,0.0729715253140104,
-1.7747961839436));
#21012=CARTESIAN_POINT('Ctrl Pts',(90.7597918812898,0.0602416677140853,
-1.77527385633855));
#21013=CARTESIAN_POINT('Ctrl Pts',(90.7579410476485,0.0326767663451601,
-1.77601137833165));
#21014=CARTESIAN_POINT('Ctrl Pts',(90.7569394271945,0.0178414967196386,
-1.77622235228174));
#21015=CARTESIAN_POINT('Ctrl Pts',(90.7541031093799,-0.023925986262745,
-1.7762930298592));
#21016=CARTESIAN_POINT('Ctrl Pts',(90.7522553276262,-0.050853866988934,
-1.77572608435241));
#21017=CARTESIAN_POINT('Ctrl Pts',(90.7440044955107,-0.169795627824018,
-1.77051428714231));
#21018=CARTESIAN_POINT('Ctrl Pts',(90.7374058369908,-0.261367302710889,
-1.75932771822355));
#21019=CARTESIAN_POINT('Ctrl Pts',(90.7232913756903,-0.45145846185995,-1.72093523936765));
#21020=CARTESIAN_POINT('Ctrl Pts',(90.7157767048709,-0.549352705534145,
-1.6922308459127));
#21021=CARTESIAN_POINT('Ctrl Pts',(90.7059473023638,-0.677331225236316,
-1.64242097110127));
#21022=CARTESIAN_POINT('Ctrl Pts',(90.7034374861994,-0.710022118810011,
-1.62855556314141));
#21023=CARTESIAN_POINT('Ctrl Pts',(90.7001591121276,-0.75299511728136,-1.60878885427543));
#21024=CARTESIAN_POINT('Ctrl Pts',(90.6993470035675,-0.763663369219857,
-1.60375231933771));
#21025=CARTESIAN_POINT('Ctrl Pts',(90.6980746875968,-0.780425713776407,
-1.59563353648172));
#21026=CARTESIAN_POINT('Ctrl Pts',(90.6976103696032,-0.786553340724527,
-1.59262190229232));
#21027=CARTESIAN_POINT('Ctrl Pts',(90.696645936336,-0.799305899429894,-1.58626266213039));
#21028=CARTESIAN_POINT('Ctrl Pts',(90.6961462786212,-0.805927425707033,
-1.58290875947911));
#21029=CARTESIAN_POINT('Ctrl Pts',(90.6948994178961,-0.822481932274537,
-1.57439284733317));
#21030=CARTESIAN_POINT('Ctrl Pts',(90.6941554400321,-0.832387727467028,
-1.56917814606081));
#21031=CARTESIAN_POINT('Ctrl Pts',(90.6911972819851,-0.871851764224807,
-1.54792424135628));
#21032=CARTESIAN_POINT('Ctrl Pts',(90.6890252509883,-0.901003137123161,
-1.5311396566469));
#21033=CARTESIAN_POINT('Ctrl Pts',(90.6830331206487,-0.981246263259831,
-1.48185175560645));
#21034=CARTESIAN_POINT('Ctrl Pts',(90.6792878284999,-1.0311802942413,-1.44754864361974));
#21035=CARTESIAN_POINT('Ctrl Pts',(90.6669623961319,-1.19040909168765,-1.32573450536113));
#21036=CARTESIAN_POINT('Ctrl Pts',(90.6584842110468,-1.29110182760245,-1.22788345258922));
#21037=CARTESIAN_POINT('Ctrl Pts',(90.6478323179766,-1.39509742716565,-1.09972651356004));
#21038=CARTESIAN_POINT('Ctrl Pts',(90.6461959404316,-1.41051145869358,-1.07988543743793));
#21039=CARTESIAN_POINT('Ctrl Pts',(90.6435865104896,-1.4341714663286,-1.04805895605372));
#21040=CARTESIAN_POINT('Ctrl Pts',(90.6426245948387,-1.44270025403382,-1.036287279633));
#21041=CARTESIAN_POINT('Ctrl Pts',(90.6408148979829,-1.45838001792699,-1.01407684773768));
#21042=CARTESIAN_POINT('Ctrl Pts',(90.6399685370063,-1.46556583929526,-1.00366373158723));
#21043=CARTESIAN_POINT('Ctrl Pts',(90.6380569717653,-1.48146192454421,-0.980093659727605));
#21044=CARTESIAN_POINT('Ctrl Pts',(90.636989467301,-1.49010924724986,-0.966895764150478));
#21045=CARTESIAN_POINT('Ctrl Pts',(90.6337259950201,-1.51584331029082,-0.926454120866957));
#21046=CARTESIAN_POINT('Ctrl Pts',(90.631509579253,-1.53236624868443,-0.898861293022755));
#21047=CARTESIAN_POINT('Ctrl Pts',(90.6234173790807,-1.58925703770875,-0.7977236724954));
#21048=CARTESIAN_POINT('Ctrl Pts',(90.6173947836576,-1.6251475718814,-0.721798491952967));
#21049=CARTESIAN_POINT('Ctrl Pts',(90.6038138162076,-1.69273239929099,-0.547957992802273));
#21050=CARTESIAN_POINT('Ctrl Pts',(90.5962347370852,-1.72156485035034,-0.449239680180405));
#21051=CARTESIAN_POINT('Ctrl Pts',(90.5864322471817,-1.74845905521874,-0.314861304597428));
#21052=CARTESIAN_POINT('Ctrl Pts',(90.5840022961059,-1.75422770488908,-0.280948810899604));
#21053=CARTESIAN_POINT('Ctrl Pts',(90.5808126636568,-1.76062515771961,-0.235368686768145));
#21054=CARTESIAN_POINT('Ctrl Pts',(90.5800119666206,-1.76212879212487,-0.223833650245843));
#21055=CARTESIAN_POINT('Ctrl Pts',(90.5787543717479,-1.76432901311362,-0.205555653267928));
#21056=CARTESIAN_POINT('Ctrl Pts',(90.5782934819438,-1.76510047699653,-0.198822290355401));
#21057=CARTESIAN_POINT('Ctrl Pts',(90.577326440946,-1.76664567259632,-0.184617304969676));
#21058=CARTESIAN_POINT('Ctrl Pts',(90.576820805837,-1.76741059025658,-0.177144834056858));
#21059=CARTESIAN_POINT('Ctrl Pts',(90.5755527948373,-1.76921903364286,-0.158298807376265));
#21060=CARTESIAN_POINT('Ctrl Pts',(90.5747937872704,-1.77020032877952,-0.146919414814571));
#21061=CARTESIAN_POINT('Ctrl Pts',(90.5717285552652,-1.77374464984017,-0.100603456763478));
#21062=CARTESIAN_POINT('Ctrl Pts',(90.5694676523215,-1.775383882622,-0.0656017469455326));
#21063=CARTESIAN_POINT('Ctrl Pts',(90.5631338560187,-1.7770984862331,0.0340034011332461));
#21064=CARTESIAN_POINT('Ctrl Pts',(90.559144938162,-1.77468737191219,0.0985958262223297));
#21065=CARTESIAN_POINT('Ctrl Pts',(90.54703751644,-1.75662537261308,0.294691684681125));
#21066=CARTESIAN_POINT('Ctrl Pts',(90.5389818428074,-1.72980243366558,0.42468262781185));
#21067=CARTESIAN_POINT('Ctrl Pts',(90.5287631777443,-1.68070754224882,0.575297587422005));
#21068=CARTESIAN_POINT('Ctrl Pts',(90.527063910504,-1.67207396965095,0.599928065069647));
#21069=CARTESIAN_POINT('Ctrl Pts',(90.5243698980803,-1.65768119532713,0.638261435568397));
#21070=CARTESIAN_POINT('Ctrl Pts',(90.5233872202813,-1.65228710791401,0.652098072452742));
#21071=CARTESIAN_POINT('Ctrl Pts',(90.5215474468001,-1.64192614026216,0.677721303937154));
#21072=CARTESIAN_POINT('Ctrl Pts',(90.5206919085464,-1.6370041927749,0.689525107620895));
#21073=CARTESIAN_POINT('Ctrl Pts',(90.51877100643,-1.62572530325261,0.715772524957874));
#21074=CARTESIAN_POINT('Ctrl Pts',(90.5177034627051,-1.61930254436453,0.730186490586994));
#21075=CARTESIAN_POINT('Ctrl Pts',(90.5144793100564,-1.59944980931749,0.773189502109483));
#21076=CARTESIAN_POINT('Ctrl Pts',(90.5123034561485,-1.58544908565549,0.801506503654535));
#21077=CARTESIAN_POINT('Ctrl Pts',(90.504084304135,-1.53036654106553,0.905816518903952));
#21078=CARTESIAN_POINT('Ctrl Pts',(90.4978844002723,-1.48451873790832,0.97914549612045));
#21079=CARTESIAN_POINT('Ctrl Pts',(90.4839080985347,-1.37111392453091,1.13414396369614));
#21080=CARTESIAN_POINT('Ctrl Pts',(90.4761128415445,-1.30121136469294,1.21370765009496));
#21081=CARTESIAN_POINT('Ctrl Pts',(90.46643890602,-1.20277415857796,1.30740595006728));
#21082=CARTESIAN_POINT('Ctrl Pts',(90.4643140275816,-1.18037180431038,1.32766661985536));
#21083=CARTESIAN_POINT('Ctrl Pts',(90.4614517724146,-1.14898265714858,1.35463201005526));
#21084=CARTESIAN_POINT('Ctrl Pts',(90.4606835312438,-1.14043425739005,1.36183653565372));
#21085=CARTESIAN_POINT('Ctrl Pts',(90.4594130047932,-1.12608091232583,1.37370348211296));
#21086=CARTESIAN_POINT('Ctrl Pts',(90.4589076455416,-1.1203137655118,1.37841087964511));
#21087=CARTESIAN_POINT('Ctrl Pts',(90.4578622236763,-1.10825967514635,1.38812432150205));
#21088=CARTESIAN_POINT('Ctrl Pts',(90.4573225672702,-1.10196813748527,1.39312414010998));
#21089=CARTESIAN_POINT('Ctrl Pts',(90.4558914620666,-1.08510617249149,1.40633845789726));
#21090=CARTESIAN_POINT('Ctrl Pts',(90.4550050455433,-1.07447622010225,1.41447663192102));
#21091=CARTESIAN_POINT('Ctrl Pts',(90.4503376224201,-1.01758251620421,1.45702229459449));
#21092=CARTESIAN_POINT('Ctrl Pts',(90.4466795344339,-0.969751438643358,
1.48928562257418));
#21093=CARTESIAN_POINT('Ctrl Pts',(90.4385254596719,-0.858162831344932,
1.55689474843891));
#21094=CARTESIAN_POINT('Ctrl Pts',(90.4340679726641,-0.793632347699398,
1.59075863465574));
#21095=CARTESIAN_POINT('Ctrl Pts',(90.4235431140112,-0.638078331995184,
1.66056104955992));
#21096=CARTESIAN_POINT('Ctrl Pts',(90.4174577494542,-0.545815868431496,
1.69312986752891));
#21097=CARTESIAN_POINT('Ctrl Pts',(90.4096559488324,-0.429481479981975,
1.72369399568845));
#21098=CARTESIAN_POINT('Ctrl Pts',(90.4081773400052,-0.407505491656879,
1.72902126432773));
#21099=CARTESIAN_POINT('Ctrl Pts',(90.4057593236647,-0.371730440535109,
1.73697369732101));
#21100=CARTESIAN_POINT('Ctrl Pts',(90.4048280957307,-0.357991015325491,
1.73985733889243));
#21101=CARTESIAN_POINT('Ctrl Pts',(90.4030199872131,-0.33139827621741,1.74511032154339));
#21102=CARTESIAN_POINT('Ctrl Pts',(90.4021438514935,-0.318550121125323,
1.74750126081862));
#21103=CARTESIAN_POINT('Ctrl Pts',(90.4000798891294,-0.288379170163522,
1.75277205160587));
#21104=CARTESIAN_POINT('Ctrl Pts',(90.3988885488663,-0.27103799993061,1.75553717561614));
#21105=CARTESIAN_POINT('Ctrl Pts',(90.3948476544138,-0.212487310191983,
1.76398515304366));
#21106=CARTESIAN_POINT('Ctrl Pts',(90.3919617861875,-0.171122654339681,
1.76847703413931));
#21107=CARTESIAN_POINT('Ctrl Pts',(90.3846678953406,-0.0677439472668281,
1.77604240285535));
#21108=CARTESIAN_POINT('Ctrl Pts',(90.3802134746023,-0.0056573794241821,
1.77732455496254));
#21109=CARTESIAN_POINT('Ctrl Pts',(90.3670967695023,0.174895057219392,1.77159238430677));
#21110=CARTESIAN_POINT('Ctrl Pts',(90.3583119772578,0.292750020355315,1.75596859022942));
#21111=CARTESIAN_POINT('Ctrl Pts',(90.3498698986825,0.408169026503127,1.72871689651704));
#21112=CARTESIAN_POINT('',(90.3498698986825,-1.48890580190326,0.968619417293912));
#21113=CARTESIAN_POINT('Origin',(90.3498698986825,0.,0.));
#21114=CARTESIAN_POINT('Ctrl Pts',(90.3498698986825,-1.48890580190324,0.968619417293899));
#21115=CARTESIAN_POINT('Ctrl Pts',(90.3538563142452,-1.52125431666485,0.918895149483884));
#21116=CARTESIAN_POINT('Ctrl Pts',(90.3577455404558,-1.55108810095714,0.867478027813688));
#21117=CARTESIAN_POINT('Ctrl Pts',(90.3615871323241,-1.57825856532581,0.814657819541863));
#21118=CARTESIAN_POINT('Ctrl Pts',(90.3619810187035,-1.58104440937268,0.80924205407051));
#21119=CARTESIAN_POINT('Ctrl Pts',(90.3623744043114,-1.58380226099585,0.803811582878728));
#21120=CARTESIAN_POINT('Ctrl Pts',(90.3627673425631,-1.58653196531297,0.79836674871169));
#21121=CARTESIAN_POINT('Ctrl Pts',(90.3670119182073,-1.61601862488144,0.739550865070549));
#21122=CARTESIAN_POINT('Ctrl Pts',(90.3712050420279,-1.64222035080938,0.679053296202822));
#21123=CARTESIAN_POINT('Ctrl Pts',(90.3754073490847,-1.6649903892128,0.617281304883328));
#21124=CARTESIAN_POINT('Ctrl Pts',(90.379587284972,-1.68763921029854,0.555838159521998));
#21125=CARTESIAN_POINT('Ctrl Pts',(90.3837767749571,-1.70689329459749,0.493134426296299));
#21126=CARTESIAN_POINT('Ctrl Pts',(90.3880198339045,-1.72265438865196,0.429574094169994));
#21127=CARTESIAN_POINT('Ctrl Pts',(90.3922629594753,-1.73841573018284,0.366012764036609));
#21128=CARTESIAN_POINT('Ctrl Pts',(90.3965599313326,-1.75068430678455,0.301594930371655));
#21129=CARTESIAN_POINT('Ctrl Pts',(90.4009335405249,-1.75940186175885,0.236724745270866));
#21130=CARTESIAN_POINT('Ctrl Pts',(90.405308475957,-1.7681220602179,0.171834889133232));
#21131=CARTESIAN_POINT('Ctrl Pts',(90.4097602207429,-1.77328927467888,0.10649243312025));
#21132=CARTESIAN_POINT('Ctrl Pts',(90.4142873758366,-1.77488127340981,0.0411009767190024));
#21133=CARTESIAN_POINT('Ctrl Pts',(90.4188550969619,-1.77648753740658,-0.024876426449256));
#21134=CARTESIAN_POINT('Ctrl Pts',(90.4234996199107,-1.77445421991782,-0.0909037515290607));
#21135=CARTESIAN_POINT('Ctrl Pts',(90.4281935981655,-1.76879385216752,-0.156567278160123));
#21136=CARTESIAN_POINT('Ctrl Pts',(90.4328560318523,-1.76317152333553,-0.221789531425848));
#21137=CARTESIAN_POINT('Ctrl Pts',(90.4375670778683,-1.75397062604308,-0.286652943004453));
#21138=CARTESIAN_POINT('Ctrl Pts',(90.4422756562143,-1.7412388162352,-0.350751928860527));
#21139=CARTESIAN_POINT('Ctrl Pts',(90.4470320197127,-1.72837779726297,-0.415501425250696));
#21140=CARTESIAN_POINT('Ctrl Pts',(90.4517855276462,-1.71191336093139,-0.479470963433884));
#21141=CARTESIAN_POINT('Ctrl Pts',(90.4564623747301,-1.69193526026765,-0.542241124442562));
#21142=CARTESIAN_POINT('Ctrl Pts',(90.4606543295379,-1.67402847528455,-0.598503318504739));
#21143=CARTESIAN_POINT('Ctrl Pts',(90.4647841420072,-1.65329854864641,-0.653802855979749));
#21144=CARTESIAN_POINT('Ctrl Pts',(90.4687890441026,-1.6298447879185,-0.707834103636427));
#21145=CARTESIAN_POINT('Ctrl Pts',(90.4692522995958,-1.6271318418251,-0.714084012295091));
#21146=CARTESIAN_POINT('Ctrl Pts',(90.4697138837835,-1.62438246579518,-0.720317006591094));
#21147=CARTESIAN_POINT('Ctrl Pts',(90.4701736995197,-1.62159682426134,-0.726532657354804));
#21148=CARTESIAN_POINT('Ctrl Pts',(90.4701754501884,-1.62158621841431,-0.726556322367136));
#21149=CARTESIAN_POINT('Ctrl Pts',(90.4701772008335,-1.62157561202607,-0.726579987165501));
#21150=CARTESIAN_POINT('Ctrl Pts',(90.470178951455,-1.62156500509664,-0.726603651749862));
#21151=CARTESIAN_POINT('Ctrl Pts',(90.47399760591,-1.59842796628609,-0.778223530068028));
#21152=CARTESIAN_POINT('Ctrl Pts',(90.4777041248918,-1.57271198408437,-0.828827245037696));
#21153=CARTESIAN_POINT('Ctrl Pts',(90.4813509415062,-1.54454993674521,-0.878148106426725));
#21154=CARTESIAN_POINT('Ctrl Pts',(90.4817603601505,-1.54138825672098,-0.883685231634755));
#21155=CARTESIAN_POINT('Ctrl Pts',(90.4821690263079,-1.5381957948568,-0.889206163508004));
#21156=CARTESIAN_POINT('Ctrl Pts',(90.4825770141721,-1.53497277616297,-0.894710507219073));
#21157=CARTESIAN_POINT('Ctrl Pts',(90.486565021165,-1.50346835601027,-0.94851446351322));
#21158=CARTESIAN_POINT('Ctrl Pts',(90.4904889952222,-1.46903946690765,-1.00073583159466));
#21159=CARTESIAN_POINT('Ctrl Pts',(90.4944116230711,-1.43190267812393,-1.05105650382837));
#21160=CARTESIAN_POINT('Ctrl Pts',(90.4946259244998,-1.4298738170642,-1.05380562823408));
#21161=CARTESIAN_POINT('Ctrl Pts',(90.4948402219106,-1.42783688463797,-1.05654907261513));
#21162=CARTESIAN_POINT('Ctrl Pts',(90.495054525525,-1.42579191997013,-1.05928678275577));
#21163=CARTESIAN_POINT('Ctrl Pts',(90.4990196573749,-1.38795515944602,-1.10994099923413));
#21164=CARTESIAN_POINT('Ctrl Pts',(90.5029872835318,-1.34736523212034,-1.15863524651694));
#21165=CARTESIAN_POINT('Ctrl Pts',(90.5070063827528,-1.30427777250265,-1.20507464471594));
#21166=CARTESIAN_POINT('Ctrl Pts',(90.5110226047008,-1.26122115919562,-1.25148079695157));
#21167=CARTESIAN_POINT('Ctrl Pts',(90.5150904846149,-1.21567087598052,-1.29563546976753));
#21168=CARTESIAN_POINT('Ctrl Pts',(90.519238130043,-1.16790637143662,-1.33727572254209));
#21169=CARTESIAN_POINT('Ctrl Pts',(90.5233843674953,-1.12015808121726,-1.37890183995444));
#21170=CARTESIAN_POINT('Ctrl Pts',(90.5276104382176,-1.07019723849451,-1.41801532460637));
#21171=CARTESIAN_POINT('Ctrl Pts',(90.5319208490151,-1.01832400466784,-1.45438312205025));
#21172=CARTESIAN_POINT('Ctrl Pts',(90.5362314191256,-0.966448853603774,
-1.4907522636498));
#21173=CARTESIAN_POINT('Ctrl Pts',(90.5406263480194,-0.912661235175542,
-1.52437552719678));
#21174=CARTESIAN_POINT('Ctrl Pts',(90.5450855649199,-0.857280619042244,
-1.55504875905309));
#21175=CARTESIAN_POINT('Ctrl Pts',(90.5495495604224,-0.80184065573558,-1.58575486106751));
#21176=CARTESIAN_POINT('Ctrl Pts',(90.554077878698,-0.74480423322187,-1.61350452338537));
#21177=CARTESIAN_POINT('Ctrl Pts',(90.5586264001637,-0.686511008695593,
-1.63812241542801));
#21178=CARTESIAN_POINT('Ctrl Pts',(90.5631778158279,-0.628180692520079,
-1.66275597169618));
#21179=CARTESIAN_POINT('Ctrl Pts',(90.5677491887434,-0.56859182097684,-1.68425353719366));
#21180=CARTESIAN_POINT('Ctrl Pts',(90.5722750656712,-0.508105382050814,
-1.70247122901301));
#21181=CARTESIAN_POINT('Ctrl Pts',(90.5765173364677,-0.451409219619926,
-1.71954734116053));
#21182=CARTESIAN_POINT('Ctrl Pts',(90.5807191840371,-0.393923833804837,
-1.73374174739534));
#21183=CARTESIAN_POINT('Ctrl Pts',(90.5848140042572,-0.335967087298439,
-1.74496526177759));
#21184=CARTESIAN_POINT('Ctrl Pts',(90.5850952976667,-0.331985752356128,
-1.74573626037015));
#21185=CARTESIAN_POINT('Ctrl Pts',(90.5853760860147,-0.328002178447056,
-1.74649325361629));
#21186=CARTESIAN_POINT('Ctrl Pts',(90.5856563477101,-0.324016461984582,
-1.74723621877522));
#21187=CARTESIAN_POINT('Ctrl Pts',(90.586974240284,-0.305274171430572,-1.7507299115683));
#21188=CARTESIAN_POINT('Ctrl Pts',(90.5882804122919,-0.286485050445651,
-1.75391334329275));
#21189=CARTESIAN_POINT('Ctrl Pts',(90.5895724730613,-0.26766022811415,-1.75678435040296));
#21190=CARTESIAN_POINT('Ctrl Pts',(90.5895746269833,-0.267628846309676,
-1.75678913649773));
#21191=CARTESIAN_POINT('Ctrl Pts',(90.5895767808694,-0.267597464341494,
-1.75679392173609));
#21192=CARTESIAN_POINT('Ctrl Pts',(90.5895789347197,-0.267566082209624,
-1.75679870611799));
#21193=CARTESIAN_POINT('Ctrl Pts',(90.5934312878049,-0.211436344065201,
-1.76535599930008));
#21194=CARTESIAN_POINT('Ctrl Pts',(90.5971689910853,-0.154779224758392,
-1.7711712273231));
#21195=CARTESIAN_POINT('Ctrl Pts',(90.6008427914221,-0.0978911430855949,
-1.77421564503471));
#21196=CARTESIAN_POINT('Ctrl Pts',(90.6012855002881,-0.0910358826428607,
-1.77458251056605));
#21197=CARTESIAN_POINT('Ctrl Pts',(90.6017272812006,-0.084177321001716,
-1.77490917335082));
#21198=CARTESIAN_POINT('Ctrl Pts',(90.6021682229604,-0.0773160193275386,
-1.77519561121616));
#21199=CARTESIAN_POINT('Ctrl Pts',(90.6063891314751,-0.0116363099084832,
-1.77793753347171));
#21200=CARTESIAN_POINT('Ctrl Pts',(90.6105340022366,0.0543000403042987,
-1.77699014460809));
#21201=CARTESIAN_POINT('Ctrl Pts',(90.6146743800401,0.120045333876444,-1.77237148682125));
#21202=CARTESIAN_POINT('Ctrl Pts',(90.6186870951359,0.183763464084872,-1.76789523883056));
#21203=CARTESIAN_POINT('Ctrl Pts',(90.6226960186818,0.247302095079509,-1.75997141185029));
#21204=CARTESIAN_POINT('Ctrl Pts',(90.6267510949758,0.310267424014638,-1.7486612585104));
#21205=CARTESIAN_POINT('Ctrl Pts',(90.6308036507985,0.37319361624946,-1.73735813510412));
#21206=CARTESIAN_POINT('Ctrl Pts',(90.6349025817534,0.435547204357498,-1.7226732392878));
#21207=CARTESIAN_POINT('Ctrl Pts',(90.6390770766321,0.496949467663568,-1.70470523642112));
#21208=CARTESIAN_POINT('Ctrl Pts',(90.6432504727539,0.558335569455983,-1.68674196286094));
#21209=CARTESIAN_POINT('Ctrl Pts',(90.6474995272466,0.6187708514289,-1.66549750550593));
#21210=CARTESIAN_POINT('Ctrl Pts',(90.6518296869147,0.677891277099393,-1.64110394788305));
#21211=CARTESIAN_POINT('Ctrl Pts',(90.6561602585123,0.737017326914143,-1.61670806969355));
#21212=CARTESIAN_POINT('Ctrl Pts',(90.6605719693885,0.794828270312418,-1.5891625530848));
#21213=CARTESIAN_POINT('Ctrl Pts',(90.66504540428,0.850974313885249,-1.55863110702535));
#21214=CARTESIAN_POINT('Ctrl Pts',(90.6695236925955,0.907181272741975,-1.52806653607256));
#21215=CARTESIAN_POINT('Ctrl Pts',(90.674063737033,0.961719693086612,-1.49450945947954));
#21216=CARTESIAN_POINT('Ctrl Pts',(90.6786217336073,1.01425317371748,-1.4581559940994));
#21217=CARTESIAN_POINT('Ctrl Pts',(90.6831827264511,1.06682118804405,-1.42177863120674));
#21218=CARTESIAN_POINT('Ctrl Pts',(90.6877614187742,1.11738152335539,-1.38260092592077));
#21219=CARTESIAN_POINT('Ctrl Pts',(90.6922923521835,1.16561251953689,-1.34085402094085));
#21220=CARTESIAN_POINT('Ctrl Pts',(90.6965307994336,1.21073005154868,-1.30180201142529));
#21221=CARTESIAN_POINT('Ctrl Pts',(90.7007269946079,1.25380961442412,-1.26050123889405));
#21222=CARTESIAN_POINT('Ctrl Pts',(90.7048145774088,1.29460112222741,-1.21717422755039));
#21223=CARTESIAN_POINT('Ctrl Pts',(90.7051038995783,1.29748837567578,-1.214107509264));
#21224=CARTESIAN_POINT('Ctrl Pts',(90.7053926776092,1.30036418725321,-1.21103063464629));
#21225=CARTESIAN_POINT('Ctrl Pts',(90.7056808879696,1.30322847787149,-1.20794368006088));
#21226=CARTESIAN_POINT('Ctrl Pts',(90.706642560046,1.31278576200889,-1.19764343262661));
#21227=CARTESIAN_POINT('Ctrl Pts',(90.7075978710689,1.32221459126303,-1.18723119764786));
#21228=CARTESIAN_POINT('Ctrl Pts',(90.7085458919079,1.33151184766431,-1.1767102021235));
#21229=CARTESIAN_POINT('Ctrl Pts',(90.7085477520551,1.33153009015947,-1.17668955848396));
#21230=CARTESIAN_POINT('Ctrl Pts',(90.7085496121766,1.33154833217906,-1.17666891439259));
#21231=CARTESIAN_POINT('Ctrl Pts',(90.7085514722723,1.33156657372303,-1.17664826984943));
#21232=CARTESIAN_POINT('Ctrl Pts',(90.7124095359009,1.36940174310797,-1.13382898936784));
#21233=CARTESIAN_POINT('Ctrl Pts',(90.7161568944749,1.40519106883275,-1.08906167835935));
#21234=CARTESIAN_POINT('Ctrl Pts',(90.7198447048519,1.43874779482561,-1.04258403106708));
#21235=CARTESIAN_POINT('Ctrl Pts',(90.7202667374043,1.44258802229817,-1.03726513499749));
#21236=CARTESIAN_POINT('Ctrl Pts',(90.7206879900847,1.44639900936124,-1.03192389566102));
#21237=CARTESIAN_POINT('Ctrl Pts',(90.721108539565,1.45018047627668,-1.02656071269748));
#21238=CARTESIAN_POINT('Ctrl Pts',(90.7251999964893,1.48696974774802,-0.974383185190741));
#21239=CARTESIAN_POINT('Ctrl Pts',(90.729225622378,1.52096537489848,-0.920122745683341));
#21240=CARTESIAN_POINT('Ctrl Pts',(90.7332498753217,1.55195968493651,-0.864131848584758));
#21241=CARTESIAN_POINT('Ctrl Pts',(90.7372699500544,1.58292181489895,-0.808199084456343));
#21242=CARTESIAN_POINT('Ctrl Pts',(90.7412891299274,1.61088923626005,-0.750539827506467));
#21243=CARTESIAN_POINT('Ctrl Pts',(90.7453565652005,1.63569909853021,-0.69151804308843));
#21244=CARTESIAN_POINT('Ctrl Pts',(90.7494217935304,1.66049549925754,-0.632528283204455));
#21245=CARTESIAN_POINT('Ctrl Pts',(90.7535355012154,1.68213804425792,-0.572177673540597));
#21246=CARTESIAN_POINT('Ctrl Pts',(90.7577260849918,1.70050334020167,-0.510837996941952));
#21247=CARTESIAN_POINT('Ctrl Pts',(90.7619153268021,1.71886275495941,-0.449517963372648));
#21248=CARTESIAN_POINT('Ctrl Pts',(90.7661815269526,1.73394718308619,-0.387209598446523));
#21249=CARTESIAN_POINT('Ctrl Pts',(90.7705293740152,1.74566922202807,-0.324290519440164));
#21250=CARTESIAN_POINT('Ctrl Pts',(90.7748788694906,1.7573957051829,-0.261347585728403));
#21251=CARTESIAN_POINT('Ctrl Pts',(90.7793100912484,1.76575729635694,-0.19779350654627));
#21252=CARTESIAN_POINT('Ctrl Pts',(90.7838029196334,1.77070081358476,-0.134011531087324));
#21253=CARTESIAN_POINT('Ctrl Pts',(90.7858318981217,1.77293332487895,-0.105207346937488));
#21254=CARTESIAN_POINT('Ctrl Pts',(90.7878731037697,1.77446919335584,-0.0763567518078401));
#21255=CARTESIAN_POINT('Ctrl Pts',(90.7899230490922,1.77530581490221,-0.0474953858958098));
#21256=CARTESIAN_POINT('Origin',(88.3562164250559,0.,0.));
#21257=CARTESIAN_POINT('',(91.6892085959652,1.77561363837197,-0.0475422940912394));
#21258=CARTESIAN_POINT('',(91.5422141974348,1.77561363837144,-0.0475422941110715));
#21259=CARTESIAN_POINT('',(88.3562164250559,1.77561363837197,-0.0475422940912398));
#21260=CARTESIAN_POINT('Ctrl Pts',(91.6892085959652,1.77561363837197,-0.0475422940912359));
#21261=CARTESIAN_POINT('Ctrl Pts',(91.6826296493429,1.77317281232423,-0.138702472666949));
#21262=CARTESIAN_POINT('Ctrl Pts',(91.6759149193743,1.76371331345252,-0.229614208752581));
#21263=CARTESIAN_POINT('Ctrl Pts',(91.6643821335648,1.73522339018167,-0.385436676345231));
#21264=CARTESIAN_POINT('Ctrl Pts',(91.6595491631098,1.71943375700664,-0.450678526944558));
#21265=CARTESIAN_POINT('Ctrl Pts',(91.6539287316192,1.69602371461896,-0.527972385438873));
#21266=CARTESIAN_POINT('Ctrl Pts',(91.6529836089651,1.69190619307101,-0.541021943213308));
#21267=CARTESIAN_POINT('Ctrl Pts',(91.6514999167809,1.68514750048711,-0.561609942369776));
#21268=CARTESIAN_POINT('Ctrl Pts',(91.6509559672094,1.68260567713873,-0.569180083416648));
#21269=CARTESIAN_POINT('Ctrl Pts',(91.6499223610523,1.67765126990361,-0.583612182041431));
#21270=CARTESIAN_POINT('Ctrl Pts',(91.6494322470786,1.67524747915378,-0.590476797094879));
#21271=CARTESIAN_POINT('Ctrl Pts',(91.6483456422136,1.66979780691413,-0.605738499458421));
#21272=CARTESIAN_POINT('Ctrl Pts',(91.6477503827448,1.66673057207595,-0.614127880956124));
#21273=CARTESIAN_POINT('Ctrl Pts',(91.6456999947142,1.65588627874564,-0.643108992245147));
#21274=CARTESIAN_POINT('Ctrl Pts',(91.6442621190886,1.64778950971065,-0.663579974064104));
#21275=CARTESIAN_POINT('Ctrl Pts',(91.6345175979573,1.58969180114976,-0.802841416987966));
#21276=CARTESIAN_POINT('Ctrl Pts',(91.6267615875747,1.52726583677266,-0.916046674103866));
#21277=CARTESIAN_POINT('Ctrl Pts',(91.6150501003413,1.4180051541739,-1.07147360270502));
#21278=CARTESIAN_POINT('Ctrl Pts',(91.611254650614,1.38032936482806,-1.11959114832423));
#21279=CARTESIAN_POINT('Ctrl Pts',(91.6047754119644,1.31335358689614,-1.19659788256551));
#21280=CARTESIAN_POINT('Ctrl Pts',(91.6021389272148,1.28539395364529,-1.22658310545357));
#21281=CARTESIAN_POINT('Ctrl Pts',(91.5983254879301,1.24417155307738,-1.26783344795948));
#21282=CARTESIAN_POINT('Ctrl Pts',(91.5971845319235,1.23174078880252,-1.27991370775004));
#21283=CARTESIAN_POINT('Ctrl Pts',(91.5951804954699,1.20975292009111,-1.30066459050129));
#21284=CARTESIAN_POINT('Ctrl Pts',(91.5943210110471,1.20027428264879,-1.30941671595651));
#21285=CARTESIAN_POINT('Ctrl Pts',(91.5925294649403,1.18042236884044,-1.32735035926103));
#21286=CARTESIAN_POINT('Ctrl Pts',(91.5915967881965,1.17003537112961,-1.33651530348929));
#21287=CARTESIAN_POINT('Ctrl Pts',(91.5891512859068,1.14267262055608,-1.36009532114593));
#21288=CARTESIAN_POINT('Ctrl Pts',(91.5876305633874,1.12553154597135,-1.37431388723694));
#21289=CARTESIAN_POINT('Ctrl Pts',(91.5800310116375,1.0392922044019,-1.44315400639718));
#21290=CARTESIAN_POINT('Ctrl Pts',(91.5737652270432,0.96647492198799,-1.49289778941215));
#21291=CARTESIAN_POINT('Ctrl Pts',(91.5598710806628,0.800631599885092,-1.58895757418608));
#21292=CARTESIAN_POINT('Ctrl Pts',(91.5522203315567,0.70661504025961,-1.63293965944108));
#21293=CARTESIAN_POINT('Ctrl Pts',(91.5425675423318,0.580764312996491,-1.67889841692755));
#21294=CARTESIAN_POINT('Ctrl Pts',(91.5403974382705,0.5519621084944,-1.68858672269114));
#21295=CARTESIAN_POINT('Ctrl Pts',(91.5367689921219,0.502736464015158,-1.70375066271102));
#21296=CARTESIAN_POINT('Ctrl Pts',(91.5352955943416,0.482438457589693,-1.70960916731568));
#21297=CARTESIAN_POINT('Ctrl Pts',(91.5331901230705,0.45291727772037,-1.71756201054307));
#21298=CARTESIAN_POINT('Ctrl Pts',(91.5325432470355,0.443775133870238,-1.719946790228));
#21299=CARTESIAN_POINT('Ctrl Pts',(91.5314112844725,0.427642142689588,-1.72401797105399));
#21300=CARTESIAN_POINT('Ctrl Pts',(91.5309245214273,0.420659502634534,-1.72573501902722));
#21301=CARTESIAN_POINT('Ctrl Pts',(91.5298580839211,0.405260617343389,-1.72942262057064));
#21302=CARTESIAN_POINT('Ctrl Pts',(91.5292794734823,0.396840210694156,-1.73137420089205));
#21303=CARTESIAN_POINT('Ctrl Pts',(91.5276171672606,0.372471492100008,-1.73683496566747));
#21304=CARTESIAN_POINT('Ctrl Pts',(91.52654190647,0.356488131968085,-1.74018590059446));
#21305=CARTESIAN_POINT('Ctrl Pts',(91.5177637555482,0.224422147541329,-1.76597766884389));
#21306=CARTESIAN_POINT('Ctrl Pts',(91.5105803185552,0.106394729830693,-1.7770004006878));
#21307=CARTESIAN_POINT('Ctrl Pts',(91.4967372440651,-0.119007806605712,
-1.775494608696));
#21308=CARTESIAN_POINT('Ctrl Pts',(91.4901175842461,-0.225852135552002,
-1.76508666694622));
#21309=CARTESIAN_POINT('Ctrl Pts',(91.4816202469844,-0.354956980557504,
-1.74059162395977));
#21310=CARTESIAN_POINT('Ctrl Pts',(91.4800361437933,-0.378716699610612,
-1.73557691505368));
#21311=CARTESIAN_POINT('Ctrl Pts',(91.4774963104821,-0.416267935295048,
-1.72684359669201));
#21312=CARTESIAN_POINT('Ctrl Pts',(91.4765507673244,-0.430130774113298,
-1.72344286197296));
#21313=CARTESIAN_POINT('Ctrl Pts',(91.4747482112428,-0.456327225807575,
-1.71668078219239));
#21314=CARTESIAN_POINT('Ctrl Pts',(91.4738923228931,-0.468668529293851,
-1.71335263149227));
#21315=CARTESIAN_POINT('Ctrl Pts',(91.4719257717743,-0.49679607990436,-1.70544067977924));
#21316=CARTESIAN_POINT('Ctrl Pts',(91.4708123545692,-0.512556564177838,
-1.70077041190923));
#21317=CARTESIAN_POINT('Ctrl Pts',(91.4672703569929,-0.562160449487276,
-1.68531932228674));
#21318=CARTESIAN_POINT('Ctrl Pts',(91.4648161591335,-0.595744656745387,
-1.67374238753223));
#21319=CARTESIAN_POINT('Ctrl Pts',(91.4521477258142,-0.765056985236665,
-1.60963672689961));
#21320=CARTESIAN_POINT('Ctrl Pts',(91.4414289212185,-0.89429196544866,-1.54158075779734));
#21321=CARTESIAN_POINT('Ctrl Pts',(91.4275552356117,-1.05079419334238,-1.43280508124705));
#21322=CARTESIAN_POINT('Ctrl Pts',(91.4242945118892,-1.08684280589143,-1.40565716048554));
#21323=CARTESIAN_POINT('Ctrl Pts',(91.4191120590128,-1.14342039327851,-1.35956978253387));
#21324=CARTESIAN_POINT('Ctrl Pts',(91.4171559705445,-1.16460467316928,-1.34146798437002));
#21325=CARTESIAN_POINT('Ctrl Pts',(91.4145056371625,-1.19317740923358,-1.31586550717301));
#21326=CARTESIAN_POINT('Ctrl Pts',(91.4137846105695,-1.20093707209892,-1.30878742559641));
#21327=CARTESIAN_POINT('Ctrl Pts',(91.4125691318587,-1.21400219346931,-1.29665585486836));
#21328=CARTESIAN_POINT('Ctrl Pts',(91.4120721361137,-1.21933992019365,-1.29163768097164));
#21329=CARTESIAN_POINT('Ctrl Pts',(91.4110341004383,-1.23048142611786,-1.28103255682529));
#21330=CARTESIAN_POINT('Ctrl Pts',(91.4104935745226,-1.23627845571372,-1.27543895896636));
#21331=CARTESIAN_POINT('Ctrl Pts',(91.4090208300729,-1.25205337650327,-1.26000901019667));
#21332=CARTESIAN_POINT('Ctrl Pts',(91.4080944865329,-1.26195350111415,-1.2500934984102));
#21333=CARTESIAN_POINT('Ctrl Pts',(91.4026309890176,-1.32012687176673,-1.1904342405566));
#21334=CARTESIAN_POINT('Ctrl Pts',(91.3982768200263,-1.36557762100826,-1.13801083333082));
#21335=CARTESIAN_POINT('Ctrl Pts',(91.3841997336238,-1.50415736935112,-0.957873106752965));
#21336=CARTESIAN_POINT('Ctrl Pts',(91.3747253165413,-1.58332890279708,-0.820413322369242));
#21337=CARTESIAN_POINT('Ctrl Pts',(91.3628929591193,-1.65292408720351,-0.650807756524253));
#21338=CARTESIAN_POINT('Ctrl Pts',(91.3612390717011,-1.66205784374785,-0.627114337891258));
#21339=CARTESIAN_POINT('Ctrl Pts',(91.3586045528446,-1.67565453493951,-0.589457781037764));
#21340=CARTESIAN_POINT('Ctrl Pts',(91.357635254108,-1.6804580860561,-0.575620704525858));
#21341=CARTESIAN_POINT('Ctrl Pts',(91.3558131153594,-1.68911436805312,-0.549653223728241));
#21342=CARTESIAN_POINT('Ctrl Pts',(91.354961723422,-1.69300893208587,-0.537537678715284));
#21343=CARTESIAN_POINT('Ctrl Pts',(91.3530404756013,-1.70145982160554,-0.510244678218971));
#21344=CARTESIAN_POINT('Ctrl Pts',(91.3519683282945,-1.70594385148206,-0.495046162841493));
#21345=CARTESIAN_POINT('Ctrl Pts',(91.3486957218741,-1.71892738420683,-0.448766036527064));
#21346=CARTESIAN_POINT('Ctrl Pts',(91.3464748878821,-1.72678463025911,-0.4175127700728));
#21347=CARTESIAN_POINT('Ctrl Pts',(91.3383938041444,-1.75197228212532,-0.304396974724843));
#21348=CARTESIAN_POINT('Ctrl Pts',(91.3323886517178,-1.76436213727278,-0.221556748651658));
#21349=CARTESIAN_POINT('Ctrl Pts',(91.318851184071,-1.77882871158686,-0.036133311173877));
#21350=CARTESIAN_POINT('Ctrl Pts',(91.311298450084,-1.77795670261595,0.0663929387965299));
#21351=CARTESIAN_POINT('Ctrl Pts',(91.3014914549188,-1.76496809820928,0.202879161166147));
#21352=CARTESIAN_POINT('Ctrl Pts',(91.2990352327657,-1.76065970613732,0.237381793567552));
#21353=CARTESIAN_POINT('Ctrl Pts',(91.2958149134345,-1.75355007352704,0.283307716586331));
#21354=CARTESIAN_POINT('Ctrl Pts',(91.2950090952338,-1.75164464678338,0.294859581185639));
#21355=CARTESIAN_POINT('Ctrl Pts',(91.2937442532734,-1.74845044291918,0.313099798006016));
#21356=CARTESIAN_POINT('Ctrl Pts',(91.2932811970449,-1.74723721852877,0.319800783322098));
#21357=CARTESIAN_POINT('Ctrl Pts',(91.2923135512147,-1.74460887521808,0.333856289440616));
#21358=CARTESIAN_POINT('Ctrl Pts',(91.2918094606678,-1.74318572793642,0.341209130491232));
#21359=CARTESIAN_POINT('Ctrl Pts',(91.2905462942246,-1.73948440211319,0.35970462812763));
#21360=CARTESIAN_POINT('Ctrl Pts',(91.2897905591451,-1.73714558373789,0.370835061012365));
#21361=CARTESIAN_POINT('Ctrl Pts',(91.2867447660612,-1.72721964964845,0.415916485012722));
#21362=CARTESIAN_POINT('Ctrl Pts',(91.2844995358084,-1.71874231725382,0.449665945880171));
#21363=CARTESIAN_POINT('Ctrl Pts',(91.278220956436,-1.69188131136068,0.544694845038104));
#21364=CARTESIAN_POINT('Ctrl Pts',(91.2742702238187,-1.67117127087735,0.605262383363768));
#21365=CARTESIAN_POINT('Ctrl Pts',(91.2621814589209,-1.59759844301491,0.787619886974256));
#21366=CARTESIAN_POINT('Ctrl Pts',(91.2541097007993,-1.53433742922395,0.904693575425017));
#21367=CARTESIAN_POINT('Ctrl Pts',(91.243882587421,-1.44385212322838,1.03490399280535));
#21368=CARTESIAN_POINT('Ctrl Pts',(91.2421959797649,-1.42860517980615,1.05585148427319));
#21369=CARTESIAN_POINT('Ctrl Pts',(91.239520953229,-1.40396148493965,1.0881976182194));
#21370=CARTESIAN_POINT('Ctrl Pts',(91.2385444676047,-1.39487102002495,1.09982576933207));
#21371=CARTESIAN_POINT('Ctrl Pts',(91.236715766698,-1.37767954658768,1.12126039952323));
#21372=CARTESIAN_POINT('Ctrl Pts',(91.2358650921355,-1.36961602115249,1.13109582118615));
#21373=CARTESIAN_POINT('Ctrl Pts',(91.2339546066057,-1.3513638053314,1.15287745578858));
#21374=CARTESIAN_POINT('Ctrl Pts',(91.2328926199139,-1.34112104741554,1.16477674725793));
#21375=CARTESIAN_POINT('Ctrl Pts',(91.2296846384023,-1.30990088729699,1.20008826832793));
#21376=CARTESIAN_POINT('Ctrl Pts',(91.2275194431717,-1.28845935797696,1.22307990355935));
#21377=CARTESIAN_POINT('Ctrl Pts',(91.2181797254625,-1.19446346038582,1.31865543700269));
#21378=CARTESIAN_POINT('Ctrl Pts',(91.2107685365086,-1.11631182134713,1.38543759136332));
#21379=CARTESIAN_POINT('Ctrl Pts',(91.1952796022268,-0.943812264325387,
1.50872754439353));
#21380=CARTESIAN_POINT('Ctrl Pts',(91.1872235286457,-0.849081913317272,
1.56400256004418));
#21381=CARTESIAN_POINT('Ctrl Pts',(91.1783627629608,-0.734399698618942,
1.61740904038376));
#21382=CARTESIAN_POINT('Ctrl Pts',(91.177178509981,-0.718835737319015,1.62438608631868));
#21383=CARTESIAN_POINT('Ctrl Pts',(91.1754021991818,-0.695095143840516,
1.63462050084888));
#21384=CARTESIAN_POINT('Ctrl Pts',(91.1748011063388,-0.686991311147375,
1.63804285276274));
#21385=CARTESIAN_POINT('Ctrl Pts',(91.1737647254907,-0.672891017507956,
1.64387453737232));
#21386=CARTESIAN_POINT('Ctrl Pts',(91.1733278330976,-0.666906513771491,
1.64631148974407));
#21387=CARTESIAN_POINT('Ctrl Pts',(91.1722957781207,-0.652673817102096,
1.6520168455186));
#21388=CARTESIAN_POINT('Ctrl Pts',(91.1717023414018,-0.644414274879106,
1.65525617961491));
#21389=CARTESIAN_POINT('Ctrl Pts',(91.1699164828718,-0.619342021985435,
1.66487322258765));
#21390=CARTESIAN_POINT('Ctrl Pts',(91.1687347436265,-0.602455842786204,
1.67105787033356));
#21391=CARTESIAN_POINT('Ctrl Pts',(91.162771832699,-0.515928927016828,1.70126659921716));
#21392=CARTESIAN_POINT('Ctrl Pts',(91.1581801474869,-0.444928778811952,
1.72120058994853));
#21393=CARTESIAN_POINT('Ctrl Pts',(91.1451208640453,-0.237936003479186,
1.76564503671502));
#21394=CARTESIAN_POINT('Ctrl Pts',(91.1367793607157,-0.100077466102164,
1.77879111975311));
#21395=CARTESIAN_POINT('Ctrl Pts',(91.1259691324007,0.0684302052589961,
1.77519386610434));
#21396=CARTESIAN_POINT('Ctrl Pts',(91.1239903103789,0.0989267311219573,
1.77375569895112));
#21397=CARTESIAN_POINT('Ctrl Pts',(91.1209554170376,0.145052983691987,1.77038723796495));
#21398=CARTESIAN_POINT('Ctrl Pts',(91.1199172749827,0.160719955518372,1.76903375032678));
#21399=CARTESIAN_POINT('Ctrl Pts',(91.118027343948,0.189026222953417,1.76620922157189));
#21400=CARTESIAN_POINT('Ctrl Pts',(91.1171778697097,0.201671733886498,1.76481002507206));
#21401=CARTESIAN_POINT('Ctrl Pts',(91.1153343871106,0.228940385422187,1.76149591092199));
#21402=CARTESIAN_POINT('Ctrl Pts',(91.1143389689357,0.243556800376245,1.75953448570266));
#21403=CARTESIAN_POINT('Ctrl Pts',(91.1115342241407,0.284428972079078,1.75353069081313));
#21404=CARTESIAN_POINT('Ctrl Pts',(91.1097122344657,0.310619992418844,1.74908113338163));
#21405=CARTESIAN_POINT('Ctrl Pts',(91.1016762603998,0.424522154356266,1.72709153131278));
#21406=CARTESIAN_POINT('Ctrl Pts',(91.0952783024372,0.510925356109155,1.70353025359939));
#21407=CARTESIAN_POINT('Ctrl Pts',(91.0817416384733,0.686325602147335,1.64115209257749));
#21408=CARTESIAN_POINT('Ctrl Pts',(91.0746066882567,0.774673825118238,1.60134435540629));
#21409=CARTESIAN_POINT('Ctrl Pts',(91.0646031844759,0.896357649723831,1.53407820097511));
#21410=CARTESIAN_POINT('Ctrl Pts',(91.0615982965574,0.932634486120392,1.51229841788795));
#21411=CARTESIAN_POINT('Ctrl Pts',(91.0577948544236,0.978571838050334,1.48243622496298));
#21412=CARTESIAN_POINT('Ctrl Pts',(91.0569340592789,0.988970018650634,1.47551968058925));
#21413=CARTESIAN_POINT('Ctrl Pts',(91.0555518560824,1.00568255691507,1.46414697219685));
#21414=CARTESIAN_POINT('Ctrl Pts',(91.0550262076812,1.01204208440103,1.45975840009881));
#21415=CARTESIAN_POINT('Ctrl Pts',(91.0539952907533,1.02452598220697,1.45102273340401));
#21416=CARTESIAN_POINT('Ctrl Pts',(91.0534898984312,1.0306517618313,1.44667806040265));
#21417=CARTESIAN_POINT('Ctrl Pts',(91.0522175478289,1.04608218375293,1.43558636768372));
#21418=CARTESIAN_POINT('Ctrl Pts',(91.0514540410584,1.05534944315585,1.42878750151326));
#21419=CARTESIAN_POINT('Ctrl Pts',(91.0483264004739,1.09330815410136,1.40036849207165));
#21420=CARTESIAN_POINT('Ctrl Pts',(91.0460102521039,1.12140847692253,1.37796882078168));
#21421=CARTESIAN_POINT('Ctrl Pts',(91.0394399909226,1.20032608829171,1.31104664658149));
#21422=CARTESIAN_POINT('Ctrl Pts',(91.0352780207815,1.24931012110267,1.26445699732421));
#21423=CARTESIAN_POINT('Ctrl Pts',(91.0233391421653,1.38228677708623,1.12268919506221));
#21424=CARTESIAN_POINT('Ctrl Pts',(91.0156033691866,1.45888449288332,1.02117568175833));
#21425=CARTESIAN_POINT('Ctrl Pts',(91.0058771395955,1.53639852186612,0.891697557030682));
#21426=CARTESIAN_POINT('Ctrl Pts',(91.0043102430581,1.54835573172312,0.87076942415628));
#21427=CARTESIAN_POINT('Ctrl Pts',(91.0017061903901,1.56733104967099,0.835930567722899));
#21428=CARTESIAN_POINT('Ctrl Pts',(91.0006779203798,1.57459875766763,0.822158901826114));
#21429=CARTESIAN_POINT('Ctrl Pts',(90.9987991609346,1.58746449824674,0.796982983104844));
#21430=CARTESIAN_POINT('Ctrl Pts',(90.9979508752841,1.59312309023943,0.785610726416097));
#21431=CARTESIAN_POINT('Ctrl Pts',(90.9961021399136,1.60512728941075,0.760822373759666));
#21432=CARTESIAN_POINT('Ctrl Pts',(90.9951001924201,1.61142765484908,0.747385569476833));
#21433=CARTESIAN_POINT('Ctrl Pts',(90.992254068052,1.62874243819139,0.709221299652784));
#21434=CARTESIAN_POINT('Ctrl Pts',(90.9903965864751,1.63936060905985,0.684319687436978));
#21435=CARTESIAN_POINT('Ctrl Pts',(90.9820411650697,1.68409381653847,0.572388993700153));
#21436=CARTESIAN_POINT('Ctrl Pts',(90.9753411044094,1.71187199064594,0.483001801999001));
#21437=CARTESIAN_POINT('Ctrl Pts',(90.960916186721,1.75557419121274,0.289784547682405));
#21438=CARTESIAN_POINT('Ctrl Pts',(90.9531908183237,1.76959579491818,0.18587013192019));
#21439=CARTESIAN_POINT('Ctrl Pts',(90.9434531987421,1.77584482714027,0.0495235656792568));
#21440=CARTESIAN_POINT('Ctrl Pts',(90.9412089529301,1.7764472631034,0.0176876180614906));
#21441=CARTESIAN_POINT('Ctrl Pts',(90.938233924654,1.776104960991,-0.025281661185769));
#21442=CARTESIAN_POINT('Ctrl Pts',(90.9374681330973,1.7759116246033,-0.0364130790099715));
#21443=CARTESIAN_POINT('Ctrl Pts',(90.9367078804582,1.77561363837197,-0.047542294091302));
#21444=CARTESIAN_POINT('Ctrl Pts',(90.7897454441732,1.7756150039535,-0.0474912648304961));
#21445=CARTESIAN_POINT('Ctrl Pts',(90.7993156250187,1.77915527271836,0.0848731680678009));
#21446=CARTESIAN_POINT('Ctrl Pts',(90.8091563929607,1.76788427360103,0.217214520202615));
#21447=CARTESIAN_POINT('Ctrl Pts',(90.8206238752608,1.73636860213996,0.375395942414399));
#21448=CARTESIAN_POINT('Ctrl Pts',(90.8226534426878,1.73003555099807,0.403578069599024));
#21449=CARTESIAN_POINT('Ctrl Pts',(90.825382050939,1.72044236685113,0.441876063702402));
#21450=CARTESIAN_POINT('Ctrl Pts',(90.8261099787572,1.71777505501923,0.452134125762967));
#21451=CARTESIAN_POINT('Ctrl Pts',(90.8273303954271,1.71311693854743,0.469412017096595));
#21452=CARTESIAN_POINT('Ctrl Pts',(90.8278255381535,1.7111744367089,0.476444478862312));
#21453=CARTESIAN_POINT('Ctrl Pts',(90.8288487216917,1.70704946125473,0.491027458977852));
#21454=CARTESIAN_POINT('Ctrl Pts',(90.8293763637131,1.70486011660728,0.498575789102205));
#21455=CARTESIAN_POINT('Ctrl Pts',(90.8307983899849,1.69879298132516,0.518986450415898));
#21456=CARTESIAN_POINT('Ctrl Pts',(90.8316874196534,1.69481916958428,0.531820024657418));
#21457=CARTESIAN_POINT('Ctrl Pts',(90.8363417341777,1.67307994049936,0.599308072673576));
#21458=CARTESIAN_POINT('Ctrl Pts',(90.8399813234926,1.65281367335895,0.653127112136689));
#21459=CARTESIAN_POINT('Ctrl Pts',(90.849886729446,1.58965465691844,0.798970979677874));
#21460=CARTESIAN_POINT('Ctrl Pts',(90.8560216604907,1.54143569642201,0.888444572145996));
#21461=CARTESIAN_POINT('Ctrl Pts',(90.865518575516,1.45741769331623,1.01670462959569));
#21462=CARTESIAN_POINT('Ctrl Pts',(90.8687634326733,1.42710939633498,1.05882615364145));
#21463=CARTESIAN_POINT('Ctrl Pts',(90.8736813970622,1.37934539289045,1.1194240156371));
#21464=CARTESIAN_POINT('Ctrl Pts',(90.8753072946828,1.36326576138031,1.13895136306727));
#21465=CARTESIAN_POINT('Ctrl Pts',(90.8783051339677,1.33315573808991,1.17396600176898));
#21466=CARTESIAN_POINT('Ctrl Pts',(90.8796717508298,1.3192584060519,1.18956193326501));
#21467=CARTESIAN_POINT('Ctrl Pts',(90.8819015095843,1.29633349395425,1.21439291759901));
#21468=CARTESIAN_POINT('Ctrl Pts',(90.8827574814467,1.28747432545772,1.22378124359616));
#21469=CARTESIAN_POINT('Ctrl Pts',(90.8844598705407,1.26974529951079,1.24216362930097));
#21470=CARTESIAN_POINT('Ctrl Pts',(90.8853060493219,1.26088025957503,1.25116128626806));
#21471=CARTESIAN_POINT('Ctrl Pts',(90.887256105412,1.24033525575579,1.2715735169381));
#21472=CARTESIAN_POINT('Ctrl Pts',(90.8883627645017,1.22859247399894,1.28292293500371));
#21473=CARTESIAN_POINT('Ctrl Pts',(90.8919891849614,1.18985457306871,1.31934354300732));
#21474=CARTESIAN_POINT('Ctrl Pts',(90.8945373036121,1.1622372349487,1.34373566898384));
#21475=CARTESIAN_POINT('Ctrl Pts',(90.9063805092729,1.032150039759,1.4516191454765));
#21476=CARTESIAN_POINT('Ctrl Pts',(90.9160771373006,0.921330794638997,1.52435925063414));
#21477=CARTESIAN_POINT('Ctrl Pts',(90.93099899312,0.739186450119857,1.61674580883643));
#21478=CARTESIAN_POINT('Ctrl Pts',(90.9362311828995,0.672944713849992,1.64542123656831));
#21479=CARTESIAN_POINT('Ctrl Pts',(90.9425284677456,0.588498383117651,1.67602115709609));
#21480=CARTESIAN_POINT('Ctrl Pts',(90.9437581926369,0.571769534773552,1.68180169016051));
#21481=CARTESIAN_POINT('Ctrl Pts',(90.9455741910302,0.546667400371461,1.69005767768158));
#21482=CARTESIAN_POINT('Ctrl Pts',(90.9461705704884,0.538358297206668,1.69272282211189));
#21483=CARTESIAN_POINT('Ctrl Pts',(90.9471961941674,0.523949119784549,1.6972277305699));
#21484=CARTESIAN_POINT('Ctrl Pts',(90.9476270477855,0.517858496607324,1.69909600371066));
#21485=CARTESIAN_POINT('Ctrl Pts',(90.9486401843571,0.50344874769937,1.70343145090378));
#21486=CARTESIAN_POINT('Ctrl Pts',(90.9492208410614,0.495121439469026,1.70587048675016));
#21487=CARTESIAN_POINT('Ctrl Pts',(90.9509465355028,0.470179782390178,1.71297777217132));
#21488=CARTESIAN_POINT('Ctrl Pts',(90.9520818175481,0.45351438768808,1.71746517586375));
#21489=CARTESIAN_POINT('Ctrl Pts',(90.9602738922053,0.331626561716199,1.74838725852858));
#21490=CARTESIAN_POINT('Ctrl Pts',(90.9669005649932,0.224230021972518,1.76537852957928));
#21491=CARTESIAN_POINT('Ctrl Pts',(90.9808220935346,-0.00210002200388923,
1.78018349565924));
#21492=CARTESIAN_POINT('Ctrl Pts',(90.9880994087397,-0.120603365252351,
1.77609345000407));
#21493=CARTESIAN_POINT('Ctrl Pts',(90.9972513888182,-0.260609268790078,
1.75717841661155));
#21494=CARTESIAN_POINT('Ctrl Pts',(90.9987541378413,-0.283341821030742,
1.75365632660867));
#21495=CARTESIAN_POINT('Ctrl Pts',(91.0011893501169,-0.319722864929306,
1.74729375446312));
#21496=CARTESIAN_POINT('Ctrl Pts',(91.0021129656754,-0.333417927353208,
1.7447322550437));
#21497=CARTESIAN_POINT('Ctrl Pts',(91.0038904278634,-0.359566695792879,
1.73952232863774));
#21498=CARTESIAN_POINT('Ctrl Pts',(91.0047433728787,-0.372024878531452,
1.73690057738642));
#21499=CARTESIAN_POINT('Ctrl Pts',(91.0067085270168,-0.400516029671903,
1.73058419533377));
#21500=CARTESIAN_POINT('Ctrl Pts',(91.0078235327917,-0.416527790364592,
1.72680031134141));
#21501=CARTESIAN_POINT('Ctrl Pts',(91.0114783602131,-0.468497957886142,
1.71375390604744));
#21502=CARTESIAN_POINT('Ctrl Pts',(91.0140467350314,-0.504216833483936,
1.70358675040614));
#21503=CARTESIAN_POINT('Ctrl Pts',(91.0258129536839,-0.66418587079092,1.65258098695349));
#21504=CARTESIAN_POINT('Ctrl Pts',(91.0353968911163,-0.783999239892148,
1.59921925682782));
#21505=CARTESIAN_POINT('Ctrl Pts',(91.0501408458299,-0.958411538080903,
1.49719668595346));
#21506=CARTESIAN_POINT('Ctrl Pts',(91.0553093936267,-1.01775421874025,1.45750776177013));
#21507=CARTESIAN_POINT('Ctrl Pts',(91.0615464072451,-1.08862420808789,1.40366435983973));
#21508=CARTESIAN_POINT('Ctrl Pts',(91.062773776462,-1.102534701564,1.39276472971141));
#21509=CARTESIAN_POINT('Ctrl Pts',(91.0645907447932,-1.12310526886498,1.37614519228709));
#21510=CARTESIAN_POINT('Ctrl Pts',(91.0651902598137,-1.12988891792469,1.37058092667042));
#21511=CARTESIAN_POINT('Ctrl Pts',(91.0662214400196,-1.14155519739722,1.36086621361119));
#21512=CARTESIAN_POINT('Ctrl Pts',(91.0666547216233,-1.14645689026059,1.35673937159642));
#21513=CARTESIAN_POINT('Ctrl Pts',(91.0676744828321,-1.15799256532709,1.34692007445035));
#21514=CARTESIAN_POINT('Ctrl Pts',(91.0682593135512,-1.16460699039142,1.34120506795032));
#21515=CARTESIAN_POINT('Ctrl Pts',(91.07000889991,-1.18438009603199,1.32386409729363));
#21516=CARTESIAN_POINT('Ctrl Pts',(91.0711635170415,-1.19740928661618,1.31209123819717));
#21517=CARTESIAN_POINT('Ctrl Pts',(91.0810075772964,-1.30807008317365,1.20907927089604));
#21518=CARTESIAN_POINT('Ctrl Pts',(91.0890477692518,-1.39530515361664,1.10727307526567));
#21519=CARTESIAN_POINT('Ctrl Pts',(91.1026245749139,-1.51895616421602,0.924854279858832));
#21520=CARTESIAN_POINT('Ctrl Pts',(91.1080248078927,-1.56228351631279,0.849618165046805));
#21521=CARTESIAN_POINT('Ctrl Pts',(91.1153014577173,-1.61127777820839,0.748016782202922));
#21522=CARTESIAN_POINT('Ctrl Pts',(91.1170009637716,-1.62209375827819,0.72426301186416));
#21523=CARTESIAN_POINT('Ctrl Pts',(91.1196765795121,-1.63812370243641,0.686896567880262));
#21524=CARTESIAN_POINT('Ctrl Pts',(91.1206403445507,-1.64370036256524,0.673442838195278));
#21525=CARTESIAN_POINT('Ctrl Pts',(91.1224484752508,-1.65379220488112,0.64822386283719));
#21526=CARTESIAN_POINT('Ctrl Pts',(91.1232913756476,-1.65834886571468,0.636476125820999));
#21527=CARTESIAN_POINT('Ctrl Pts',(91.1251884143469,-1.66827195313591,0.610062792260358));
#21528=CARTESIAN_POINT('Ctrl Pts',(91.126244737964,-1.67357067726382,0.595373060460751));
#21529=CARTESIAN_POINT('Ctrl Pts',(91.1289750988566,-1.68668371149883,0.557460688465905));
#21530=CARTESIAN_POINT('Ctrl Pts',(91.1306583184987,-1.69421222029347,0.534143436105127));
#21531=CARTESIAN_POINT('Ctrl Pts',(91.1403000899471,-1.73419655206887,0.400941197229571));
#21532=CARTESIAN_POINT('Ctrl Pts',(91.1485802151878,-1.75643712083253,0.288291544750243));
#21533=CARTESIAN_POINT('Ctrl Pts',(91.1625186589797,-1.77514871567458,0.0985316822635118));
#21534=CARTESIAN_POINT('Ctrl Pts',(91.1681042828945,-1.77774089524666,0.0223536772101882));
#21535=CARTESIAN_POINT('Ctrl Pts',(91.1754304370838,-1.77464885383945,-0.079765291498497));
#21536=CARTESIAN_POINT('Ctrl Pts',(91.1772803545186,-1.77328999568864,-0.105753436881783));
#21537=CARTESIAN_POINT('Ctrl Pts',(91.1804285438643,-1.76996541504043,-0.150467698956513));
#21538=CARTESIAN_POINT('Ctrl Pts',(91.1817375241805,-1.76827214033286,-0.169209359045446));
#21539=CARTESIAN_POINT('Ctrl Pts',(91.1836488818063,-1.76533162411925,-0.196847385115945));
#21540=CARTESIAN_POINT('Ctrl Pts',(91.184262749798,-1.76431428960216,-0.205766208150988));
#21541=CARTESIAN_POINT('Ctrl Pts',(91.185355345103,-1.76237147708351,-0.221723303105304));
#21542=CARTESIAN_POINT('Ctrl Pts',(91.185835408436,-1.76147137713992,-0.228764155432254));
#21543=CARTESIAN_POINT('Ctrl Pts',(91.1869089823393,-1.75935355041328,-0.244576276104114));
#21544=CARTESIAN_POINT('Ctrl Pts',(91.1875011917161,-1.75811241872631,-0.253344038158499));
#21545=CARTESIAN_POINT('Ctrl Pts',(91.1892998221417,-1.75412098211091,-0.28009762437475));
#21546=CARTESIAN_POINT('Ctrl Pts',(91.1904952089221,-1.75115976344716,-0.298051413525627));
#21547=CARTESIAN_POINT('Ctrl Pts',(91.197344592085,-1.7324262782389,-0.401687832087028));
#21548=CARTESIAN_POINT('Ctrl Pts',(91.2027297192348,-1.71064128653493,-0.486172733150881));
#21549=CARTESIAN_POINT('Ctrl Pts',(91.2132249058077,-1.65597225645751,-0.647926919155193));
#21550=CARTESIAN_POINT('Ctrl Pts',(91.2183254886979,-1.62364639111528,-0.725138034746177));
#21551=CARTESIAN_POINT('Ctrl Pts',(91.2273611868068,-1.55857906432791,-0.854169454192178));
#21552=CARTESIAN_POINT('Ctrl Pts',(91.2312294257906,-1.52837645285302,-0.90710440496241));
#21553=CARTESIAN_POINT('Ctrl Pts',(91.2364776654948,-1.48487942067013,-0.974979942292468));
#21554=CARTESIAN_POINT('Ctrl Pts',(91.2377707343639,-1.47396634509887,-0.991401000757056));
#21555=CARTESIAN_POINT('Ctrl Pts',(91.2399485013833,-1.45527836540388,-1.01853027896938));
#21556=CARTESIAN_POINT('Ctrl Pts',(91.2408275083637,-1.44765290318997,-1.02933964547821));
#21557=CARTESIAN_POINT('Ctrl Pts',(91.2425716951597,-1.43236502743538,-1.0505048412973));
#21558=CARTESIAN_POINT('Ctrl Pts',(91.2434365811453,-1.42470927311038,-1.06086448961843));
#21559=CARTESIAN_POINT('Ctrl Pts',(91.245361652411,-1.40750810549772,-1.08361880545344));
#21560=CARTESIAN_POINT('Ctrl Pts',(91.2464238557884,-1.39791034918522,-1.0959723586013));
#21561=CARTESIAN_POINT('Ctrl Pts',(91.2501469784148,-1.36390926762477,-1.13856282315742));
#21562=CARTESIAN_POINT('Ctrl Pts',(91.2528405448028,-1.33867953992551,-1.16812262851464));
#21563=CARTESIAN_POINT('Ctrl Pts',(91.2646089437274,-1.22582337815656,-1.29188628180531));
#21564=CARTESIAN_POINT('Ctrl Pts',(91.2740474102044,-1.12908387016809,-1.37723409169065));
#21565=CARTESIAN_POINT('Ctrl Pts',(91.2885987568033,-0.966196861288616,
-1.49215673627703));
#21566=CARTESIAN_POINT('Ctrl Pts',(91.2937255126596,-0.906005389609694,
-1.52945227319384));
#21567=CARTESIAN_POINT('Ctrl Pts',(91.2999162989816,-0.828269812292595,
-1.57141414748713));
#21568=CARTESIAN_POINT('Ctrl Pts',(91.3011378243745,-0.812671205839852,
-1.57953755085097));
#21569=CARTESIAN_POINT('Ctrl Pts',(91.3029464755025,-0.789146324290969,
-1.59134800155561));
#21570=CARTESIAN_POINT('Ctrl Pts',(91.3035434700806,-0.78130981805221,-1.59521013021559));
#21571=CARTESIAN_POINT('Ctrl Pts',(91.3045709630611,-0.767692545719014,
-1.60179681907707));
#21572=CARTESIAN_POINT('Ctrl Pts',(91.3050030627059,-0.761925263122236,
-1.60454815791507));
#21573=CARTESIAN_POINT('Ctrl Pts',(91.3060207313517,-0.748246150753339,
-1.61098352616868));
#21574=CARTESIAN_POINT('Ctrl Pts',(91.3066046484938,-0.740321869038026,
-1.61464044355246));
#21575=CARTESIAN_POINT('Ctrl Pts',(91.3083504580245,-0.716414239633213,
-1.62546038392408));
#21576=CARTESIAN_POINT('Ctrl Pts',(91.309502253525,-0.700351052286214,-1.63244579779591));
#21577=CARTESIAN_POINT('Ctrl Pts',(91.31936204865,-0.560615594713262,-1.69077030085083));
#21578=CARTESIAN_POINT('Ctrl Pts',(91.3274167848657,-0.431591433690345,
-1.72821673450586));
#21579=CARTESIAN_POINT('Ctrl Pts',(91.3410055552292,-0.214161570667849,
-1.76541974707872));
#21580=CARTESIAN_POINT('Ctrl Pts',(91.346401617071,-0.127808459809235,-1.77376283747623));
#21581=CARTESIAN_POINT('Ctrl Pts',(91.3536733281398,-0.0151143994283971,
-1.77637729589402));
#21582=CARTESIAN_POINT('Ctrl Pts',(91.3553722371953,0.0109774259569875,
-1.77640764595333));
#21583=CARTESIAN_POINT('Ctrl Pts',(91.3580469835552,0.0516160836335758,
-1.77555958264593));
#21584=CARTESIAN_POINT('Ctrl Pts',(91.3590104801715,0.0661680972872522,
-1.77507684715068));
#21585=CARTESIAN_POINT('Ctrl Pts',(91.3608181354188,0.0932968062942999,
-1.773842853534));
#21586=CARTESIAN_POINT('Ctrl Pts',(91.3616608294583,0.105874702123737,-1.77313657015911));
#21587=CARTESIAN_POINT('Ctrl Pts',(91.3635574396542,0.134022029597899,-1.77125546572881));
#21588=CARTESIAN_POINT('Ctrl Pts',(91.3646135409346,0.149585457152417,-1.77000903757965));
#21589=CARTESIAN_POINT('Ctrl Pts',(91.3673434427241,0.189522100166671,-1.76628015817118));
#21590=CARTESIAN_POINT('Ctrl Pts',(91.3690264243102,0.21386334589933,-1.76349839490747));
#21591=CARTESIAN_POINT('Ctrl Pts',(91.3786075067603,0.350818407721299,-1.74496983218926));
#21592=CARTESIAN_POINT('Ctrl Pts',(91.3868217643885,0.461756225916469,-1.71894342012451));
#21593=CARTESIAN_POINT('Ctrl Pts',(91.4007270838061,0.641979138753719,-1.65794853929313));
#21594=CARTESIAN_POINT('Ctrl Pts',(91.4063461578826,0.712868366638673,-1.62872655169136));
#21595=CARTESIAN_POINT('Ctrl Pts',(91.4137106856654,0.805088233832541,-1.58353344145636));
#21596=CARTESIAN_POINT('Ctrl Pts',(91.4155663519107,0.828269702049839,-1.57153258576421));
#21597=CARTESIAN_POINT('Ctrl Pts',(91.418723233832,0.867731944495391,-1.54998741662749));
#21598=CARTESIAN_POINT('Ctrl Pts',(91.4200352228598,0.884140340749637,-1.54068674559509));
#21599=CARTESIAN_POINT('Ctrl Pts',(91.4219502136567,0.908144372133074,-1.52657086746632));
#21600=CARTESIAN_POINT('Ctrl Pts',(91.4225647562539,0.91585599019513,-1.52195684171674));
#21601=CARTESIAN_POINT('Ctrl Pts',(91.4236583073059,0.929599408262028,-1.51359157211002));
#21602=CARTESIAN_POINT('Ctrl Pts',(91.4241386558857,0.935644085722084,-1.50986246285927));
#21603=CARTESIAN_POINT('Ctrl Pts',(91.4252126553516,0.949176472692837,-1.50140152253524));
#21604=CARTESIAN_POINT('Ctrl Pts',(91.4258050071342,0.956651334779626,-1.49664983887793));
#21605=CARTESIAN_POINT('Ctrl Pts',(91.4276031406114,0.979363596454923,-1.48197223093913));
#21606=CARTESIAN_POINT('Ctrl Pts',(91.4287979145563,0.994484913052898,-1.4718677141785));
#21607=CARTESIAN_POINT('Ctrl Pts',(91.4358963299324,1.08428866150907,-1.40984218554888));
#21608=CARTESIAN_POINT('Ctrl Pts',(91.441506083376,1.15505690375489,-1.35247345616729));
#21609=CARTESIAN_POINT('Ctrl Pts',(91.4545791935594,1.30958876101723,-1.20618419841582));
#21610=CARTESIAN_POINT('Ctrl Pts',(91.4620087480821,1.38919431205177,-1.11357029454688));
#21611=CARTESIAN_POINT('Ctrl Pts',(91.4717593981496,1.4758604047627,-0.988840260840585));
#21612=CARTESIAN_POINT('Ctrl Pts',(91.4737110491638,1.49239431445975,-0.963705367367069));
#21613=CARTESIAN_POINT('Ctrl Pts',(91.4766942346479,1.51638898607544,-0.925129256983195));
#21614=CARTESIAN_POINT('Ctrl Pts',(91.4777082113679,1.52432712609382,-0.911990398599405));
#21615=CARTESIAN_POINT('Ctrl Pts',(91.4794834949495,1.53784204527992,-0.888951612777335));
#21616=CARTESIAN_POINT('Ctrl Pts',(91.4802419401809,1.54349605317321,-0.87909786122651));
#21617=CARTESIAN_POINT('Ctrl Pts',(91.4819631056009,1.55605438883789,-0.85671663679039));
#21618=CARTESIAN_POINT('Ctrl Pts',(91.4829277735815,1.56290262352812,-0.844158767808961));
#21619=CARTESIAN_POINT('Ctrl Pts',(91.4855404856088,1.58093549419929,-0.810119457861819));
#21620=CARTESIAN_POINT('Ctrl Pts',(91.4871984411343,1.59183333756537,-0.788490391335275));
#21621=CARTESIAN_POINT('Ctrl Pts',(91.4989289802033,1.66511590629817,-0.635330338555039));
#21622=CARTESIAN_POINT('Ctrl Pts',(91.509555776627,1.71155443579279,-0.496810776419606));
#21623=CARTESIAN_POINT('Ctrl Pts',(91.5243665717549,1.75197377673693,-0.298194959594751));
#21624=CARTESIAN_POINT('Ctrl Pts',(91.5285278224775,1.76066374846439,-0.241653201940884));
#21625=CARTESIAN_POINT('Ctrl Pts',(91.5349198382908,1.7699848913351,-0.152541081512852));
#21626=CARTESIAN_POINT('Ctrl Pts',(91.537205049005,1.77247461432816,-0.12020546207983));
#21627=CARTESIAN_POINT('Ctrl Pts',(91.5402117281035,1.77462319028804,-0.0768002173295743));
#21628=CARTESIAN_POINT('Ctrl Pts',(91.5409700025633,1.77506592803839,-0.0657777142948062));
#21629=CARTESIAN_POINT('Ctrl Pts',(91.541886871471,1.77548006742821,-0.052348562860265));
#21630=CARTESIAN_POINT('Ctrl Pts',(91.5420506674495,1.7755492920597,-0.0499455056259374));
#21631=CARTESIAN_POINT('Ctrl Pts',(91.5422141974348,1.77561363837091,-0.0475422941309033));
#21632=CARTESIAN_POINT('Origin',(88.3562164250559,0.,0.));
#21633=CARTESIAN_POINT('',(92.4397243119761,1.77561363837197,-0.0475422940913782));
#21634=CARTESIAN_POINT('',(92.2900876926257,1.77561363857513,-0.047542286503657));
#21635=CARTESIAN_POINT('',(88.3562164250559,1.77561363837197,-0.0475422940912398));
#21636=CARTESIAN_POINT('',(92.4397193140361,1.77561154215721,-0.047620519296831));
#21637=CARTESIAN_POINT('Ctrl Pts',(92.4397243119761,1.77561363837196,-0.0475422940915214));
#21638=CARTESIAN_POINT('Ctrl Pts',(92.4397224335513,1.77561285117158,-0.0475716945183764));
#21639=CARTESIAN_POINT('Ctrl Pts',(92.4397211924972,1.77561233065394,-0.0475911188635325));
#21640=CARTESIAN_POINT('Ctrl Pts',(92.4397193140361,1.77561154215721,-0.0476205192968057));
#21641=CARTESIAN_POINT('Ctrl Pts',(92.4397193140361,1.77561154215721,-0.0476205192967044));
#21642=CARTESIAN_POINT('Ctrl Pts',(92.4384162706077,1.77506458088494,-0.0680148947152969));
#21643=CARTESIAN_POINT('Ctrl Pts',(92.4371048348684,1.77416680544134,-0.0883877160786648));
#21644=CARTESIAN_POINT('Ctrl Pts',(92.4347613706043,1.77195318636845,-0.124475693326451));
#21645=CARTESIAN_POINT('Ctrl Pts',(92.4337342110471,1.77077941231963,-0.140187519064086));
#21646=CARTESIAN_POINT('Ctrl Pts',(92.4318637772838,1.76827725088801,-0.168589370914655));
#21647=CARTESIAN_POINT('Ctrl Pts',(92.4310227541361,1.76702083497391,-0.181284766744872));
#21648=CARTESIAN_POINT('Ctrl Pts',(92.4293764235636,1.76430771801814,-0.205981739748837));
#21649=CARTESIAN_POINT('Ctrl Pts',(92.4285715967944,1.76286502317096,-0.217984170741241));
#21650=CARTESIAN_POINT('Ctrl Pts',(92.4268572589327,1.75954733667217,-0.243393674222738));
#21651=CARTESIAN_POINT('Ctrl Pts',(92.4259468177277,1.75764136986009,-0.256795848774373));
#21652=CARTESIAN_POINT('Ctrl Pts',(92.4236283969233,1.75242632634737,-0.290682966275401));
#21653=CARTESIAN_POINT('Ctrl Pts',(92.422213995457,1.74891120659691,-0.311133643018388));
#21654=CARTESIAN_POINT('Ctrl Pts',(92.4162767462431,1.73278400641467,-0.396023898322558));
#21655=CARTESIAN_POINT('Ctrl Pts',(92.411654521346,1.7169634042702,-0.459793615133651));
#21656=CARTESIAN_POINT('Ctrl Pts',(92.4021046474298,1.67778014761543,-0.587095150418172));
#21657=CARTESIAN_POINT('Ctrl Pts',(92.3971795864593,1.65424325619602,-0.650465327122878));
#21658=CARTESIAN_POINT('Ctrl Pts',(92.3870494763906,1.59869069907259,-0.777361262422159));
#21659=CARTESIAN_POINT('Ctrl Pts',(92.3818517147233,1.56635116142991,-0.840623247298179));
#21660=CARTESIAN_POINT('Ctrl Pts',(92.3741186200029,1.51154005078284,-0.933636861374367));
#21661=CARTESIAN_POINT('Ctrl Pts',(92.3715033217727,1.49177731797006,-0.964899991260372));
#21662=CARTESIAN_POINT('Ctrl Pts',(92.3681370516592,1.46454397456659,-1.0051416930856));
#21663=CARTESIAN_POINT('Ctrl Pts',(92.3673380194824,1.45794209507266,-1.01469391551458));
#21664=CARTESIAN_POINT('Ctrl Pts',(92.3660301905661,1.44690034856385,-1.03033987932306));
#21665=CARTESIAN_POINT('Ctrl Pts',(92.3655179241297,1.44251460618257,-1.03647117820593));
#21666=CARTESIAN_POINT('Ctrl Pts',(92.3645510806996,1.43411867500942,-1.04805222363226));
#21667=CARTESIAN_POINT('Ctrl Pts',(92.3640959731004,1.43011616954989,-1.05350727712053));
#21668=CARTESIAN_POINT('Ctrl Pts',(92.3628748512699,1.41924380007105,-1.06814918703678));
#21669=CARTESIAN_POINT('Ctrl Pts',(92.3621127479233,1.41231581214442,-1.07729277073242));
#21670=CARTESIAN_POINT('Ctrl Pts',(92.3591889681092,1.38520712231163,-1.1123598907171));
#21671=CARTESIAN_POINT('Ctrl Pts',(92.3570665068653,1.36439604486501,-1.13779042438384));
#21672=CARTESIAN_POINT('Ctrl Pts',(92.3483628942292,1.2749303647725,-1.24112724157452));
#21673=CARTESIAN_POINT('Ctrl Pts',(92.3420620211534,1.20021345764129,-1.31352028679284));
#21674=CARTESIAN_POINT('Ctrl Pts',(92.3299537090243,1.04735027494071,-1.43763036408985));
#21675=CARTESIAN_POINT('Ctrl Pts',(92.3241814717585,0.970616776156143,-1.49051130918445));
#21676=CARTESIAN_POINT('Ctrl Pts',(92.3164452519067,0.86671287661616,-1.55067830307281));
#21677=CARTESIAN_POINT('Ctrl Pts',(92.3146870482974,0.843021022140021,-1.5636846997781));
#21678=CARTESIAN_POINT('Ctrl Pts',(92.311933916625,0.805875972799583,-1.58298709867434));
#21679=CARTESIAN_POINT('Ctrl Pts',(92.3109524128512,0.792624410471672,-1.58966372531649));
#21680=CARTESIAN_POINT('Ctrl Pts',(92.3091191482691,0.767867302141811,-1.60175075424609));
#21681=CARTESIAN_POINT('Ctrl Pts',(92.3082689936447,0.756384235853919,-1.60720519712905));
#21682=CARTESIAN_POINT('Ctrl Pts',(92.3063659496786,0.730681675707032,-1.6190774261403));
#21683=CARTESIAN_POINT('Ctrl Pts',(92.3053109631407,0.716434333570718,-1.62543201691363));
#21684=CARTESIAN_POINT('Ctrl Pts',(92.3026042941029,0.679895886453454,-1.64115515855599));
#21685=CARTESIAN_POINT('Ctrl Pts',(92.3009438184613,0.657494423553019,-1.65025745075125));
#21686=CARTESIAN_POINT('Ctrl Pts',(92.2905656268471,0.517623478910721,-1.70379064120068));
#21687=CARTESIAN_POINT('Ctrl Pts',(92.2814529765301,0.395921060732133,-1.7361084800252));
#21688=CARTESIAN_POINT('Ctrl Pts',(92.267278649882,0.20439943424351,-1.7657701042476));
#21689=CARTESIAN_POINT('Ctrl Pts',(92.2622855257097,0.136396408661462,-1.77232054561005));
#21690=CARTESIAN_POINT('Ctrl Pts',(92.2548117718038,0.0320607790416382,
-1.77632847661682));
#21691=CARTESIAN_POINT('Ctrl Pts',(92.2522564444011,-0.00409766566065642,
-1.77661317659523));
#21692=CARTESIAN_POINT('Ctrl Pts',(92.2489541773622,-0.0517623354439688,
-1.77553301907567));
#21693=CARTESIAN_POINT('Ctrl Pts',(92.2481613400909,-0.0632799178735311,
-1.77515985504275));
#21694=CARTESIAN_POINT('Ctrl Pts',(92.2468609329884,-0.0823066235505851,
-1.77435797699596));
#21695=CARTESIAN_POINT('Ctrl Pts',(92.2463499683301,-0.0898179543904061,
-1.77399361690382));
#21696=CARTESIAN_POINT('Ctrl Pts',(92.2453833914227,-0.104098400217065,
-1.77320996382178));
#21697=CARTESIAN_POINT('Ctrl Pts',(92.2449272701061,-0.110867781690771,
-1.7727995914977));
#21698=CARTESIAN_POINT('Ctrl Pts',(92.2436995390321,-0.129165743014583,
-1.77158511563581));
#21699=CARTESIAN_POINT('Ctrl Pts',(92.2429319165576,-0.140689334039717,
-1.77070724290043));
#21700=CARTESIAN_POINT('Ctrl Pts',(92.2399587098838,-0.185606528062117,
-1.76684415461661));
#21701=CARTESIAN_POINT('Ctrl Pts',(92.2377940490086,-0.218923658287862,
-1.76302604027329));
#21702=CARTESIAN_POINT('Ctrl Pts',(92.2290880227354,-0.35436489857077,-1.74360533218544));
#21703=CARTESIAN_POINT('Ctrl Pts',(92.2228194346928,-0.455149079117714,
-1.72005141200978));
#21704=CARTESIAN_POINT('Ctrl Pts',(92.2107594851322,-0.641495395311842,
-1.65896291784003));
#21705=CARTESIAN_POINT('Ctrl Pts',(92.2050028075449,-0.72725959327133,-1.62319593042249));
#21706=CARTESIAN_POINT('Ctrl Pts',(92.1972855347556,-0.833855371826907,
-1.56859102934989));
#21707=CARTESIAN_POINT('Ctrl Pts',(92.1955294564356,-0.857593521728362,
-1.5557396390121));
#21708=CARTESIAN_POINT('Ctrl Pts',(92.1927789247224,-0.893907181450863,
-1.53499641293168));
#21709=CARTESIAN_POINT('Ctrl Pts',(92.1917978537178,-0.906692706365165,
-1.5274790835144));
#21710=CARTESIAN_POINT('Ctrl Pts',(92.1899649883115,-0.930259828558774,
-1.51322249990443));
#21711=CARTESIAN_POINT('Ctrl Pts',(92.1891147944941,-0.941066170781586,
-1.50652584795496));
#21712=CARTESIAN_POINT('Ctrl Pts',(92.1872111332242,-0.964977858574336,
-1.49135019931309));
#21713=CARTESIAN_POINT('Ctrl Pts',(92.1861555619857,-0.978045060928342,
-1.48281337873496));
#21714=CARTESIAN_POINT('Ctrl Pts',(92.1834463158229,-1.01108734797192,-1.46060002531754));
#21715=CARTESIAN_POINT('Ctrl Pts',(92.1817838188473,-1.03089788655939,-1.44668569710708));
#21716=CARTESIAN_POINT('Ctrl Pts',(92.1714366396688,-1.15130334514369,-1.35838740749496));
#21717=CARTESIAN_POINT('Ctrl Pts',(92.1623604611292,-1.24407428406101,-1.27396411046387));
#21718=CARTESIAN_POINT('Ctrl Pts',(92.1481988293956,-1.37276474707537,-1.12928405745019));
#21719=CARTESIAN_POINT('Ctrl Pts',(92.1431824620932,-1.41533280276073,-1.07545316019012));
#21720=CARTESIAN_POINT('Ctrl Pts',(92.1356791453553,-1.47548174532882,-0.989611672438018));
#21721=CARTESIAN_POINT('Ctrl Pts',(92.1331169037432,-1.49536823517074,-0.959297611233721));
#21722=CARTESIAN_POINT('Ctrl Pts',(92.129807246919,-1.52034270328216,-0.918561452719356));
#21723=CARTESIAN_POINT('Ctrl Pts',(92.1290136870216,-1.52627508130396,-0.90867016669605));
#21724=CARTESIAN_POINT('Ctrl Pts',(92.1277124146958,-1.53591675303896,-0.892233360974677));
#21725=CARTESIAN_POINT('Ctrl Pts',(92.1272012987223,-1.5396814794406,-0.885720944473918));
#21726=CARTESIAN_POINT('Ctrl Pts',(92.1261712376869,-1.54722530287246,-0.872477794520266));
#21727=CARTESIAN_POINT('Ctrl Pts',(92.1256524343739,-1.55100210368083,-0.865745990399245));
#21728=CARTESIAN_POINT('Ctrl Pts',(92.1243036408515,-1.56075713798443,-0.848089789612762));
#21729=CARTESIAN_POINT('Ctrl Pts',(92.1234779701487,-1.5666647051273,-0.837126548687118));
#21730=CARTESIAN_POINT('Ctrl Pts',(92.1199010174589,-1.59194656589751,-0.78900338062029));
#21731=CARTESIAN_POINT('Ctrl Pts',(92.1172148760661,-1.6101192078813,-0.751223636607381));
#21732=CARTESIAN_POINT('Ctrl Pts',(92.1084501943705,-1.66587078188128,-0.623978655682495));
#21733=CARTESIAN_POINT('Ctrl Pts',(92.1025620093898,-1.69745960757359,-0.532078969323977));
#21734=CARTESIAN_POINT('Ctrl Pts',(92.0910776878918,-1.74347711518394,-0.351247802887306));
#21735=CARTESIAN_POINT('Ctrl Pts',(92.0855099249027,-1.7589674342231,-0.262903850354378));
#21736=CARTESIAN_POINT('Ctrl Pts',(92.0780227141735,-1.77032938296649,-0.147323908230554));
#21737=CARTESIAN_POINT('Ctrl Pts',(92.0762928336041,-1.77233546264824,-0.120819476066508));
#21738=CARTESIAN_POINT('Ctrl Pts',(92.0735743674978,-1.77452885493572,-0.0795543536124082));
#21739=CARTESIAN_POINT('Ctrl Pts',(92.0725986530132,-1.77512817862992,-0.0648188210614253));
#21740=CARTESIAN_POINT('Ctrl Pts',(92.0707706890069,-1.77590251252812,-0.0373643176233218));
#21741=CARTESIAN_POINT('Ctrl Pts',(92.0699199705932,-1.77612451990107,-0.0246475458464306));
#21742=CARTESIAN_POINT('Ctrl Pts',(92.0680084594704,-1.77631548099647,0.00378444383170876));
#21743=CARTESIAN_POINT('Ctrl Pts',(92.0669454794358,-1.77621248026179,0.0194989044897602));
#21744=CARTESIAN_POINT('Ctrl Pts',(92.0642034855025,-1.77541391757267,0.0597769061715121));
#21745=CARTESIAN_POINT('Ctrl Pts',(92.0625152782607,-1.77441712425732,0.0843304295636668));
#21746=CARTESIAN_POINT('Ctrl Pts',(92.0528664235511,-1.76588863718058,0.223233950027916));
#21747=CARTESIAN_POINT('Ctrl Pts',(92.044584243175,-1.74781483915964,0.336647026443929));
#21748=CARTESIAN_POINT('Ctrl Pts',(92.0306709074447,-1.69985930938506,0.520850913337519));
#21749=CARTESIAN_POINT('Ctrl Pts',(92.025112149224,-1.67609131359707,0.592896423639816));
#21750=CARTESIAN_POINT('Ctrl Pts',(92.0169265218084,-1.63346964055078,0.698793715386502));
#21751=CARTESIAN_POINT('Ctrl Pts',(92.0142102350385,-1.61799578438501,0.733911340574197));
#21752=CARTESIAN_POINT('Ctrl Pts',(92.0107366429896,-1.59630998077861,0.77909990690063));
#21753=CARTESIAN_POINT('Ctrl Pts',(92.0099275351686,-1.59111931043537,0.789646489521547));
#21754=CARTESIAN_POINT('Ctrl Pts',(92.0086076132218,-1.58241495787134,0.806897912043264));
#21755=CARTESIAN_POINT('Ctrl Pts',(92.0080932070205,-1.57896251896122,0.813633031136685));
#21756=CARTESIAN_POINT('Ctrl Pts',(92.0071258091406,-1.57235359692246,0.826325404927407));
#21757=CARTESIAN_POINT('Ctrl Pts',(92.0066722527021,-1.56920607109502,0.832287101226458));
#21758=CARTESIAN_POINT('Ctrl Pts',(92.0054613674507,-1.56067364376164,0.848227806669165));
#21759=CARTESIAN_POINT('Ctrl Pts',(92.0047078318479,-1.55522689698367,0.858173612959993));
#21760=CARTESIAN_POINT('Ctrl Pts',(92.0018590678015,-1.53412877686555,0.895838270487618));
#21761=CARTESIAN_POINT('Ctrl Pts',(91.9998005364955,-1.51782759656934,0.923188491452394));
#21762=CARTESIAN_POINT('Ctrl Pts',(91.9910999242232,-1.44482855201506,1.03850089019707));
#21763=CARTESIAN_POINT('Ctrl Pts',(91.9847497337416,-1.38115017437794,1.12180285336836));
#21764=CARTESIAN_POINT('Ctrl Pts',(91.9725676513696,-1.2474138892642,1.26797382925055));
#21765=CARTESIAN_POINT('Ctrl Pts',(91.9667717445636,-1.17898821282085,1.33183446579999));
#21766=CARTESIAN_POINT('Ctrl Pts',(91.9590067018434,-1.08467317627199,1.40686931300259));
#21767=CARTESIAN_POINT('Ctrl Pts',(91.9572452735813,-1.06310318272823,1.42323879210941));
#21768=CARTESIAN_POINT('Ctrl Pts',(91.954488196641,-1.02913811600939,1.44781189456886));
#21769=CARTESIAN_POINT('Ctrl Pts',(91.9535060359196,-1.01699950088809,1.4563641497182));
#21770=CARTESIAN_POINT('Ctrl Pts',(91.9516721632255,-0.994272599941517,
1.47195368622833));
#21771=CARTESIAN_POINT('Ctrl Pts',(91.9508220659182,-0.98371315790604,1.47903146209307));
#21772=CARTESIAN_POINT('Ctrl Pts',(91.9489199497421,-0.960038605580013,
1.49453434400107));
#21773=CARTESIAN_POINT('Ctrl Pts',(91.9478658436122,-0.946886861040254,
1.50290128582479));
#21774=CARTESIAN_POINT('Ctrl Pts',(91.9451630555746,-0.913094508367213,
1.52377984036966));
#21775=CARTESIAN_POINT('Ctrl Pts',(91.9435056240067,-0.892306451459931,
1.53604546815214));
#21776=CARTESIAN_POINT('Ctrl Pts',(91.9330833336318,-0.761233467836146,
1.6098241072713));
#21777=CARTESIAN_POINT('Ctrl Pts',(91.9239185934707,-0.644917891274431,
1.65984346453568));
#21778=CARTESIAN_POINT('Ctrl Pts',(91.9097259041086,-0.45950959129633,1.71712390057367));
#21779=CARTESIAN_POINT('Ctrl Pts',(91.9047656930783,-0.393615351687797,
1.73341611071753));
#21780=CARTESIAN_POINT('Ctrl Pts',(91.8973338477697,-0.291550667199426,
1.75252936755916));
#21781=CARTESIAN_POINT('Ctrl Pts',(91.8947883560639,-0.255956960426443,
1.75808060841535));
#21782=CARTESIAN_POINT('Ctrl Pts',(91.8914966051869,-0.208796860709239,
1.76397289517714));
#21783=CARTESIAN_POINT('Ctrl Pts',(91.8907047988677,-0.197363344843533,
1.76528871060033));
#21784=CARTESIAN_POINT('Ctrl Pts',(91.8894056252635,-0.178441910814071,
1.76728012776684));
#21785=CARTESIAN_POINT('Ctrl Pts',(91.8888948755928,-0.170961204841223,
1.76801946792131));
#21786=CARTESIAN_POINT('Ctrl Pts',(91.8878647521115,-0.155783411864449,
1.76942229819417));
#21787=CARTESIAN_POINT('Ctrl Pts',(91.8873455279225,-0.148086286713316,
1.77008310488363));
#21788=CARTESIAN_POINT('Ctrl Pts',(91.8859943474189,-0.127941197248894,
1.77168025666717));
#21789=CARTESIAN_POINT('Ctrl Pts',(91.8851667387025,-0.115486991149258,
1.77253565793019));
#21790=CARTESIAN_POINT('Ctrl Pts',(91.8815657708556,-0.0608501975413613,
1.77570999332726));
#21791=CARTESIAN_POINT('Ctrl Pts',(91.8788586490298,-0.0185982483418953,
1.77665513193569));
#21792=CARTESIAN_POINT('Ctrl Pts',(91.8753622020439,0.0368335383901947,
1.77591699439609));
#21793=CARTESIAN_POINT('Ctrl Pts',(91.8745349087929,0.0500142549386234,
1.77559467993379));
#21794=CARTESIAN_POINT('Ctrl Pts',(91.8633664011248,0.228615926543652,1.769236870932));
#21795=CARTESIAN_POINT('Ctrl Pts',(91.8535216497016,0.392399803307351,1.74025550326595));
#21796=CARTESIAN_POINT('Ctrl Pts',(91.8409076018317,0.579477199565824,1.67935814700008));
#21797=CARTESIAN_POINT('Ctrl Pts',(91.8388853173912,0.608885385620271,1.66892061177424));
#21798=CARTESIAN_POINT('Ctrl Pts',(91.8358102077816,0.652613531539066,1.65209102623873));
#21799=CARTESIAN_POINT('Ctrl Pts',(91.8347764777623,0.667149585711418,1.64627475975517));
#21800=CARTESIAN_POINT('Ctrl Pts',(91.832891401069,0.693348504046896,1.63538790435042));
#21801=CARTESIAN_POINT('Ctrl Pts',(91.832042317579,0.705037526903719,1.63038272100396));
#21802=CARTESIAN_POINT('Ctrl Pts',(91.8301960411874,0.730207281430418,1.619283863412));
#21803=CARTESIAN_POINT('Ctrl Pts',(91.8291973974487,0.743667551081964,1.613146445466));
#21804=CARTESIAN_POINT('Ctrl Pts',(91.826423053717,0.780628225664122,1.59573275162663));
#21805=CARTESIAN_POINT('Ctrl Pts',(91.8246354112315,0.803958669644917,1.58410661673838));
#21806=CARTESIAN_POINT('Ctrl Pts',(91.8137524017066,0.943027524988194,1.51094165873883));
#21807=CARTESIAN_POINT('Ctrl Pts',(91.804224378576,1.0518998242969,1.43726843307516));
#21808=CARTESIAN_POINT('Ctrl Pts',(91.7898960501897,1.20105764586991,1.3102421806304));
#21809=CARTESIAN_POINT('Ctrl Pts',(91.7851561968135,1.24811641309629,1.26549608234068));
#21810=CARTESIAN_POINT('Ctrl Pts',(91.778006391002,1.31668748356836,1.19274018908559));
#21811=CARTESIAN_POINT('Ctrl Pts',(91.7755281503241,1.33999198730462,1.16649772817379));
#21812=CARTESIAN_POINT('Ctrl Pts',(91.7723084586074,1.36982345088723,1.13083061637614));
#21813=CARTESIAN_POINT('Ctrl Pts',(91.7715238242253,1.37705722589921,1.12201050948417));
#21814=CARTESIAN_POINT('Ctrl Pts',(91.7702332267552,1.38890327164627,1.10727952854062));
#21815=CARTESIAN_POINT('Ctrl Pts',(91.7697239675693,1.39356389600405,1.10140815653529));
#21816=CARTESIAN_POINT('Ctrl Pts',(91.7687576556362,1.40238357045093,1.09015167489518));
#21817=CARTESIAN_POINT('Ctrl Pts',(91.7683001229671,1.40654906076195,1.08477190992296));
#21818=CARTESIAN_POINT('Ctrl Pts',(91.767063260686,1.41777743064768,1.07009695738435));
#21819=CARTESIAN_POINT('Ctrl Pts',(91.7662880246245,1.42477990221484,1.06075566907453));
#21820=CARTESIAN_POINT('Ctrl Pts',(91.7632450834048,1.45209833828793,1.02355426970084));
#21821=CARTESIAN_POINT('Ctrl Pts',(91.7610207790669,1.4716947200969,0.995172317384239));
#21822=CARTESIAN_POINT('Ctrl Pts',(91.7523107378704,1.54623815049912,0.880186363919749));
#21823=CARTESIAN_POINT('Ctrl Pts',(91.7460874019661,1.59447016362826,0.789461020201902));
#21824=CARTESIAN_POINT('Ctrl Pts',(91.7388340402168,1.6406200505518,0.680930342919028));
#21825=CARTESIAN_POINT('Ctrl Pts',(91.7378874286032,1.64645047773804,0.666709156673473));
#21826=CARTESIAN_POINT('Ctrl Pts',(91.73202836253,1.68130427070451,0.578449586914254));
#21827=CARTESIAN_POINT('Ctrl Pts',(91.7270568303196,1.7055100168224,0.502614665240375));
#21828=CARTESIAN_POINT('Ctrl Pts',(91.7202765414743,1.73066470906533,0.400643118378392));
#21829=CARTESIAN_POINT('Ctrl Pts',(91.7186138959088,1.73624154998054,0.375739825724619));
#21830=CARTESIAN_POINT('Ctrl Pts',(91.7159777971819,1.74414879221804,0.336482057373719));
#21831=CARTESIAN_POINT('Ctrl Pts',(91.7150159437258,1.7468428323552,0.322203789946394));
#21832=CARTESIAN_POINT('Ctrl Pts',(91.7132001822935,1.75156970911691,0.295347131620639));
#21833=CARTESIAN_POINT('Ctrl Pts',(91.7123476225591,1.75364297393904,0.282776730647458));
#21834=CARTESIAN_POINT('Ctrl Pts',(91.7104134190957,1.75801711107587,0.254354945609482));
#21835=CARTESIAN_POINT('Ctrl Pts',(91.7093293507303,1.76023912703704,0.238492740923997));
#21836=CARTESIAN_POINT('Ctrl Pts',(91.7059806226956,1.76640065437399,0.189714765287039));
#21837=CARTESIAN_POINT('Ctrl Pts',(91.7036941703071,1.76963328852576,0.156718640754545));
#21838=CARTESIAN_POINT('Ctrl Pts',(91.697390069832,1.77592041452695,0.0666246359638738));
#21839=CARTESIAN_POINT('Ctrl Pts',(91.693324754067,1.77714075608374,0.0094926279344601));
#21840=CARTESIAN_POINT('Ctrl Pts',(91.6892085959652,1.77561363837197,-0.0475422940912359));
#21841=CARTESIAN_POINT('Ctrl Pts',(91.5422141974348,1.77561363837091,-0.0475422941309033));
#21842=CARTESIAN_POINT('Ctrl Pts',(91.5425519318852,1.77574653122244,-0.0425790006270345));
#21843=CARTESIAN_POINT('Ctrl Pts',(91.5428885299719,1.77585861629585,-0.0376150490231579));
#21844=CARTESIAN_POINT('Ctrl Pts',(91.5436822177452,1.7760745899505,-0.0258676734239604));
#21845=CARTESIAN_POINT('Ctrl Pts',(91.5441382891879,1.7761604350442,-0.0190839848731418));
#21846=CARTESIAN_POINT('Ctrl Pts',(91.5453824660129,1.77628917985943,-0.000492058207452863));
#21847=CARTESIAN_POINT('Ctrl Pts',(91.5461663296664,1.77625320414425,0.0113166306758942));
#21848=CARTESIAN_POINT('Ctrl Pts',(91.5493297410634,1.7756282768274,0.0593148228646064));
#21849=CARTESIAN_POINT('Ctrl Pts',(91.5516611592437,1.77405101696591,0.0954852307471094));
#21850=CARTESIAN_POINT('Ctrl Pts',(91.5629724388346,1.76084423229778,0.273272296370204));
#21851=CARTESIAN_POINT('Ctrl Pts',(91.5714485930022,1.73335746888836,0.413192838573033));
#21852=CARTESIAN_POINT('Ctrl Pts',(91.5843105432977,1.66973662378181,0.609210664155319));
#21853=CARTESIAN_POINT('Ctrl Pts',(91.588366794124,1.64671191933351,0.668951830668713));
#21854=CARTESIAN_POINT('Ctrl Pts',(91.5938323575766,1.61231893159721,0.745582024222819));
#21855=CARTESIAN_POINT('Ctrl Pts',(91.5951449262976,1.60381315424725,0.763706884215499));
#21856=CARTESIAN_POINT('Ctrl Pts',(91.5973467248221,1.58915207158709,0.793622408729495));
#21857=CARTESIAN_POINT('Ctrl Pts',(91.5982299959621,1.58316730546669,0.805494941522774));
#21858=CARTESIAN_POINT('Ctrl Pts',(91.599975952941,1.5711391266092,0.828704368234416));
#21859=CARTESIAN_POINT('Ctrl Pts',(91.6008382737704,1.56510487981056,0.840045109048163));
#21860=CARTESIAN_POINT('Ctrl Pts',(91.6027493051344,1.55153018224219,0.864903297216508));
#21861=CARTESIAN_POINT('Ctrl Pts',(91.6037999213665,1.54393505300273,0.878389518116582));
#21862=CARTESIAN_POINT('Ctrl Pts',(91.607461713061,1.51701486077285,0.924762068604568));
#21863=CARTESIAN_POINT('Ctrl Pts',(91.6101042527252,1.4968086475851,0.957121966447943));
#21864=CARTESIAN_POINT('Ctrl Pts',(91.621869423726,1.40351796854557,1.09633823509033));
#21865=CARTESIAN_POINT('Ctrl Pts',(91.6313641976844,1.31992734195272,1.19565996791369));
#21866=CARTESIAN_POINT('Ctrl Pts',(91.6459922333852,1.17495045547046,1.33401467858381));
#21867=CARTESIAN_POINT('Ctrl Pts',(91.6511376289472,1.1206960358983,1.37990799055999));
#21868=CARTESIAN_POINT('Ctrl Pts',(91.6573484360426,1.04972712866114,1.43298548217403));
#21869=CARTESIAN_POINT('Ctrl Pts',(91.6585722199366,1.0354620742978,1.44332698588431));
#21870=CARTESIAN_POINT('Ctrl Pts',(91.6603837958991,1.01388802678376,1.45848264611069));
#21871=CARTESIAN_POINT('Ctrl Pts',(91.6609814873964,1.00669396768641,1.46345748945314));
#21872=CARTESIAN_POINT('Ctrl Pts',(91.6620098489672,0.994178730341113,1.47197607964926));
#21873=CARTESIAN_POINT('Ctrl Pts',(91.6624421264867,0.988874878167424,1.47554444380408));
#21874=CARTESIAN_POINT('Ctrl Pts',(91.6634597697117,0.976287135375212,1.48391495698939));
#21875=CARTESIAN_POINT('Ctrl Pts',(91.6640434879078,0.968986993958848,1.48869217228892));
#21876=CARTESIAN_POINT('Ctrl Pts',(91.6657881620775,0.946938087578518,1.50289007578937));
#21877=CARTESIAN_POINT('Ctrl Pts',(91.6669390394554,0.932084515807071,1.51214709390441));
#21878=CARTESIAN_POINT('Ctrl Pts',(91.6768023363388,0.802366118897334,1.59035212828615));
#21879=CARTESIAN_POINT('Ctrl Pts',(91.6848606573189,0.680163382060995,1.64632902600288));
#21880=CARTESIAN_POINT('Ctrl Pts',(91.6984505274092,0.470514268804361,1.71498685779538));
#21881=CARTESIAN_POINT('Ctrl Pts',(91.7038436646326,0.38636335416173,1.73588147781375));
#21882=CARTESIAN_POINT('Ctrl Pts',(91.7111116468031,0.275327105440494,1.75497556409935));
#21883=CARTESIAN_POINT('Ctrl Pts',(91.7128099411117,0.249530971905259,1.75882870848304));
#21884=CARTESIAN_POINT('Ctrl Pts',(91.7154837934504,0.209220516165679,1.7639452110253));
#21885=CARTESIAN_POINT('Ctrl Pts',(91.7164470185801,0.19475902641779,1.76560041694032));
#21886=CARTESIAN_POINT('Ctrl Pts',(91.7182541990949,0.167749602095877,1.76835594772748));
#21887=CARTESIAN_POINT('Ctrl Pts',(91.7190966907885,0.155207068665014,1.76950090098788));
#21888=CARTESIAN_POINT('Ctrl Pts',(91.720992880387,0.127094315643159,1.77176600128456));
#21889=CARTESIAN_POINT('Ctrl Pts',(91.7220487633459,0.111519538705679,1.77281445551605));
#21890=CARTESIAN_POINT('Ctrl Pts',(91.7247781308554,0.0714756030363633,
1.77498034750434));
#21891=CARTESIAN_POINT('Ctrl Pts',(91.7264607959453,0.0469941918793711,
1.77579712742451));
#21892=CARTESIAN_POINT('Ctrl Pts',(91.7360700870387,-0.0916038404876299,
1.77755327864952));
#21893=CARTESIAN_POINT('Ctrl Pts',(91.7443155224906,-0.205567735304695,
1.7679990859125));
#21894=CARTESIAN_POINT('Ctrl Pts',(91.7582349886872,-0.392935650278824,
1.7339251046491));
#21895=CARTESIAN_POINT('Ctrl Pts',(91.7638366925282,-0.467105698121408,
1.71543227170823));
#21896=CARTESIAN_POINT('Ctrl Pts',(91.7711811368466,-0.564680806581021,
1.68430357844077));
#21897=CARTESIAN_POINT('Ctrl Pts',(91.7730336688769,-0.589327924888796,
1.67583880403174));
#21898=CARTESIAN_POINT('Ctrl Pts',(91.7761857451629,-0.631455511862717,
1.66032609492333));
#21899=CARTESIAN_POINT('Ctrl Pts',(91.7774960292812,-0.649026185341669,
1.6535367811025));
#21900=CARTESIAN_POINT('Ctrl Pts',(91.7794088922743,-0.67480995125309,1.64309957896986));
#21901=CARTESIAN_POINT('Ctrl Pts',(91.7800229854057,-0.683108070206707,
1.63966706069126));
#21902=CARTESIAN_POINT('Ctrl Pts',(91.781115959176,-0.697920583288976,1.63340789127914));
#21903=CARTESIAN_POINT('Ctrl Pts',(91.7815961760271,-0.704444442446769,
1.63060495283948));
#21904=CARTESIAN_POINT('Ctrl Pts',(91.7826701311017,-0.71906945257132,1.62421724340548));
#21905=CARTESIAN_POINT('Ctrl Pts',(91.7832625674971,-0.727160784982456,
1.62061091337473));
#21906=CARTESIAN_POINT('Ctrl Pts',(91.7850614349111,-0.751787841983871,
1.60941298249954));
#21907=CARTESIAN_POINT('Ctrl Pts',(91.7862568425081,-0.768234770260599,
1.60162745620269));
#21908=CARTESIAN_POINT('Ctrl Pts',(91.7928718788215,-0.85948670054037,1.55670209981919));
#21909=CARTESIAN_POINT('Ctrl Pts',(91.7980455689796,-0.931727763273796,
1.51457104335979));
#21910=CARTESIAN_POINT('Ctrl Pts',(91.8090871906988,-1.08002453651872,1.41344251073098));
#21911=CARTESIAN_POINT('Ctrl Pts',(91.8149303404641,-1.15479137072698,1.35304422457224));
#21912=CARTESIAN_POINT('Ctrl Pts',(91.8232407852767,-1.25062076575433,1.26187570758489));
#21913=CARTESIAN_POINT('Ctrl Pts',(91.8255455094886,-1.27615377857022,1.23604768741076));
#21914=CARTESIAN_POINT('Ctrl Pts',(91.8296955439495,-1.32007299345992,1.18880873207118));
#21915=CARTESIAN_POINT('Ctrl Pts',(91.8315277288333,-1.3387745237276,1.16770781532602));
#21916=CARTESIAN_POINT('Ctrl Pts',(91.8343652962756,-1.36663234318274,1.13472663854121));
#21917=CARTESIAN_POINT('Ctrl Pts',(91.835355689996,-1.37615405910815,1.12316004567167));
#21918=CARTESIAN_POINT('Ctrl Pts',(91.8371056542482,-1.39261866699155,1.1026358025135));
#21919=CARTESIAN_POINT('Ctrl Pts',(91.8378626406892,-1.39962435619276,1.09372945280813));
#21920=CARTESIAN_POINT('Ctrl Pts',(91.8396026069154,-1.41545847003973,1.07319823325502));
#21921=CARTESIAN_POINT('Ctrl Pts',(91.8405877751235,-1.42422966928899,1.06153047774835));
#21922=CARTESIAN_POINT('Ctrl Pts',(91.8433141545825,-1.44796558775933,1.02913233786918));
#21923=CARTESIAN_POINT('Ctrl Pts',(91.8450667949396,-1.46262756000237,1.00818560506822));
#21924=CARTESIAN_POINT('Ctrl Pts',(91.8561829171046,-1.55186571776381,0.874650648695101));
#21925=CARTESIAN_POINT('Ctrl Pts',(91.8660105609902,-1.61383773358196,0.754198806567161));
#21926=CARTESIAN_POINT('Ctrl Pts',(91.8804739315429,-1.68375778544943,0.569180732782464));
#21927=CARTESIAN_POINT('Ctrl Pts',(91.8850566363689,-1.70282642520583,0.509303449289825));
#21928=CARTESIAN_POINT('Ctrl Pts',(91.8919989415696,-1.72735703059993,0.415308602374065));
#21929=CARTESIAN_POINT('Ctrl Pts',(91.8944232036531,-1.7350645956287,0.381830802954414));
#21930=CARTESIAN_POINT('Ctrl Pts',(91.8975800912173,-1.74400306373291,0.337111335901463));
#21931=CARTESIAN_POINT('Ctrl Pts',(91.8983541432809,-1.74610419988145,0.326053490808516));
#21932=CARTESIAN_POINT('Ctrl Pts',(91.8996286390645,-1.74941483822113,0.307679626733279));
#21933=CARTESIAN_POINT('Ctrl Pts',(91.9001322838279,-1.75068386999912,0.300374804640621));
#21934=CARTESIAN_POINT('Ctrl Pts',(91.9011520465193,-1.75317380398139,0.285490128164897));
#21935=CARTESIAN_POINT('Ctrl Pts',(91.9016679795735,-1.75439136861259,0.277909934368844));
#21936=CARTESIAN_POINT('Ctrl Pts',(91.9030162476974,-1.75746042734692,0.257978452724952));
#21937=CARTESIAN_POINT('Ctrl Pts',(91.9038441972181,-1.75923091042241,0.245614864237416));
#21938=CARTESIAN_POINT('Ctrl Pts',(91.9075057845089,-1.76653874757136,0.190441939138185));
#21939=CARTESIAN_POINT('Ctrl Pts',(91.9102700285676,-1.77064540358375,0.147454389309093));
#21940=CARTESIAN_POINT('Ctrl Pts',(91.9190531877026,-1.77883314519859,0.00833144120753962));
#21941=CARTESIAN_POINT('Ctrl Pts',(91.924891945633,-1.7766752984376,-0.0879991154976709));
#21942=CARTESIAN_POINT('Ctrl Pts',(91.9363074492755,-1.75749720032711,-0.27245798831861));
#21943=CARTESIAN_POINT('Ctrl Pts',(91.9418567939805,-1.74159120012447,-0.360398758734652));
#21944=CARTESIAN_POINT('Ctrl Pts',(91.9493150138125,-1.712498448419,-0.472347009752864));
#21945=CARTESIAN_POINT('Ctrl Pts',(91.951035518596,-1.70528076420434,-0.497775080151869));
#21946=CARTESIAN_POINT('Ctrl Pts',(91.9537365372346,-1.69319176047877,-0.537009932927673));
#21947=CARTESIAN_POINT('Ctrl Pts',(91.9547042931065,-1.68871239387534,-0.550934147674725));
#21948=CARTESIAN_POINT('Ctrl Pts',(91.9565155219082,-1.68005889553645,-0.576736194935529));
#21949=CARTESIAN_POINT('Ctrl Pts',(91.9573574721371,-1.67592943177664,-0.588628114043661));
#21950=CARTESIAN_POINT('Ctrl Pts',(91.9592466105132,-1.66642890397615,-0.615076823189348));
#21951=CARTESIAN_POINT('Ctrl Pts',(91.9602959108043,-1.66099285731871,-0.629608999047637));
#21952=CARTESIAN_POINT('Ctrl Pts',(91.962996250949,-1.64660315834898,-0.666593056353544));
#21953=CARTESIAN_POINT('Ctrl Pts',(91.9646561435933,-1.63738057228142,-0.688936154787929));
#21954=CARTESIAN_POINT('Ctrl Pts',(91.9749417825677,-1.57795956540621,-0.824953840683884));
#21955=CARTESIAN_POINT('Ctrl Pts',(91.9839533423938,-1.51641022468229,-0.933271170475915));
#21956=CARTESIAN_POINT('Ctrl Pts',(91.9981093751224,-1.40370587949371,-1.09063357379551));
#21957=CARTESIAN_POINT('Ctrl Pts',(92.0031834121047,-1.36006431738604,-1.14459502019992));
#21958=CARTESIAN_POINT('Ctrl Pts',(92.0107548787148,-1.28886123290988,-1.2227946855183));
#21959=CARTESIAN_POINT('Ctrl Pts',(92.0133294203464,-1.26352033314355,-1.24896233599829));
#21960=CARTESIAN_POINT('Ctrl Pts',(92.0166473109977,-1.22915310485126,-1.28233324486217));
#21961=CARTESIAN_POINT('Ctrl Pts',(92.0174373557782,-1.22083770706403,-1.29025238485724));
#21962=CARTESIAN_POINT('Ctrl Pts',(92.0187309907237,-1.2069935217153,-1.30318316555679));
#21963=CARTESIAN_POINT('Ctrl Pts',(92.0192379727642,-1.20150902865715,-1.30824148573596));
#21964=CARTESIAN_POINT('Ctrl Pts',(92.0202571770162,-1.19036055803366,-1.31839441494967));
#21965=CARTESIAN_POINT('Ctrl Pts',(92.0207692855079,-1.18469538008056,-1.32348742095573));
#21966=CARTESIAN_POINT('Ctrl Pts',(92.0220957296958,-1.16986143648105,-1.33665159378802));
#21967=CARTESIAN_POINT('Ctrl Pts',(92.0229059355096,-1.16064169083018,-1.34466506977725));
#21968=CARTESIAN_POINT('Ctrl Pts',(92.0263493872838,-1.12081272729846,-1.3785681014705));
#21969=CARTESIAN_POINT('Ctrl Pts',(92.0289231063123,-1.08941216027471,-1.40351447086431));
#21970=CARTESIAN_POINT('Ctrl Pts',(92.0376764168079,-0.978115845369659,
-1.48594636884029));
#21971=CARTESIAN_POINT('Ctrl Pts',(92.0436487359532,-0.894304958489487,
-1.53784538128026));
#21972=CARTESIAN_POINT('Ctrl Pts',(92.0552677409654,-0.726079608906529,
-1.62359010624519));
#21973=CARTESIAN_POINT('Ctrl Pts',(92.0608847387086,-0.642529731144645,
-1.65842977746595));
#21974=CARTESIAN_POINT('Ctrl Pts',(92.0684253573349,-0.531456170209446,
-1.69508846539179));
#21975=CARTESIAN_POINT('Ctrl Pts',(92.0701553536954,-0.506032545487175,
-1.70285099438323));
#21976=CARTESIAN_POINT('Ctrl Pts',(92.0728680004031,-0.46633431263439,-1.71400443727344));
#21977=CARTESIAN_POINT('Ctrl Pts',(92.0738377098263,-0.452175098528091,
-1.71779409731215));
#21978=CARTESIAN_POINT('Ctrl Pts',(92.0756507426971,-0.425772961978432,
-1.72451148735308));
#21979=CARTESIAN_POINT('Ctrl Pts',(92.0764925185536,-0.413542605697971,
-1.72748516183582));
#21980=CARTESIAN_POINT('Ctrl Pts',(92.0783788574649,-0.386204729737495,
-1.73382511161694));
#21981=CARTESIAN_POINT('Ctrl Pts',(92.0794255028663,-0.371082889453845,
-1.73712436906814));
#21982=CARTESIAN_POINT('Ctrl Pts',(92.0825036208095,-0.326759572922621,
-1.74618961199936));
#21983=CARTESIAN_POINT('Ctrl Pts',(92.0845518293549,-0.297455208408674,
-1.7514194793164));
#21984=CARTESIAN_POINT('Ctrl Pts',(92.0962935114343,-0.130610694939501,
-1.77688782294627));
#21985=CARTESIAN_POINT('Ctrl Pts',(92.1064653124034,0.00878068179485438,
-1.7816563613688));
#21986=CARTESIAN_POINT('Ctrl Pts',(92.1220276840634,0.221114897287929,-1.76399061123504));
#21987=CARTESIAN_POINT('Ctrl Pts',(92.1274070239509,0.294508989966902,-1.75323164953646));
#21988=CARTESIAN_POINT('Ctrl Pts',(92.1338625866123,0.384588060156227,-1.73420829242975));
#21989=CARTESIAN_POINT('Ctrl Pts',(92.1351102108654,0.402097367072228,-1.73023239677276));
#21990=CARTESIAN_POINT('Ctrl Pts',(92.1369498025625,0.428106734187949,-1.72391018780301));
#21991=CARTESIAN_POINT('Ctrl Pts',(92.1375521031531,0.436653894719554,-1.72176511058206));
#21992=CARTESIAN_POINT('Ctrl Pts',(92.1385853088255,0.451376416154418,-1.71795352001386));
#21993=CARTESIAN_POINT('Ctrl Pts',(92.1390178730658,0.457559112104252,-1.71631717014676));
#21994=CARTESIAN_POINT('Ctrl Pts',(92.1400317631408,0.472095266265816,-1.71238580977867));
#21995=CARTESIAN_POINT('Ctrl Pts',(92.1406114929616,0.480440933777247,-1.71006304532222));
#21996=CARTESIAN_POINT('Ctrl Pts',(92.1423317172581,0.505293853975976,-1.70294967837966));
#21997=CARTESIAN_POINT('Ctrl Pts',(92.1434625455105,0.521749452693285,-1.69798028504208));
#21998=CARTESIAN_POINT('Ctrl Pts',(92.1517290200104,0.642661868524556,-1.65954232393089));
#21999=CARTESIAN_POINT('Ctrl Pts',(92.1584242322625,0.743904502015605,-1.61669649032372));
#22000=CARTESIAN_POINT('Ctrl Pts',(92.1714619427221,0.93101957165145,-1.5161831720467));
#22001=CARTESIAN_POINT('Ctrl Pts',(92.1777779170461,1.01708857960022,-1.45984136232376));
#22002=CARTESIAN_POINT('Ctrl Pts',(92.1863682453358,1.12242973853387,-1.37702459188812));
#22003=CARTESIAN_POINT('Ctrl Pts',(92.1883982760072,1.14653699270516,-1.35701804606764));
#22004=CARTESIAN_POINT('Ctrl Pts',(92.1914766676314,1.18182770762601,-1.32611848874536));
#22005=CARTESIAN_POINT('Ctrl Pts',(92.1925056786124,1.19341785785592,-1.31569782526542));
#22006=CARTESIAN_POINT('Ctrl Pts',(92.1943777408234,1.21412170667499,-1.29658440464684));
#22007=CARTESIAN_POINT('Ctrl Pts',(92.1952185068084,1.22328302614618,-1.28794458766101));
#22008=CARTESIAN_POINT('Ctrl Pts',(92.1970414024861,1.24284646691842,-1.26909774612404));
#22009=CARTESIAN_POINT('Ctrl Pts',(92.1980248960732,1.25321632151024,-1.25885871286726));
#22010=CARTESIAN_POINT('Ctrl Pts',(92.2007419485579,1.28135119760027,-1.23038659398809));
#22011=CARTESIAN_POINT('Ctrl Pts',(92.2024868085714,1.29885147415598,-1.21189801271387));
#22012=CARTESIAN_POINT('Ctrl Pts',(92.2136603939448,1.4072993783695,-1.09227780103013));
#22013=CARTESIAN_POINT('Ctrl Pts',(92.2235610967633,1.48676021584207,-0.981373136811511));
#22014=CARTESIAN_POINT('Ctrl Pts',(92.2380544706016,1.58300710073718,-0.808101152675607));
#22015=CARTESIAN_POINT('Ctrl Pts',(92.2425963608807,1.61035424642723,-0.752129641879309));
#22016=CARTESIAN_POINT('Ctrl Pts',(92.2494858157535,1.64807151500799,-0.663393921046877));
#22017=CARTESIAN_POINT('Ctrl Pts',(92.251897030935,1.66052685562834,-0.631571164964032));
#22018=CARTESIAN_POINT('Ctrl Pts',(92.2550398795592,1.67584856121881,-0.588830943434232));
#22019=CARTESIAN_POINT('Ctrl Pts',(92.2558124950465,1.67953947155165,-0.578219214579228));
#22020=CARTESIAN_POINT('Ctrl Pts',(92.2570852778343,1.68549726151928,-0.560551469105874));
#22021=CARTESIAN_POINT('Ctrl Pts',(92.2575886290755,1.68782107173756,-0.553515135286951));
#22022=CARTESIAN_POINT('Ctrl Pts',(92.2586084750066,1.69246448612714,-0.539154014804802));
#22023=CARTESIAN_POINT('Ctrl Pts',(92.259124778183,1.69478071803537,-0.531828366962221));
#22024=CARTESIAN_POINT('Ctrl Pts',(92.2604751386562,1.70074485226118,-0.51253062267433));
#22025=CARTESIAN_POINT('Ctrl Pts',(92.2613047857374,1.70431395985522,-0.500534354468809));
#22026=CARTESIAN_POINT('Ctrl Pts',(92.2649878024943,1.71971057940575,-0.446709134278103));
#22027=CARTESIAN_POINT('Ctrl Pts',(92.2677707691593,1.73012804537282,-0.404488751248554));
#22028=CARTESIAN_POINT('Ctrl Pts',(92.276556990232,1.75854201205792,-0.267964616486354));
#22029=CARTESIAN_POINT('Ctrl Pts',(92.2823826576816,1.77045114333896,-0.172568675480497));
#22030=CARTESIAN_POINT('Ctrl Pts',(92.2888893700168,1.77501388171394,-0.0669643044145619));
#22031=CARTESIAN_POINT('Ctrl Pts',(92.2894881254696,1.77535361373816,-0.0572537193054558));
#22032=CARTESIAN_POINT('Ctrl Pts',(92.2900876926257,1.77561363877829,-0.0475422789160742));
#22033=CARTESIAN_POINT('Origin',(88.3562164250559,0.,0.));
#22034=CARTESIAN_POINT('',(93.1870734163657,1.77561363809323,-0.0475423045015944));
#22035=CARTESIAN_POINT('',(93.0389806716583,1.77561363838114,-0.0475422937485569));
#22036=CARTESIAN_POINT('',(88.3562164250559,1.77561363837197,-0.0475422940912398));
#22037=CARTESIAN_POINT('Ctrl Pts',(93.1870734170205,1.77561363809212,-0.0475423045429159));
#22038=CARTESIAN_POINT('Ctrl Pts',(93.1843673805862,1.77446631716615,-0.0903925345226306));
#22039=CARTESIAN_POINT('Ctrl Pts',(93.1817066455266,1.77176788935747,-0.133200198010226));
#22040=CARTESIAN_POINT('Ctrl Pts',(93.1704258635094,1.7536542695672,-0.315233559152988));
#22041=CARTESIAN_POINT('Ctrl Pts',(93.1619621166615,1.72335900659772,-0.452444856457427));
#22042=CARTESIAN_POINT('Ctrl Pts',(93.1512695216931,1.66858663503551,-0.609572023947492));
#22043=CARTESIAN_POINT('Ctrl Pts',(93.1495592451614,1.65935381954731,-0.634274544278217));
#22044=CARTESIAN_POINT('Ctrl Pts',(93.1467672866258,1.64355573744733,-0.673833813572958));
#22045=CARTESIAN_POINT('Ctrl Pts',(93.145696890934,1.63733041970008,-0.688822573714308));
#22046=CARTESIAN_POINT('Ctrl Pts',(93.1437724891179,1.625845524013,-0.715439170253147));
#22047=CARTESIAN_POINT('Ctrl Pts',(93.1429211990053,1.62066431823258,-0.727099736830207));
#22048=CARTESIAN_POINT('Ctrl Pts',(93.1411003149421,1.6093718737776,-0.751793471311541));
#22049=CARTESIAN_POINT('Ctrl Pts',(93.1401296066326,1.60322696207297,-0.764810132269781));
#22050=CARTESIAN_POINT('Ctrl Pts',(93.1374671879178,1.58603888844342,-0.800101738619688));
#22051=CARTESIAN_POINT('Ctrl Pts',(93.1357648103294,1.57468553774726,-0.822221074750268));
#22052=CARTESIAN_POINT('Ctrl Pts',(93.1264507071165,1.51064967405584,-0.940785928120775));
#22053=CARTESIAN_POINT('Ctrl Pts',(93.1185425967317,1.44957549047646,-1.03240689354177));
#22054=CARTESIAN_POINT('Ctrl Pts',(93.1022224701107,1.30890587238961,-1.20613088569067));
#22055=CARTESIAN_POINT('Ctrl Pts',(93.0938417551999,1.22904976357941,-1.28741087716945));
#22056=CARTESIAN_POINT('Ctrl Pts',(93.0847061384313,1.12910405227286,-1.37130235895337));
#22057=CARTESIAN_POINT('Ctrl Pts',(93.0835403350365,1.11608728938702,-1.38191726748776));
#22058=CARTESIAN_POINT('Ctrl Pts',(93.0817860293388,1.09606923888548,-1.39777419428674));
#22059=CARTESIAN_POINT('Ctrl Pts',(93.0811888070299,1.08917696967992,-1.40315145708248));
#22060=CARTESIAN_POINT('Ctrl Pts',(93.0801562750995,1.07712076060961,-1.41241519811146));
#22061=CARTESIAN_POINT('Ctrl Pts',(93.0797194060113,1.07197505125258,-1.41632458053809));
#22062=CARTESIAN_POINT('Ctrl Pts',(93.0786838944363,1.05967204171987,-1.42556616033597));
#22063=CARTESIAN_POINT('Ctrl Pts',(93.0780870217076,1.05249575016018,-1.43087260717026));
#22064=CARTESIAN_POINT('Ctrl Pts',(93.0762789259939,1.03050921498149,-1.44687544680128));
#22065=CARTESIAN_POINT('Ctrl Pts',(93.0750787889028,1.01557317178617,-1.45739802294471));
#22066=CARTESIAN_POINT('Ctrl Pts',(93.0689209533595,0.937328876468771,-1.51073466917814));
#22067=CARTESIAN_POINT('Ctrl Pts',(93.0641668884786,0.87146133019501,-1.54966526005496));
#22068=CARTESIAN_POINT('Ctrl Pts',(93.0504766827301,0.673310650565444,-1.65013727612473));
#22069=CARTESIAN_POINT('Ctrl Pts',(93.0416621358394,0.535735953823592,-1.69978921579432));
#22070=CARTESIAN_POINT('Ctrl Pts',(93.0306563655123,0.369707433424003,-1.73752212495236));
#22071=CARTESIAN_POINT('Ctrl Pts',(93.0290552666102,0.345659566130191,-1.74246552034583));
#22072=CARTESIAN_POINT('Ctrl Pts',(93.0264946158224,0.307425470731535,-1.74950249106907));
#22073=CARTESIAN_POINT('Ctrl Pts',(93.0255455505255,0.293302534992512,-1.75192550897179));
#22074=CARTESIAN_POINT('Ctrl Pts',(93.0237402903007,0.266539947072141,-1.75618439111149));
#22075=CARTESIAN_POINT('Ctrl Pts',(93.0228852694801,0.253906737887011,-1.75805532128426));
#22076=CARTESIAN_POINT('Ctrl Pts',(93.0209264008257,0.225067367983645,-1.76200899482881));
#22077=CARTESIAN_POINT('Ctrl Pts',(93.0198198758359,0.20885064657166,-1.76400464688679));
#22078=CARTESIAN_POINT('Ctrl Pts',(93.0163238802699,0.157862238576624,-1.76956641309156));
#22079=CARTESIAN_POINT('Ctrl Pts',(93.0139097300579,0.123013307105346,-1.77232988018401));
#22080=CARTESIAN_POINT('Ctrl Pts',(92.9999928010988,-0.0757404713423424,
-1.78220084245671));
#22081=CARTESIAN_POINT('Ctrl Pts',(92.9878210116381,-0.239911681590536,
-1.76759747852855));
#22082=CARTESIAN_POINT('Ctrl Pts',(92.9723562543569,-0.448349156027029,
-1.71945921412546));
#22083=CARTESIAN_POINT('Ctrl Pts',(92.9687914126519,-0.496507019657609,
-1.70617662834811));
#22084=CARTESIAN_POINT('Ctrl Pts',(92.9644079428029,-0.556535988513159,
-1.6868621532881));
#22085=CARTESIAN_POINT('Ctrl Pts',(92.9635024540357,-0.568982205374252,
-1.68270481853185));
#22086=CARTESIAN_POINT('Ctrl Pts',(92.962066432522,-0.588812232377587,-1.67583592741605));
#22087=CARTESIAN_POINT('Ctrl Pts',(92.9615310675691,-0.596225809967661,
-1.67321268528922));
#22088=CARTESIAN_POINT('Ctrl Pts',(92.9604961718943,-0.610601856938426,
-1.66801814004576));
#22089=CARTESIAN_POINT('Ctrl Pts',(92.9599963686371,-0.617565990660018,
-1.66545230879401));
#22090=CARTESIAN_POINT('Ctrl Pts',(92.9587600187878,-0.634839669341869,
-1.6589648328293));
#22091=CARTESIAN_POINT('Ctrl Pts',(92.9580265155479,-0.645129381522193,
-1.65499057970824));
#22092=CARTESIAN_POINT('Ctrl Pts',(92.9551928964557,-0.685007733688089,
-1.63915968916185));
#22093=CARTESIAN_POINT('Ctrl Pts',(92.9531301053352,-0.714313984906699,
-1.62660256639049));
#22094=CARTESIAN_POINT('Ctrl Pts',(92.9475576639566,-0.793656333575301,
-1.59004765945956));
#22095=CARTESIAN_POINT('Ctrl Pts',(92.9441100354529,-0.842932531552592,
-1.56448314921777));
#22096=CARTESIAN_POINT('Ctrl Pts',(92.9319877639403,-1.01301471285963,-1.46587136257078));
#22097=CARTESIAN_POINT('Ctrl Pts',(92.9234582465617,-1.12621472543064,-1.38080230647322));
#22098=CARTESIAN_POINT('Ctrl Pts',(92.9127366014071,-1.24662940472908,-1.26555645510259));
#22099=CARTESIAN_POINT('Ctrl Pts',(92.9110766451555,-1.26471925088722,-1.2474787071396));
#22100=CARTESIAN_POINT('Ctrl Pts',(92.9083503863304,-1.29348459470841,-1.21746365927781));
#22101=CARTESIAN_POINT('Ctrl Pts',(92.9072944936625,-1.30440038022468,-1.20576107855679));
#22102=CARTESIAN_POINT('Ctrl Pts',(92.9053858656151,-1.32371891678303,-1.18448072047841));
#22103=CARTESIAN_POINT('Ctrl Pts',(92.9045356672638,-1.33217965090295,-1.17495689751596));
#22104=CARTESIAN_POINT('Ctrl Pts',(92.9027058099775,-1.35007601430589,-1.15437005253446));
#22105=CARTESIAN_POINT('Ctrl Pts',(92.9017249119142,-1.35947965580081,-1.14328058941164));
#22106=CARTESIAN_POINT('Ctrl Pts',(92.899003764132,-1.3850389887192,-1.11237789948475));
#22107=CARTESIAN_POINT('Ctrl Pts',(92.897252038892,-1.40090415594431,-1.09233008688981));
#22108=CARTESIAN_POINT('Ctrl Pts',(92.8932809637014,-1.43554363353485,-1.04656204729599));
#22109=CARTESIAN_POINT('Ctrl Pts',(92.8910530477858,-1.45406971606169,-1.02066580627248));
#22110=CARTESIAN_POINT('Ctrl Pts',(92.8834946910346,-1.51390978920111,-0.932081786295268));
#22111=CARTESIAN_POINT('Ctrl Pts',(92.8780635928175,-1.55194097204341,-0.867281115467987));
#22112=CARTESIAN_POINT('Ctrl Pts',(92.8641441341732,-1.63786329875699,-0.697024873027511));
#22113=CARTESIAN_POINT('Ctrl Pts',(92.8556119688851,-1.67976500427924,-0.588925478803648));
#22114=CARTESIAN_POINT('Ctrl Pts',(92.8463537898442,-1.71532586980725,-0.461516056973144));
#22115=CARTESIAN_POINT('Ctrl Pts',(92.8452011798296,-1.71956642934384,-0.445456232595381));
#22116=CARTESIAN_POINT('Ctrl Pts',(92.8434626004822,-1.72568470341,-0.420894399555913));
#22117=CARTESIAN_POINT('Ctrl Pts',(92.84286813445,-1.72772609635524,-0.412434643526438));
#22118=CARTESIAN_POINT('Ctrl Pts',(92.8417939683239,-1.73132371965613,-0.397030078767995));
#22119=CARTESIAN_POINT('Ctrl Pts',(92.8413131744304,-1.73290045498333,-0.390090658967901));
#22120=CARTESIAN_POINT('Ctrl Pts',(92.840207557654,-1.73644787711398,-0.374031907282422));
#22121=CARTESIAN_POINT('Ctrl Pts',(92.839584425486,-1.73838847777447,-0.364906299787943));
#22122=CARTESIAN_POINT('Ctrl Pts',(92.8376070696733,-1.74435383594001,-0.335726249982958));
#22123=CARTESIAN_POINT('Ctrl Pts',(92.8362671627631,-1.74810430606625,-0.315616606699628));
#22124=CARTESIAN_POINT('Ctrl Pts',(92.833058508216,-1.75634162093474,-0.266782875578532));
#22125=CARTESIAN_POINT('Ctrl Pts',(92.8312050931124,-1.76047243829011,-0.238004143461919));
#22126=CARTESIAN_POINT('Ctrl Pts',(92.8234306336066,-1.77498732249631,-0.115582370821546));
#22127=CARTESIAN_POINT('Ctrl Pts',(92.8177068178969,-1.7786197400268,-0.0212896962673536));
#22128=CARTESIAN_POINT('Ctrl Pts',(92.8058156854698,-1.77069192889892,0.171843713879389));
#22129=CARTESIAN_POINT('Ctrl Pts',(92.7996581036799,-1.75835397810964,0.27031081915597));
#22130=CARTESIAN_POINT('Ctrl Pts',(92.7917713932719,-1.73319728442869,0.389362278079672));
#22131=CARTESIAN_POINT('Ctrl Pts',(92.7902928802,-1.7280981413152,0.411403146030047));
#22132=CARTESIAN_POINT('Ctrl Pts',(92.7878824979592,-1.71918224409287,0.44684494451532));
#22133=CARTESIAN_POINT('Ctrl Pts',(92.7869590411346,-1.71562621974485,0.460309296316371));
#22134=CARTESIAN_POINT('Ctrl Pts',(92.7851719168077,-1.70847872115155,0.486138118032187));
#22135=CARTESIAN_POINT('Ctrl Pts',(92.7843090518241,-1.70491039326013,0.498508120566227));
#22136=CARTESIAN_POINT('Ctrl Pts',(92.7822862601781,-1.69627516346444,0.527265423220525));
#22137=CARTESIAN_POINT('Ctrl Pts',(92.7811230124424,-1.69110480648257,0.543620045736141));
#22138=CARTESIAN_POINT('Ctrl Pts',(92.7772324613061,-1.67314329655655,0.59769732372607));
#22139=CARTESIAN_POINT('Ctrl Pts',(92.7744718236204,-1.65932104596304,0.635062052097813));
#22140=CARTESIAN_POINT('Ctrl Pts',(92.767559884455,-1.62211205029763,0.726115082455237));
#22141=CARTESIAN_POINT('Ctrl Pts',(92.7633678110767,-1.59730538737095,0.779169436418959));
#22142=CARTESIAN_POINT('Ctrl Pts',(92.750974053264,-1.51730275344643,0.93032908987476));
#22143=CARTESIAN_POINT('Ctrl Pts',(92.7426514302909,-1.45535271419137,1.02453310607392));
#22144=CARTESIAN_POINT('Ctrl Pts',(92.731876610334,-1.36126411094349,1.14168737692302));
#22145=CARTESIAN_POINT('Ctrl Pts',(92.7292022422055,-1.3366834333077,1.17037084376798));
#22146=CARTESIAN_POINT('Ctrl Pts',(92.7257470983207,-1.30307395845825,1.20714854199916));
#22147=CARTESIAN_POINT('Ctrl Pts',(92.7249169123541,-1.2948522360585,1.21596342486316));
#22148=CARTESIAN_POINT('Ctrl Pts',(92.7236232396188,-1.28179969613591,1.22967511643292));
#22149=CARTESIAN_POINT('Ctrl Pts',(92.7231554120005,-1.27702926548414,1.23462853205417));
#22150=CARTESIAN_POINT('Ctrl Pts',(92.722186917708,-1.26704604054714,1.24487492456682));
#22151=CARTESIAN_POINT('Ctrl Pts',(92.7216866732231,-1.26182862575356,1.25016309674087));
#22152=CARTESIAN_POINT('Ctrl Pts',(92.7204475024709,-1.24875676082029,1.26324703639823));
#22153=CARTESIAN_POINT('Ctrl Pts',(92.7197116506484,-1.24086217068869,1.27100260096203));
#22154=CARTESIAN_POINT('Ctrl Pts',(92.7168564198474,-1.20973659536803,1.30101359179794));
#22155=CARTESIAN_POINT('Ctrl Pts',(92.7147750960966,-1.18597374780656,1.32271144603613));
#22156=CARTESIAN_POINT('Ctrl Pts',(92.7091334567072,-1.11904254874655,1.38057138322055));
#22157=CARTESIAN_POINT('Ctrl Pts',(92.7056370449854,-1.07472279400941,1.41534637248659));
#22158=CARTESIAN_POINT('Ctrl Pts',(92.6931103558333,-0.909051133620568,
1.53306159289965));
#22159=CARTESIAN_POINT('Ctrl Pts',(92.6842278957725,-0.779196297777744,
1.6029663470421));
#22160=CARTESIAN_POINT('Ctrl Pts',(92.6731531225254,-0.619495007711486,
1.66489762911858));
#22161=CARTESIAN_POINT('Ctrl Pts',(92.671563117473,-0.596591405779294,1.67324139942057));
#22162=CARTESIAN_POINT('Ctrl Pts',(92.6690160703683,-0.559997049039636,
1.68572585254875));
#22163=CARTESIAN_POINT('Ctrl Pts',(92.66806931944,-0.546414991197009,1.69017720435915));
#22164=CARTESIAN_POINT('Ctrl Pts',(92.6662658730183,-0.520591620046023,
1.69829670503486));
#22165=CARTESIAN_POINT('Ctrl Pts',(92.6654103194738,-0.50836150123457,1.70199762118008));
#22166=CARTESIAN_POINT('Ctrl Pts',(92.6634465523734,-0.480343410667287,
1.71014715698984));
#22167=CARTESIAN_POINT('Ctrl Pts',(92.6623356119028,-0.464531816512941,
1.71450962395588));
#22168=CARTESIAN_POINT('Ctrl Pts',(92.6588101012366,-0.414492088314664,
1.72757273741767));
#22169=CARTESIAN_POINT('Ctrl Pts',(92.6563702505991,-0.380065498998132,
1.73547145261305));
#22170=CARTESIAN_POINT('Ctrl Pts',(92.6504547129736,-0.297124696358117,
1.7519149336425));
#22171=CARTESIAN_POINT('Ctrl Pts',(92.6469522730853,-0.248447506173411,
1.75947780508053));
#22172=CARTESIAN_POINT('Ctrl Pts',(92.6381958553743,-0.127592410754624,
1.77313966993264));
#22173=CARTESIAN_POINT('Ctrl Pts',(92.632898490908,-0.0552358435429476,
1.77686580972084));
#22174=CARTESIAN_POINT('Ctrl Pts',(92.6215499092297,0.0999696476038994,
1.77536790231446));
#22175=CARTESIAN_POINT('Ctrl Pts',(92.6155130170895,0.18264790660041,1.76877568174811));
#22176=CARTESIAN_POINT('Ctrl Pts',(92.608420214926,0.282625809337143,1.75371608313486));
#22177=CARTESIAN_POINT('Ctrl Pts',(92.607150862131,0.30063887253928,1.75071807597795));
#22178=CARTESIAN_POINT('Ctrl Pts',(92.6052822199219,0.327381534363827,1.74584220691877));
#22179=CARTESIAN_POINT('Ctrl Pts',(92.6046722337553,0.336147769607939,1.74417555484587));
#22180=CARTESIAN_POINT('Ctrl Pts',(92.6035785016835,0.351938807013144,1.74104985726787));
#22181=CARTESIAN_POINT('Ctrl Pts',(92.6030935195458,0.358967683711983,1.73961424913318));
#22182=CARTESIAN_POINT('Ctrl Pts',(92.6019980814948,0.374904017415935,1.73625863816039));
#22183=CARTESIAN_POINT('Ctrl Pts',(92.6013890902225,0.383805615585702,1.73431264176113));
#22184=CARTESIAN_POINT('Ctrl Pts',(92.5995041225156,0.411473383485588,1.728040676784));
#22185=CARTESIAN_POINT('Ctrl Pts',(92.59824064781,0.430185140408706,1.72347780514776));
#22186=CARTESIAN_POINT('Ctrl Pts',(92.5952516530929,0.474733492895714,1.71184388456262));
#22187=CARTESIAN_POINT('Ctrl Pts',(92.5935388206373,0.500492098181849,1.70449088744428));
#22188=CARTESIAN_POINT('Ctrl Pts',(92.5867771191196,0.60257091033138,1.67283785455456));
#22189=CARTESIAN_POINT('Ctrl Pts',(92.5818774607109,0.677379250394012,1.6439699592017));
#22190=CARTESIAN_POINT('Ctrl Pts',(92.5703049807169,0.848278740652362,1.56436709076239));
#22191=CARTESIAN_POINT('Ctrl Pts',(92.5636321382201,0.942160198277295,1.50968601847097));
#22192=CARTESIAN_POINT('Ctrl Pts',(92.5550542281034,1.05066392282222,1.4324050772597));
#22193=CARTESIAN_POINT('Ctrl Pts',(92.5534432425005,1.07055775764301,1.4175983122861));
#22194=CARTESIAN_POINT('Ctrl Pts',(92.5507810355504,1.10259289434307,1.39269593874321));
#22195=CARTESIAN_POINT('Ctrl Pts',(92.5497394018812,1.11492146358133,1.38284604048533));
#22196=CARTESIAN_POINT('Ctrl Pts',(92.5478460131526,1.1369499735396,1.36476030364418));
#22197=CARTESIAN_POINT('Ctrl Pts',(92.5469966190884,1.14669585758813,1.35658192691669));
#22198=CARTESIAN_POINT('Ctrl Pts',(92.5451566192781,1.16750963280789,1.33873124640728));
#22199=CARTESIAN_POINT('Ctrl Pts',(92.5441646414813,1.17854693641908,1.32902490149817));
#22200=CARTESIAN_POINT('Ctrl Pts',(92.5413791568657,1.20902086816311,1.30154759760218));
#22201=CARTESIAN_POINT('Ctrl Pts',(92.5395732593836,1.22818391416243,1.28348032780835));
#22202=CARTESIAN_POINT('Ctrl Pts',(92.5354571556932,1.27051252708568,1.24175593492237));
#22203=CARTESIAN_POINT('Ctrl Pts',(92.5331374083657,1.29343204777661,1.21786418815922));
#22204=CARTESIAN_POINT('Ctrl Pts',(92.525099372151,1.3696864335583,1.13379346799066));
#22205=CARTESIAN_POINT('Ctrl Pts',(92.5192656699838,1.41959244019577,1.07064632140312));
#22206=CARTESIAN_POINT('Ctrl Pts',(92.5056019401028,1.52531764912201,0.916423788946797));
#22207=CARTESIAN_POINT('Ctrl Pts',(92.4977626504106,1.57755751704793,0.823251111969195));
#22208=CARTESIAN_POINT('Ctrl Pts',(92.4890677419122,1.628274704619,0.70999380186209));
#22209=CARTESIAN_POINT('Ctrl Pts',(92.4878535218679,1.6351842881486,0.693932355238349));
#22210=CARTESIAN_POINT('Ctrl Pts',(92.4860495985289,1.64520316973356,0.669662261787435));
#22211=CARTESIAN_POINT('Ctrl Pts',(92.4854502077736,1.64849040222139,0.661528847880037));
#22212=CARTESIAN_POINT('Ctrl Pts',(92.4844156025092,1.65409383589656,0.647363410960038));
#22213=CARTESIAN_POINT('Ctrl Pts',(92.4839788023657,1.65643751288348,0.641342788977989));
#22214=CARTESIAN_POINT('Ctrl Pts',(92.4829455458842,1.66192861107751,0.627005910901365));
#22215=CARTESIAN_POINT('Ctrl Pts',(92.4823508328376,1.6650465042067,0.618678646731392));
#22216=CARTESIAN_POINT('Ctrl Pts',(92.48055622859,1.67431949013696,0.593334434793887));
#22217=CARTESIAN_POINT('Ctrl Pts',(92.4793671835334,1.6802774133147,0.576245939692672));
#22218=CARTESIAN_POINT('Ctrl Pts',(92.4733266640321,1.70950532720676,0.488103826572759));
#22219=CARTESIAN_POINT('Ctrl Pts',(92.4686703251204,1.72853596845471,0.415715877133255));
#22220=CARTESIAN_POINT('Ctrl Pts',(92.4559937631666,1.76816132444284,0.213970194009545));
#22221=CARTESIAN_POINT('Ctrl Pts',(92.4480789421171,1.77911485287178,0.0832213624709728));
#22222=CARTESIAN_POINT('Ctrl Pts',(92.4397243119761,1.77561363837196,-0.0475422940915189));
#22223=CARTESIAN_POINT('Ctrl Pts',(92.2900876926257,1.77561363877829,-0.0475422789160742));
#22224=CARTESIAN_POINT('Ctrl Pts',(92.294987767018,1.77773874190886,0.0318262786811712));
#22225=CARTESIAN_POINT('Ctrl Pts',(92.299947488628,1.77454014362674,0.111251623550904));
#22226=CARTESIAN_POINT('Ctrl Pts',(92.3067711489427,1.76320843930912,0.216466768547959));
#22227=CARTESIAN_POINT('Ctrl Pts',(92.3084907290523,1.7597943916703,0.242663230208114));
#22228=CARTESIAN_POINT('Ctrl Pts',(92.3111906212778,1.75358480229037,0.283228286872694));
#22229=CARTESIAN_POINT('Ctrl Pts',(92.3121581933839,1.75119361238491,0.297655558908998));
#22230=CARTESIAN_POINT('Ctrl Pts',(92.3139692636738,1.74641302368818,0.324444278856811));
#22231=CARTESIAN_POINT('Ctrl Pts',(92.3148112416232,1.74406979714128,0.336813105455989));
#22232=CARTESIAN_POINT('Ctrl Pts',(92.3167006846593,1.7385447089143,0.364372350954233));
#22233=CARTESIAN_POINT('Ctrl Pts',(92.3177502649206,1.7352948641781,0.379547918824588));
#22234=CARTESIAN_POINT('Ctrl Pts',(92.3204518236959,1.72647309803166,0.418257766624543));
#22235=CARTESIAN_POINT('Ctrl Pts',(92.3221126684961,1.72061877619451,0.441723719542048));
#22236=CARTESIAN_POINT('Ctrl Pts',(92.3323813330598,1.68182116594911,0.584737500728853));
#22237=CARTESIAN_POINT('Ctrl Pts',(92.341373129795,1.6369176302476,0.700664633085665));
#22238=CARTESIAN_POINT('Ctrl Pts',(92.3555224661115,1.54858882841298,0.872793298223924));
#22239=CARTESIAN_POINT('Ctrl Pts',(92.3606093291823,1.51325037135594,0.93272168129298));
#22240=CARTESIAN_POINT('Ctrl Pts',(92.3681970566756,1.45415533801439,1.02069885504964));
#22241=CARTESIAN_POINT('Ctrl Pts',(92.370775363499,1.43289246135653,1.05033971835392));
#22242=CARTESIAN_POINT('Ctrl Pts',(92.3740972761119,1.40374997655233,1.08843099795434));
#22243=CARTESIAN_POINT('Ctrl Pts',(92.3748877127732,1.39668098175866,1.09748726041403));
#22244=CARTESIAN_POINT('Ctrl Pts',(92.3761818207207,1.38487616689209,1.11231189188534));
#22245=CARTESIAN_POINT('Ctrl Pts',(92.3766888885216,1.38019107500477,1.11812000492222));
#22246=CARTESIAN_POINT('Ctrl Pts',(92.3777080885485,1.3706502669106,1.12979640484841));
#22247=CARTESIAN_POINT('Ctrl Pts',(92.3782201087548,1.36579315343773,1.13566330315372));
#22248=CARTESIAN_POINT('Ctrl Pts',(92.379546052183,1.35305259198395,1.15085263767614));
#22249=CARTESIAN_POINT('Ctrl Pts',(92.380355851296,1.34511034838335,1.16012554561715));
#22250=CARTESIAN_POINT('Ctrl Pts',(92.3837945206381,1.31072632040991,1.19944250077928));
#22251=CARTESIAN_POINT('Ctrl Pts',(92.3863640710019,1.28336683753283,1.22867241459741));
#22252=CARTESIAN_POINT('Ctrl Pts',(92.3951167659577,1.18537199644857,1.32651800615146));
#22253=CARTESIAN_POINT('Ctrl Pts',(92.4010920226929,1.11003594067722,1.39017249541882));
#22254=CARTESIAN_POINT('Ctrl Pts',(92.4127154989047,0.956130603278522,1.49968505749523));
#22255=CARTESIAN_POINT('Ctrl Pts',(92.4183339807237,0.878564988483435,1.546402894642));
#22256=CARTESIAN_POINT('Ctrl Pts',(92.4258764036786,0.774034383404318,1.59895012751027));
#22257=CARTESIAN_POINT('Ctrl Pts',(92.427606603258,0.750019233320723,1.61035454679107));
#22258=CARTESIAN_POINT('Ctrl Pts',(92.4303194958729,0.71237955984429,1.62720443789726));
#22259=CARTESIAN_POINT('Ctrl Pts',(92.4312892439641,0.698927649773842,1.63302756827052));
#22260=CARTESIAN_POINT('Ctrl Pts',(92.4331023078376,0.673793838062607,1.64354018701132));
#22261=CARTESIAN_POINT('Ctrl Pts',(92.4339440754815,0.662131103875427,1.648273299468));
#22262=CARTESIAN_POINT('Ctrl Pts',(92.4358303421586,0.636017786835537,1.65854905173632));
#22263=CARTESIAN_POINT('Ctrl Pts',(92.4368769228631,0.621543228706961,1.66402751496197));
#22264=CARTESIAN_POINT('Ctrl Pts',(92.4399546736348,0.579030950873135,1.6794858966941));
#22265=CARTESIAN_POINT('Ctrl Pts',(92.442002573838,0.550812983393234,1.68895073659823));
#22266=CARTESIAN_POINT('Ctrl Pts',(92.4537443151974,0.389497776793513,1.73858639498199));
#22267=CARTESIAN_POINT('Ctrl Pts',(92.4639165523496,0.252302620802843,1.76372377578804));
#22268=CARTESIAN_POINT('Ctrl Pts',(92.4794795389711,0.039662934929671,1.77735248070115));
#22269=CARTESIAN_POINT('Ctrl Pts',(92.4848590421069,-0.0345176048229986,
1.77746043892314));
#22270=CARTESIAN_POINT('Ctrl Pts',(92.4913147708779,-0.126413895956299,
1.7718368748879));
#22271=CARTESIAN_POINT('Ctrl Pts',(92.492562408806,-0.144316917094056,1.77046860284157));
#22272=CARTESIAN_POINT('Ctrl Pts',(92.4944020140745,-0.170972001694435,
1.7680244020173));
#22273=CARTESIAN_POINT('Ctrl Pts',(92.4950043149143,-0.179741181007259,
1.76715444363687));
#22274=CARTESIAN_POINT('Ctrl Pts',(92.4960375191919,-0.194863196684076,
1.76554051220674));
#22275=CARTESIAN_POINT('Ctrl Pts',(92.4964700818116,-0.201218870654983,
1.76482745201306));
#22276=CARTESIAN_POINT('Ctrl Pts',(92.4974839651924,-0.216173994872004,
1.76306775382044));
#22277=CARTESIAN_POINT('Ctrl Pts',(92.4980636899817,-0.224769803930325,
1.76199252090491));
#22278=CARTESIAN_POINT('Ctrl Pts',(92.4997838856737,-0.250396181731585,
1.75859637943415));
#22279=CARTESIAN_POINT('Ctrl Pts',(92.5009146908052,-0.267401844096548,
1.75609105150427));
#22280=CARTESIAN_POINT('Ctrl Pts',(92.5108680132218,-0.41819640648147,1.73163409889619));
#22281=CARTESIAN_POINT('Ctrl Pts',(92.5190167665743,-0.549117660468979,
1.69467556524703));
#22282=CARTESIAN_POINT('Ctrl Pts',(92.5326543502629,-0.753853549758228,
1.61062526329925));
#22283=CARTESIAN_POINT('Ctrl Pts',(92.5379944662434,-0.830666872730658,
1.57238642009697));
#22284=CARTESIAN_POINT('Ctrl Pts',(92.5451978271474,-0.926757637741552,
1.51553891879538));
#22285=CARTESIAN_POINT('Ctrl Pts',(92.5468884230646,-0.948806235862827,
1.5018337284582));
#22286=CARTESIAN_POINT('Ctrl Pts',(92.549552822635,-0.982715364505309,1.47971136067804));
#22287=CARTESIAN_POINT('Ctrl Pts',(92.5505144382567,-0.994786819273702,
1.4716230365302));
#22288=CARTESIAN_POINT('Ctrl Pts',(92.5523201423367,-1.01713498364249,1.45624831438887));
#22289=CARTESIAN_POINT('Ctrl Pts',(92.553162787542,-1.02743610358784,1.44899888441667));
#22290=CARTESIAN_POINT('Ctrl Pts',(92.5550613655639,-1.05035455017567,1.43250272590971));
#22291=CARTESIAN_POINT('Ctrl Pts',(92.5561195090194,-1.06292844601215,1.42319774877682));
#22292=CARTESIAN_POINT('Ctrl Pts',(92.5588589737818,-1.09496184097549,1.3988309774537));
#22293=CARTESIAN_POINT('Ctrl Pts',(92.5605495922196,-1.114233639748,1.38352912050741));
#22294=CARTESIAN_POINT('Ctrl Pts',(92.5695486355707,-1.21417802700063,1.30073021477178));
#22295=CARTESIAN_POINT('Ctrl Pts',(92.5771231498474,-1.28904252983136,1.22657664855662));
#22296=CARTESIAN_POINT('Ctrl Pts',(92.590856537093,-1.4104386529885,1.08287129223297));
#22297=CARTESIAN_POINT('Ctrl Pts',(92.5969552881937,-1.45947342815113,1.01581768266667));
#22298=CARTESIAN_POINT('Ctrl Pts',(92.6048679601578,-1.51813545058003,0.922534536726264));
#22299=CARTESIAN_POINT('Ctrl Pts',(92.6068060973843,-1.53209719543812,0.899157138910064));
#22300=CARTESIAN_POINT('Ctrl Pts',(92.6100869176921,-1.55510630912288,0.858537701871372));
#22301=CARTESIAN_POINT('Ctrl Pts',(92.611441460623,-1.56441760704115,0.841451273979836));
#22302=CARTESIAN_POINT('Ctrl Pts',(92.6134057981759,-1.57766683504726,0.816158154560689));
#22303=CARTESIAN_POINT('Ctrl Pts',(92.6140279762,-1.58182512234663,0.808069345461167));
#22304=CARTESIAN_POINT('Ctrl Pts',(92.6151292551768,-1.58912011308265,0.793606818001506));
#22305=CARTESIAN_POINT('Ctrl Pts',(92.6156097883214,-1.5922809282663,0.787245810496631));
#22306=CARTESIAN_POINT('Ctrl Pts',(92.6166770728118,-1.59925120226717,0.773004691110172));
#22307=CARTESIAN_POINT('Ctrl Pts',(92.6172626116304,-1.60304067078751,0.765115204609341));
#22308=CARTESIAN_POINT('Ctrl Pts',(92.6190185484187,-1.61429341002019,0.741236921853471));
#22309=CARTESIAN_POINT('Ctrl Pts',(92.6201786745559,-1.62157716251552,0.725164086171876));
#22310=CARTESIAN_POINT('Ctrl Pts',(92.628165516429,-1.67054628389508,0.6126762952755));
#22311=CARTESIAN_POINT('Ctrl Pts',(92.6345925656338,-1.70385228643998,0.512825763812056));
#22312=CARTESIAN_POINT('Ctrl Pts',(92.6433779569992,-1.73693987947621,0.373568125331418));
#22313=CARTESIAN_POINT('Ctrl Pts',(92.6457139748372,-1.74454694920296,0.336257590118528));
#22314=CARTESIAN_POINT('Ctrl Pts',(92.6533469979423,-1.76532886207983,0.214449147564586));
#22315=CARTESIAN_POINT('Ctrl Pts',(92.6587024785329,-1.77360275802386,0.12924798597122));
#22316=CARTESIAN_POINT('Ctrl Pts',(92.6656531572998,-1.77624256056255,0.0221993833918785));
#22317=CARTESIAN_POINT('Ctrl Pts',(92.6670662336691,-1.77638115751821,0.000602915287913788));
#22318=CARTESIAN_POINT('Ctrl Pts',(92.669390537153,-1.77596501978015,-0.0346097630793831));
#22319=CARTESIAN_POINT('Ctrl Pts',(92.6702943196776,-1.77564741253603,-0.0482269221148783));
#22320=CARTESIAN_POINT('Ctrl Pts',(92.6720576206877,-1.77472730201001,-0.0746400551884794));
#22321=CARTESIAN_POINT('Ctrl Pts',(92.6729165164434,-1.77414291769145,-0.0874358453206651));
#22322=CARTESIAN_POINT('Ctrl Pts',(92.6749522437852,-1.77243864758607,-0.117592192289331));
#22323=CARTESIAN_POINT('Ctrl Pts',(92.6761326622277,-1.77120202490211,-0.134944553389764));
#22324=CARTESIAN_POINT('Ctrl Pts',(92.6801952224641,-1.76610420083517,-0.194190318495858));
#22325=CARTESIAN_POINT('Ctrl Pts',(92.6831151845539,-1.76100995122983,-0.235960517560864));
#22326=CARTESIAN_POINT('Ctrl Pts',(92.6905601174575,-1.74449057140451,-0.340398112601972));
#22327=CARTESIAN_POINT('Ctrl Pts',(92.6951351088823,-1.73116943320391,-0.402702447277033));
#22328=CARTESIAN_POINT('Ctrl Pts',(92.7093429924894,-1.68007805351679,-0.591429151290706));
#22329=CARTESIAN_POINT('Ctrl Pts',(92.7191300311273,-1.63155662081395,-0.714476312882583));
#22330=CARTESIAN_POINT('Ctrl Pts',(92.7296305824709,-1.56148809716388,-0.846840782449819));
#22331=CARTESIAN_POINT('Ctrl Pts',(92.7308742653879,-1.55287563305321,-0.862532154787655));
#22332=CARTESIAN_POINT('Ctrl Pts',(92.7327092329734,-1.53967621480268,-0.885741878761088));
#22333=CARTESIAN_POINT('Ctrl Pts',(92.7333107784125,-1.53526845182023,-0.893360124116083));
#22334=CARTESIAN_POINT('Ctrl Pts',(92.7343911775643,-1.52720215624251,-0.907065635334838));
#22335=CARTESIAN_POINT('Ctrl Pts',(92.7348712175243,-1.52356357968976,-0.91316401353071));
#22336=CARTESIAN_POINT('Ctrl Pts',(92.7359569472055,-1.51520995869963,-0.926976032569233));
#22337=CARTESIAN_POINT('Ctrl Pts',(92.7365611836071,-1.51047249462615,-0.934675684788626));
#22338=CARTESIAN_POINT('Ctrl Pts',(92.7384350523057,-1.49551151705059,-0.958580446001442));
#22339=CARTESIAN_POINT('Ctrl Pts',(92.7396922838651,-1.48508407808564,-0.974657130993974));
#22340=CARTESIAN_POINT('Ctrl Pts',(92.7426677880055,-1.45952791938442,-1.01269606499421));
#22341=CARTESIAN_POINT('Ctrl Pts',(92.7443734474866,-1.44416050480417,-1.03449294518712));
#22342=CARTESIAN_POINT('Ctrl Pts',(92.7511068065287,-1.38090725388352,-1.12005213439666));
#22343=CARTESIAN_POINT('Ctrl Pts',(92.7559860196006,-1.32924063079203,-1.18090755502804));
#22344=CARTESIAN_POINT('Ctrl Pts',(92.767601040113,-1.1973454107804,-1.31659189159709));
#22345=CARTESIAN_POINT('Ctrl Pts',(92.7743366053888,-1.11394873342593,-1.38786342467876));
#22346=CARTESIAN_POINT('Ctrl Pts',(92.7829703475025,-1.004454293915,-1.46517557485391));
#22347=CARTESIAN_POINT('Ctrl Pts',(92.7845671229953,-0.984089734457473,
-1.47893042232661));
#22348=CARTESIAN_POINT('Ctrl Pts',(92.7872053233213,-0.950314011132547,
-1.50073705851073));
#22349=CARTESIAN_POINT('Ctrl Pts',(92.7882373283492,-0.93706985563731,-1.50904224530852));
#22350=CARTESIAN_POINT('Ctrl Pts',(92.7901125573652,-0.912959694795034,
-1.52372153222333));
#22351=CARTESIAN_POINT('Ctrl Pts',(92.7909534595059,-0.902132115214952,
-1.53015696734714));
#22352=CARTESIAN_POINT('Ctrl Pts',(92.7927740639245,-0.878661982245547,
-1.5437708792748));
#22353=CARTESIAN_POINT('Ctrl Pts',(92.7937551012006,-0.865997981439144,
-1.5509103394321));
#22354=CARTESIAN_POINT('Ctrl Pts',(92.7965060246811,-0.830449568001355,
-1.57037997492746));
#22355=CARTESIAN_POINT('Ctrl Pts',(92.7982879630477,-0.807380809313508,
-1.58236400828553));
#22356=CARTESIAN_POINT('Ctrl Pts',(92.806037902137,-0.706922612689067,-1.63178254653194));
#22357=CARTESIAN_POINT('Ctrl Pts',(92.8121753595661,-0.627144916999823,
-1.66407312106551));
#22358=CARTESIAN_POINT('Ctrl Pts',(92.8282280318317,-0.416755723598562,
-1.73194610749768));
#22359=CARTESIAN_POINT('Ctrl Pts',(92.8382670207413,-0.283842019951991,
-1.75862416509129));
#22360=CARTESIAN_POINT('Ctrl Pts',(92.8489426755887,-0.131967366970449,
-1.77142520258336));
#22361=CARTESIAN_POINT('Ctrl Pts',(92.8501424455267,-0.114728114753844,
-1.77262521407942));
#22362=CARTESIAN_POINT('Ctrl Pts',(92.8519258152171,-0.0888058587637963,
-1.7740498678591));
#22363=CARTESIAN_POINT('Ctrl Pts',(92.8525188829277,-0.0801347964154283,
-1.77446268954428));
#22364=CARTESIAN_POINT('Ctrl Pts',(92.8535427350123,-0.0650713359090129,
-1.77506920303215));
#22365=CARTESIAN_POINT('Ctrl Pts',(92.8539750720542,-0.0586805910574123,
-1.77529196069697));
#22366=CARTESIAN_POINT('Ctrl Pts',(92.8549972763407,-0.043499770451354,
-1.77573904058176));
#22367=CARTESIAN_POINT('Ctrl Pts',(92.8555854417489,-0.0347090632694041,
-1.77593261679578));
#22368=CARTESIAN_POINT('Ctrl Pts',(92.8573576629775,-0.00806599157180379,
-1.77632140402357));
#22369=CARTESIAN_POINT('Ctrl Pts',(92.8585311648445,0.00978882064814059,
-1.77631276228262));
#22370=CARTESIAN_POINT('Ctrl Pts',(92.8644538701237,0.10078924922353,-1.77489647848007));
#22371=CARTESIAN_POINT('Ctrl Pts',(92.8690157025129,0.173805461101921,-1.76923995003621));
#22372=CARTESIAN_POINT('Ctrl Pts',(92.8819226752765,0.380990431400312,-1.7402342419735));
#22373=CARTESIAN_POINT('Ctrl Pts',(92.8901417484114,0.513086004069158,-1.70596288561294));
#22374=CARTESIAN_POINT('Ctrl Pts',(92.9009428844723,0.670493073098504,-1.64516668689581));
#22375=CARTESIAN_POINT('Ctrl Pts',(92.9030606670229,0.700678502751117,-1.63253906780276));
#22376=CARTESIAN_POINT('Ctrl Pts',(92.9062453815342,0.744937988223441,-1.61257014221255));
#22377=CARTESIAN_POINT('Ctrl Pts',(92.9072908592143,0.759291152228356,-1.60586175896308));
#22378=CARTESIAN_POINT('Ctrl Pts',(92.9091804995949,0.784904880870786,-1.59347024957454));
#22379=CARTESIAN_POINT('Ctrl Pts',(92.9100221759129,0.796198405856377,-1.58785742203266));
#22380=CARTESIAN_POINT('Ctrl Pts',(92.9118332624201,0.82024717163652,-1.57558423321915));
#22381=CARTESIAN_POINT('Ctrl Pts',(92.9128038837592,0.832983093777067,-1.56888821869952));
#22382=CARTESIAN_POINT('Ctrl Pts',(92.9154944337239,0.867858883395908,-1.55000761916097));
#22383=CARTESIAN_POINT('Ctrl Pts',(92.9172255664099,0.889821496161764,-1.53750455324515));
#22384=CARTESIAN_POINT('Ctrl Pts',(92.9265825735306,1.00594600170679,-1.4680746381808));
#22385=CARTESIAN_POINT('Ctrl Pts',(92.9345044964078,1.09491681564403,-1.40296834600878));
#22386=CARTESIAN_POINT('Ctrl Pts',(92.9507684492121,1.261700320557,-1.25534304369367));
#22387=CARTESIAN_POINT('Ctrl Pts',(92.9590771381228,1.33881923461502,-1.17274920566313));
#22388=CARTESIAN_POINT('Ctrl Pts',(92.9681488101624,1.41784771484333,-1.07007225831311));
#22389=CARTESIAN_POINT('Ctrl Pts',(92.9693160168416,1.42791405245832,-1.05660223861011));
#22390=CARTESIAN_POINT('Ctrl Pts',(92.9710685270796,1.44289362569969,-1.03595253286846));
#22391=CARTESIAN_POINT('Ctrl Pts',(92.9716626114668,1.44794760102437,-1.0288767750056));
#22392=CARTESIAN_POINT('Ctrl Pts',(92.9726874417418,1.45662760961242,-1.01653379318001));
#22393=CARTESIAN_POINT('Ctrl Pts',(92.9731197524237,1.46027735690318,-1.01128383251189));
#22394=CARTESIAN_POINT('Ctrl Pts',(92.9741409257841,1.46887000479777,-0.998780261454234));
#22395=CARTESIAN_POINT('Ctrl Pts',(92.9747280986733,1.47378758752764,-0.991509584760297));
#22396=CARTESIAN_POINT('Ctrl Pts',(92.9764941560305,1.48849959716133,-0.969406481638364));
#22397=CARTESIAN_POINT('Ctrl Pts',(92.9776625937753,1.49812581509776,-0.954462717259428));
#22398=CARTESIAN_POINT('Ctrl Pts',(92.9835331813231,1.54582731357498,-0.877910566718759));
#22399=CARTESIAN_POINT('Ctrl Pts',(92.9880516045662,1.58033745437071,-0.814152859592063));
#22400=CARTESIAN_POINT('Ctrl Pts',(93.0007769139332,1.66722499257112,-0.627150462620073));
#22401=CARTESIAN_POINT('Ctrl Pts',(93.0088578646156,1.70970251470316,-0.499872162206162));
#22402=CARTESIAN_POINT('Ctrl Pts',(93.0196222502321,1.74471640461645,-0.335019313572613));
#22403=CARTESIAN_POINT('Ctrl Pts',(93.0218695209038,1.75094016173377,-0.300801539050298));
#22404=CARTESIAN_POINT('Ctrl Pts',(93.0252105521052,1.75858696203341,-0.250397201374686));
#22405=CARTESIAN_POINT('Ctrl Pts',(93.0262795593992,1.76079890823176,-0.234337443227318));
#22406=CARTESIAN_POINT('Ctrl Pts',(93.0281949261588,1.76434459485241,-0.205699181151343));
#22407=CARTESIAN_POINT('Ctrl Pts',(93.0290385118307,1.76576439394069,-0.193132320955662));
#22408=CARTESIAN_POINT('Ctrl Pts',(93.0308357108636,1.76848920871186,-0.166464696108202));
#22409=CARTESIAN_POINT('Ctrl Pts',(93.0317903400181,1.76976002827542,-0.152361407354624));
#22410=CARTESIAN_POINT('Ctrl Pts',(93.0343890140194,1.77274330016713,-0.114146850572733));
#22411=CARTESIAN_POINT('Ctrl Pts',(93.036043024397,1.77413237049621,-0.0900141281322493));
#22412=CARTESIAN_POINT('Ctrl Pts',(93.0381340219422,1.77525508472944,-0.0597559735022117));
#22413=CARTESIAN_POINT('Ctrl Pts',(93.0385568852539,1.77545011806415,-0.0536494645266197));
#22414=CARTESIAN_POINT('Ctrl Pts',(93.0389806716583,1.77561363839032,-0.047542293405874));
#22415=CARTESIAN_POINT('Origin',(88.3562164250559,0.,0.));
#22416=CARTESIAN_POINT('',(93.9380452419004,1.77561363831514,-0.0475422962136777));
#22417=CARTESIAN_POINT('',(93.7915308001226,1.77561363900531,-0.0475422704373303));
#22418=CARTESIAN_POINT('',(88.3562164250559,1.77561363837197,-0.0475422940912398));
#22419=CARTESIAN_POINT('Ctrl Pts',(93.9380452419004,1.77561363825831,-0.0475422983361156));
#22420=CARTESIAN_POINT('Ctrl Pts',(93.932064216968,1.77342400896609,-0.129320751841116));
#22421=CARTESIAN_POINT('Ctrl Pts',(93.9261040070707,1.76558700019008,-0.210863377491231));
#22422=CARTESIAN_POINT('Ctrl Pts',(93.9190812768447,1.74915389466268,-0.309610326783592));
#22423=CARTESIAN_POINT('Ctrl Pts',(93.9178110419327,1.74587644207947,-0.327587264195588));
#22424=CARTESIAN_POINT('Ctrl Pts',(93.9159413667903,1.74058590020062,-0.354266068078609));
#22425=CARTESIAN_POINT('Ctrl Pts',(93.91533121331,1.73878377173417,-0.363007888016686));
#22426=CARTESIAN_POINT('Ctrl Pts',(93.9142373160668,1.7354143951053,-0.378751113415867));
#22427=CARTESIAN_POINT('Ctrl Pts',(93.9137523340385,1.73387055425268,-0.385756962503964));
#22428=CARTESIAN_POINT('Ctrl Pts',(93.9126570636886,1.73027011386946,-0.401637109181372));
#22429=CARTESIAN_POINT('Ctrl Pts',(93.9120482378743,1.72818765190767,-0.410505156209504));
#22430=CARTESIAN_POINT('Ctrl Pts',(93.9101643333073,1.72149364249509,-0.438057115724141));
#22431=CARTESIAN_POINT('Ctrl Pts',(93.9089017361248,1.71664645406548,-0.456683066593837));
#22432=CARTESIAN_POINT('Ctrl Pts',(93.90591523603,1.70433858489328,-0.501008964669987));
#22433=CARTESIAN_POINT('Ctrl Pts',(93.9042039922161,1.69659787990215,-0.526626793382687));
#22434=CARTESIAN_POINT('Ctrl Pts',(93.8974529160954,1.66343481159347,-0.62804411997303));
#22435=CARTESIAN_POINT('Ctrl Pts',(93.8925618212592,1.63348585505973,-0.702268062299535));
#22436=CARTESIAN_POINT('Ctrl Pts',(93.8809715838332,1.55118372057922,-0.872207090092294));
#22437=CARTESIAN_POINT('Ctrl Pts',(93.874272408138,1.49482937438349,-0.965607449451407));
#22438=CARTESIAN_POINT('Ctrl Pts',(93.8656731771968,1.41565681372803,-1.07312085861627));
#22439=CARTESIAN_POINT('Ctrl Pts',(93.8640703636354,1.40061768571666,-1.09267680249015));
#22440=CARTESIAN_POINT('Ctrl Pts',(93.861418855841,1.37532214927653,-1.12418898498729));
#22441=CARTESIAN_POINT('Ctrl Pts',(93.8603796150051,1.36530503797323,-1.13633358434851));
#22442=CARTESIAN_POINT('Ctrl Pts',(93.8584887546109,1.34690442392916,-1.15804764228581));
#22443=CARTESIAN_POINT('Ctrl Pts',(93.8576394664736,1.3385769371677,-1.16766332382448));
#22444=CARTESIAN_POINT('Ctrl Pts',(93.8557976223561,1.32038746768316,-1.18821625067455));
#22445=CARTESIAN_POINT('Ctrl Pts',(93.8548036708995,1.31049136404233,-1.19912188086078));
#22446=CARTESIAN_POINT('Ctrl Pts',(93.8520066669708,1.2824285230712,-1.22928515362792));
#22447=CARTESIAN_POINT('Ctrl Pts',(93.8501910566705,1.26396582768971,-1.24826085435847));
#22448=CARTESIAN_POINT('Ctrl Pts',(93.8422084260967,1.18177136168752,-1.32904546997689));
#22449=CARTESIAN_POINT('Ctrl Pts',(93.8358602738192,1.1138888730116,-1.38643171477092));
#22450=CARTESIAN_POINT('Ctrl Pts',(93.8224679770277,0.964697794219947,-1.49450194901544));
#22451=CARTESIAN_POINT('Ctrl Pts',(93.8154283348047,0.882995729582544,-1.54418152978826));
#22452=CARTESIAN_POINT('Ctrl Pts',(93.8053773149932,0.758325683220617,-1.60684409208148));
#22453=CARTESIAN_POINT('Ctrl Pts',(93.8022430019592,0.718227858245852,-1.6251631357424));
#22454=CARTESIAN_POINT('Ctrl Pts',(93.7983047182628,0.665801556143529,-1.64679450459689));
#22455=CARTESIAN_POINT('Ctrl Pts',(93.7974331205392,0.654064777535289,-1.65149118750045));
#22456=CARTESIAN_POINT('Ctrl Pts',(93.7960379210879,0.635044049802805,-1.6588680857658));
#22457=CARTESIAN_POINT('Ctrl Pts',(93.795509938176,0.627791172951811,-1.66162646830613));
#22458=CARTESIAN_POINT('Ctrl Pts',(93.7944779178436,0.613501445865366,-1.66695415364624));
#22459=CARTESIAN_POINT('Ctrl Pts',(93.7939737213439,0.606466034953206,-1.66952661740373));
#22460=CARTESIAN_POINT('Ctrl Pts',(93.7927099653469,0.588701764907681,-1.67589492649203));
#22461=CARTESIAN_POINT('Ctrl Pts',(93.7919537529158,0.577952071837437,-1.67963239794334));
#22462=CARTESIAN_POINT('Ctrl Pts',(93.7889032835193,0.534139226941025,-1.69439488180496));
#22463=CARTESIAN_POINT('Ctrl Pts',(93.7866540261119,0.500788615839324,-1.70454975542391));
#22464=CARTESIAN_POINT('Ctrl Pts',(93.7803590766397,0.405257858930089,-1.7305913803883));
#22465=CARTESIAN_POINT('Ctrl Pts',(93.7763965102849,0.342484219541614,-1.7441003834496));
#22466=CARTESIAN_POINT('Ctrl Pts',(93.764318786301,0.148456156966097,-1.77497277442892));
#22467=CARTESIAN_POINT('Ctrl Pts',(93.7562682297953,0.0158998081696953,
-1.78109817790297));
#22468=CARTESIAN_POINT('Ctrl Pts',(93.7460632877515,-0.141988959481852,
-1.77075581746317));
#22469=CARTESIAN_POINT('Ctrl Pts',(93.7443744812903,-0.167833692495375,
-1.76849336144285));
#22470=CARTESIAN_POINT('Ctrl Pts',(93.7416967620832,-0.208297311049322,
-1.764056220399));
#22471=CARTESIAN_POINT('Ctrl Pts',(93.74071982405,-0.222955011140102,-1.76226364639208));
#22472=CARTESIAN_POINT('Ctrl Pts',(93.7388907482296,-0.250191254348781,
-1.75858753744992));
#22473=CARTESIAN_POINT('Ctrl Pts',(93.738040157464,-0.262775290960008,-1.75675124094689));
#22474=CARTESIAN_POINT('Ctrl Pts',(93.7361304787226,-0.290838456750996,
-1.75234791812534));
#22475=CARTESIAN_POINT('Ctrl Pts',(93.7350692228578,-0.306305309374883,
-1.74971062291305));
#22476=CARTESIAN_POINT('Ctrl Pts',(93.7318657030709,-0.352596240795009,
-1.74118485278453));
#22477=CARTESIAN_POINT('Ctrl Pts',(93.7297043162238,-0.383299832116641,
-1.73468435794648));
#22478=CARTESIAN_POINT('Ctrl Pts',(93.7206554325429,-0.509611182069572,
-1.70442493991075));
#22479=CARTESIAN_POINT('Ctrl Pts',(93.7135523773192,-0.603320151802286,
-1.67354940206419));
#22480=CARTESIAN_POINT('Ctrl Pts',(93.6980298144184,-0.799045927245915,
-1.59047738940703));
#22481=CARTESIAN_POINT('Ctrl Pts',(93.6896133338755,-0.899580743631573,
-1.53585513859791));
#22482=CARTESIAN_POINT('Ctrl Pts',(93.6804485128342,-1.00806719754256,-1.46258171375491));
#22483=CARTESIAN_POINT('Ctrl Pts',(93.6792856212177,-1.0218179624261,-1.45300820598767));
#22484=CARTESIAN_POINT('Ctrl Pts',(93.6775347847855,-1.04252738539006,-1.4381505396072));
#22485=CARTESIAN_POINT('Ctrl Pts',(93.6769381694574,-1.04958550466908,-1.43300753674767));
#22486=CARTESIAN_POINT('Ctrl Pts',(93.6759062149524,-1.06180067900675,-1.42396809982054));
#22487=CARTESIAN_POINT('Ctrl Pts',(93.6754693236448,-1.06697466237805,-1.42009538560277));
#22488=CARTESIAN_POINT('Ctrl Pts',(93.674433167974,-1.07925086259638,-1.41080170758836));
#22489=CARTESIAN_POINT('Ctrl Pts',(93.6738356808908,-1.08633346065656,-1.40535529436161));
#22490=CARTESIAN_POINT('Ctrl Pts',(93.6720237361292,-1.10781112677829,-1.38857989178399));
#22491=CARTESIAN_POINT('Ctrl Pts',(93.6708204332204,-1.122072809844,-1.37708107320852));
#22492=CARTESIAN_POINT('Ctrl Pts',(93.6646287406169,-1.19526853983663,-1.31617297336947));
#22493=CARTESIAN_POINT('Ctrl Pts',(93.6598464708331,-1.25113231978726,-1.2631899063244));
#22494=CARTESIAN_POINT('Ctrl Pts',(93.6461755011858,-1.40187971177965,-1.10036971653318));
#22495=CARTESIAN_POINT('Ctrl Pts',(93.6374037849479,-1.48696623616425,-0.982348083167489));
#22496=CARTESIAN_POINT('Ctrl Pts',(93.6264415414659,-1.56863900284259,-0.833692832635021));
#22497=CARTESIAN_POINT('Ctrl Pts',(93.624833548212,-1.5800604031398,-0.811838090916207));
#22498=CARTESIAN_POINT('Ctrl Pts',(93.622264443553,-1.59740379672548,-0.77689841321814));
#22499=CARTESIAN_POINT('Ctrl Pts',(93.6213139409969,-1.60362863692112,-0.763966758907573));
#22500=CARTESIAN_POINT('Ctrl Pts',(93.6195075397764,-1.61509352061627,-0.739391625501737));
#22501=CARTESIAN_POINT('Ctrl Pts',(93.6186528350781,-1.62036607857833,-0.727764256389499));
#22502=CARTESIAN_POINT('Ctrl Pts',(93.6166969355332,-1.632084061398,-0.701164302350791));
#22503=CARTESIAN_POINT('Ctrl Pts',(93.6155930937495,-1.63844955509484,-0.686157989688276));
#22504=CARTESIAN_POINT('Ctrl Pts',(93.6121149429335,-1.657729938153,-0.638906851947309));
#22505=CARTESIAN_POINT('Ctrl Pts',(93.60971631391,-1.66990544092752,-0.606371205076973));
#22506=CARTESIAN_POINT('Ctrl Pts',(93.5958472210486,-1.73395018128646,-0.418635307898377));
#22507=CARTESIAN_POINT('Ctrl Pts',(93.5837104342289,-1.76512212983418,-0.25722489164812));
#22508=CARTESIAN_POINT('Ctrl Pts',(93.5682221334524,-1.77644160955396,-0.0433518631493959));
#22509=CARTESIAN_POINT('Ctrl Pts',(93.564608095318,-1.77695590541709,0.00727127327235955));
#22510=CARTESIAN_POINT('Ctrl Pts',(93.560174877126,-1.77487894761392,0.0710073011846654));
#22511=CARTESIAN_POINT('Ctrl Pts',(93.5592664760859,-1.77430401511516,0.0841582040911155));
#22512=CARTESIAN_POINT('Ctrl Pts',(93.5578269487021,-1.7731516629115,0.105162834718707));
#22513=CARTESIAN_POINT('Ctrl Pts',(93.5572909506516,-1.77266813518198,0.113020927663279));
#22514=CARTESIAN_POINT('Ctrl Pts',(93.5562557660819,-1.77162767430701,0.128274893734556));
#22515=CARTESIAN_POINT('Ctrl Pts',(93.5557562975695,-1.7710766448611,0.135670870770977));
#22516=CARTESIAN_POINT('Ctrl Pts',(93.5545220997813,-1.7695931518056,0.154029834762301));
#22517=CARTESIAN_POINT('Ctrl Pts',(93.5537903901603,-1.76860510070327,0.164988260380485));
#22518=CARTESIAN_POINT('Ctrl Pts',(93.5509731565614,-1.76438019789977,0.207432851803631));
#22519=CARTESIAN_POINT('Ctrl Pts',(93.548924408518,-1.76040362424818,0.23884145600169));
#22520=CARTESIAN_POINT('Ctrl Pts',(93.543404046258,-1.74724592875639,0.324354284080489));
#22521=CARTESIAN_POINT('Ctrl Pts',(93.5399930567425,-1.73639401043948,0.37816755531454));
#22522=CARTESIAN_POINT('Ctrl Pts',(93.5280587394473,-1.68939917133564,0.565873043702462));
#22523=CARTESIAN_POINT('Ctrl Pts',(93.5196813388008,-1.6401076225318,0.695935467971167));
#22524=CARTESIAN_POINT('Ctrl Pts',(93.5088562955244,-1.56233175632845,0.845628750530105));
#22525=CARTESIAN_POINT('Ctrl Pts',(93.5069060880123,-1.54779135251087,0.871957716502482));
#22526=CARTESIAN_POINT('Ctrl Pts',(93.5039064464908,-1.52468859299561,0.91139074682668));
#22527=CARTESIAN_POINT('Ctrl Pts',(93.5028743129305,-1.51660943717015,0.924772506087227));
#22528=CARTESIAN_POINT('Ctrl Pts',(93.5009909083532,-1.50164055397037,0.948842114339685));
#22529=CARTESIAN_POINT('Ctrl Pts',(93.5001418808112,-1.49481060048346,0.959566029770632));
#22530=CARTESIAN_POINT('Ctrl Pts',(93.4982942950274,-1.47977513833724,0.982623543970468));
#22531=CARTESIAN_POINT('Ctrl Pts',(93.4972942696386,-1.4715293371001,0.99492958346697));
#22532=CARTESIAN_POINT('Ctrl Pts',(93.4944616961243,-1.44787832792654,1.02928909489754));
#22533=CARTESIAN_POINT('Ctrl Pts',(93.4926160676028,-1.43212523293026,1.05109698531739));
#22534=CARTESIAN_POINT('Ctrl Pts',(93.4843708327006,-1.36028536199637,1.14593458366941));
#22535=CARTESIAN_POINT('Ctrl Pts',(93.4777755866483,-1.29907227904524,1.21488643308539));
#22536=CARTESIAN_POINT('Ctrl Pts',(93.4636616329492,-1.15946108251805,1.34947827119889));
#22537=CARTESIAN_POINT('Ctrl Pts',(93.456143853353,-1.08017482561964,1.41374140241039));
#22538=CARTESIAN_POINT('Ctrl Pts',(93.4463221822853,-0.966532815612609,
1.4906807011022));
#22539=CARTESIAN_POINT('Ctrl Pts',(93.4438221933532,-0.936661568546289,
1.50962913814869));
#22540=CARTESIAN_POINT('Ctrl Pts',(93.4405544940258,-0.896110940857078,
1.53368445529899));
#22541=CARTESIAN_POINT('Ctrl Pts',(93.4397435695085,-0.885919748459911,
1.53959379218729));
#22542=CARTESIAN_POINT('Ctrl Pts',(93.4384726747304,-0.869733103171513,
1.54876562395411));
#22543=CARTESIAN_POINT('Ctrl Pts',(93.4380086083511,-0.863776562230541,
1.55209557799372));
#22544=CARTESIAN_POINT('Ctrl Pts',(93.4370408123907,-0.851254522718967,
1.55900150379228));
#22545=CARTESIAN_POINT('Ctrl Pts',(93.436537565545,-0.844685385861342,1.56257049546946));
#22546=CARTESIAN_POINT('Ctrl Pts',(93.4352796184397,-0.828125200432104,
1.57143264153487));
#22547=CARTESIAN_POINT('Ctrl Pts',(93.4345282005413,-0.818105559289383,
1.57667219324101));
#22548=CARTESIAN_POINT('Ctrl Pts',(93.4315250359133,-0.777579800567155,
1.59737389586408));
#22549=CARTESIAN_POINT('Ctrl Pts',(93.4293165488909,-0.746677998174211,
1.61205025819796));
#22550=CARTESIAN_POINT('Ctrl Pts',(93.4231848078267,-0.658459581322483,
1.65086667977955));
#22551=CARTESIAN_POINT('Ctrl Pts',(93.4193396320445,-0.600270196795669,
1.67290363377777));
#22552=CARTESIAN_POINT('Ctrl Pts',(93.4071631902648,-0.411708830257406,
1.73320438443527));
#22553=CARTESIAN_POINT('Ctrl Pts',(93.3989135625157,-0.278074791546838,
1.75959425939188));
#22554=CARTESIAN_POINT('Ctrl Pts',(93.3885033343085,-0.117266968741904,
1.77255911488489));
#22555=CARTESIAN_POINT('Ctrl Pts',(93.3868387516293,-0.091749743853286,
1.77406291742127));
#22556=CARTESIAN_POINT('Ctrl Pts',(93.3841909620317,-0.0515359169358551,
1.77556293580235));
#22557=CARTESIAN_POINT('Ctrl Pts',(93.3832192815249,-0.0368560317405538,
1.77592829271832));
#22558=CARTESIAN_POINT('Ctrl Pts',(93.3813949405143,-0.00945079146547175,
1.77627043037224));
#22559=CARTESIAN_POINT('Ctrl Pts',(93.3805437583539,0.00327312796116224,
1.7762925523013));
#22560=CARTESIAN_POINT('Ctrl Pts',(93.3786260024962,0.0317936252256098,
1.77603570235679));
#22561=CARTESIAN_POINT('Ctrl Pts',(93.3775571756645,0.0475882793237433,
1.77568267946322));
#22562=CARTESIAN_POINT('Ctrl Pts',(93.3743059484304,0.0953160979571939,
1.77397869043863));
#22563=CARTESIAN_POINT('Ctrl Pts',(93.3721035673673,0.127217980976721,1.77197655411225));
#22564=CARTESIAN_POINT('Ctrl Pts',(93.3583083801192,0.324308754421789,1.75425772207082));
#22565=CARTESIAN_POINT('Ctrl Pts',(93.3460112670075,0.486656738414632,1.71631634661313));
#22566=CARTESIAN_POINT('Ctrl Pts',(93.3302160596375,0.690152138386397,1.63752688002723));
#22567=CARTESIAN_POINT('Ctrl Pts',(93.3264731440086,0.738113413084914,1.61647577076743));
#22568=CARTESIAN_POINT('Ctrl Pts',(93.3219094459022,0.79698626544526,1.58746753174659));
#22569=CARTESIAN_POINT('Ctrl Pts',(93.3209931537949,0.808827980177294,1.58146691291037));
#22570=CARTESIAN_POINT('Ctrl Pts',(93.3195441289377,0.827605422254967,1.57168562023021));
#22571=CARTESIAN_POINT('Ctrl Pts',(93.319006416856,0.834584864468106,1.56799060390182));
#22572=CARTESIAN_POINT('Ctrl Pts',(93.3179704197863,0.848058580154164,1.56074197225628));
#22573=CARTESIAN_POINT('Ctrl Pts',(93.3174718273927,0.854555611178217,1.55719413337679));
#22574=CARTESIAN_POINT('Ctrl Pts',(93.3162433146843,0.870589558154492,1.54830789216091));
#22575=CARTESIAN_POINT('Ctrl Pts',(93.3155163515095,0.880099950627387,1.54292177368071));
#22576=CARTESIAN_POINT('Ctrl Pts',(93.312741991114,0.916450523592709,1.5218895004793));
#22577=CARTESIAN_POINT('Ctrl Pts',(93.3107299544161,0.942929867873822,1.50562703030943));
#22578=CARTESIAN_POINT('Ctrl Pts',(93.3053443244942,1.01362306236464,1.45961326572982));
#22579=CARTESIAN_POINT('Ctrl Pts',(93.302027819328,1.05694824863634,1.42855303378692));
#22580=CARTESIAN_POINT('Ctrl Pts',(93.2905649303247,1.2028616076847,1.31366853968444));
#22581=CARTESIAN_POINT('Ctrl Pts',(93.2825652740839,1.2974146084182,1.22037476729893));
#22582=CARTESIAN_POINT('Ctrl Pts',(93.2720476895369,1.40113835850593,1.09221276734445));
#22583=CARTESIAN_POINT('Ctrl Pts',(93.2699547525255,1.42085984449617,1.06643074083501));
#22584=CARTESIAN_POINT('Ctrl Pts',(93.2667838138539,1.44928484549225,1.02708148635314));
#22585=CARTESIAN_POINT('Ctrl Pts',(93.2657263319464,1.45852866177532,1.01391176035958));
#22586=CARTESIAN_POINT('Ctrl Pts',(93.2638747197923,1.47429708362159,0.990784456891326));
#22587=CARTESIAN_POINT('Ctrl Pts',(93.2630837143151,1.48090295627574,0.980883353485329));
#22588=CARTESIAN_POINT('Ctrl Pts',(93.2614149077411,1.49456336596262,0.959956110432165));
#22589=CARTESIAN_POINT('Ctrl Pts',(93.2605363710762,1.50159649830148,0.948916924290748));
#22590=CARTESIAN_POINT('Ctrl Pts',(93.2584080895476,1.51825042759562,0.92212812921801));
#22591=CARTESIAN_POINT('Ctrl Pts',(93.25715395688,1.52774884051114,0.906304630340698));
#22592=CARTESIAN_POINT('Ctrl Pts',(93.2525459688191,1.56149398299845,0.848049983425419));
#22593=CARTESIAN_POINT('Ctrl Pts',(93.2491394620652,1.58423151366537,0.804774472179879));
#22594=CARTESIAN_POINT('Ctrl Pts',(93.2399716105195,1.63966345229121,0.687795151691299));
#22595=CARTESIAN_POINT('Ctrl Pts',(93.2341238888131,1.66917312532955,0.612712951792597));
#22596=CARTESIAN_POINT('Ctrl Pts',(93.2204713262312,1.7255377664724,0.43459480648691));
#22597=CARTESIAN_POINT('Ctrl Pts',(93.2126582125065,1.74844221397177,0.330615576841279));
#22598=CARTESIAN_POINT('Ctrl Pts',(93.2039837022445,1.76413778331815,0.207819983310635));
#22599=CARTESIAN_POINT('Ctrl Pts',(93.2027663351122,1.7661026566286,0.190401491911574));
#22600=CARTESIAN_POINT('Ctrl Pts',(93.2009587090377,1.76866447420252,0.164216762282819));
#22601=CARTESIAN_POINT('Ctrl Pts',(93.2003587061771,1.76945469378544,0.155471097681425));
#22602=CARTESIAN_POINT('Ctrl Pts',(93.1993235127337,1.77071367410087,0.140281441403671));
#22603=CARTESIAN_POINT('Ctrl Pts',(93.1988867291409,1.77121216870269,0.1338404093729));
#22604=CARTESIAN_POINT('Ctrl Pts',(93.1978540964208,1.77231258804181,0.118537110675026));
#22605=CARTESIAN_POINT('Ctrl Pts',(93.1972599832262,1.7728831956536,0.109672874277451));
#22606=CARTESIAN_POINT('Ctrl Pts',(93.1954691157638,1.77441151937427,0.082786078274788));
#22607=CARTESIAN_POINT('Ctrl Pts',(93.1942831416912,1.7751611148671,0.0647522416044393));
#22608=CARTESIAN_POINT('Ctrl Pts',(93.1910644008543,1.77646221521149,0.015291391870698));
#22609=CARTESIAN_POINT('Ctrl Pts',(93.1890567017321,1.77645452257652,-0.0161368862966694));
#22610=CARTESIAN_POINT('Ctrl Pts',(93.1870734170205,1.77561363809212,-0.0475423045429159));
#22611=CARTESIAN_POINT('Ctrl Pts',(93.0389806716583,1.77561363839032,-0.047542293405874));
#22612=CARTESIAN_POINT('Ctrl Pts',(93.0406142785543,1.77624397463933,-0.0240004412921055));
#22613=CARTESIAN_POINT('Ctrl Pts',(93.0422616476878,1.77640604792239,-0.000448753302874027));
#22614=CARTESIAN_POINT('Ctrl Pts',(93.0486331855031,1.77523068615551,0.0899260868132504));
#22615=CARTESIAN_POINT('Ctrl Pts',(93.0534448008932,1.77059074467301,0.156644745852565));
#22616=CARTESIAN_POINT('Ctrl Pts',(93.0656822186869,1.74948528761673,0.323472131199964));
#22617=CARTESIAN_POINT('Ctrl Pts',(93.0731601714229,1.72818673807063,0.422734339993162));
#22618=CARTESIAN_POINT('Ctrl Pts',(93.0830061780318,1.68796328643129,0.554212140705317));
#22619=CARTESIAN_POINT('Ctrl Pts',(93.0855633978304,1.67633262754556,0.588456023419935));
#22620=CARTESIAN_POINT('Ctrl Pts',(93.0888879996843,1.65952821414169,0.63337943210798));
#22621=CARTESIAN_POINT('Ctrl Pts',(93.08970069677,1.65528231549723,0.644394191123166));
#22622=CARTESIAN_POINT('Ctrl Pts',(93.0909706465522,1.64842388787623,0.661671191850491));
#22623=CARTESIAN_POINT('Ctrl Pts',(93.091432041536,1.6458848409825,0.667961955793922));
#22624=CARTESIAN_POINT('Ctrl Pts',(93.0923901448549,1.64051209253187,0.6810568688574));
#22625=CARTESIAN_POINT('Ctrl Pts',(93.092886415574,1.63767198186023,0.687858173508663));
#22626=CARTESIAN_POINT('Ctrl Pts',(93.0941195709511,1.63047380726,0.704798562713444));
#22627=CARTESIAN_POINT('Ctrl Pts',(93.0948533729094,1.62606333629056,0.714915304100834));
#22628=CARTESIAN_POINT('Ctrl Pts',(93.097725857473,1.60830876588358,0.754626271998064));
#22629=CARTESIAN_POINT('Ctrl Pts',(93.0998256718011,1.59424786945938,0.783895362317591));
#22630=CARTESIAN_POINT('Ctrl Pts',(93.1055471244885,1.55318058095326,0.86369869612356));
#22631=CARTESIAN_POINT('Ctrl Pts',(93.1091023449359,1.52451919295323,0.913338648689704));
#22632=CARTESIAN_POINT('Ctrl Pts',(93.1215850284528,1.41485156146095,1.0836847163296));
#22633=CARTESIAN_POINT('Ctrl Pts',(93.1303761840958,1.32151150240489,1.19573448139649));
#22634=CARTESIAN_POINT('Ctrl Pts',(93.1413352204001,1.19789011291407,1.31175887919233));
#22635=CARTESIAN_POINT('Ctrl Pts',(93.1429165699177,1.17987151840116,1.32798915189923));
#22636=CARTESIAN_POINT('Ctrl Pts',(93.1454555967787,1.15070050009218,1.35320257218564));
#22637=CARTESIAN_POINT('Ctrl Pts',(93.1464031659091,1.13976157589448,1.36242885032582));
#22638=CARTESIAN_POINT('Ctrl Pts',(93.1481126797813,1.11994161809837,1.37873995664914));
#22639=CARTESIAN_POINT('Ctrl Pts',(93.1488725757104,1.11110174388814,1.38587373176154));
#22640=CARTESIAN_POINT('Ctrl Pts',(93.1506667936614,1.09016453962537,1.40244096541801));
#22641=CARTESIAN_POINT('Ctrl Pts',(93.1517038725532,1.07801238571957,1.41180333452864));
#22642=CARTESIAN_POINT('Ctrl Pts',(93.1547897455314,1.04171626110587,1.4390250616293));
#22643=CARTESIAN_POINT('Ctrl Pts',(93.1568558100862,1.01723998919406,1.45643005664982));
#22644=CARTESIAN_POINT('Ctrl Pts',(93.1616930092813,0.959565114260596,1.49527924154872));
#22645=CARTESIAN_POINT('Ctrl Pts',(93.1644795358848,0.926069503570083,1.51625199095094));
#22646=CARTESIAN_POINT('Ctrl Pts',(93.1754864340768,0.79264514446526,1.59372261243583));
#22647=CARTESIAN_POINT('Ctrl Pts',(93.1839418669352,0.688038806069294,1.64159567293732));
#22648=CARTESIAN_POINT('Ctrl Pts',(93.197088608169,0.517299364806754,1.70053041041206));
#22649=CARTESIAN_POINT('Ctrl Pts',(93.2018332248535,0.453884512140813,1.71854386208169));
#22650=CARTESIAN_POINT('Ctrl Pts',(93.207380256267,0.37614108235373,1.73602203725509));
#22651=CARTESIAN_POINT('Ctrl Pts',(93.2083340204843,0.362637351062339,1.73889298372775));
#22652=CARTESIAN_POINT('Ctrl Pts',(93.2098247392325,0.341294153731156,1.74317117888793));
#22653=CARTESIAN_POINT('Ctrl Pts',(93.2103672280361,0.333476671794237,1.7446835741515));
#22654=CARTESIAN_POINT('Ctrl Pts',(93.2113982471524,0.318517420158293,1.74747341762132));
#22655=CARTESIAN_POINT('Ctrl Pts',(93.2118872261099,0.311377666597152,1.74875974415353));
#22656=CARTESIAN_POINT('Ctrl Pts',(93.2130717604991,0.293976992228449,1.75178477392434));
#22657=CARTESIAN_POINT('Ctrl Pts',(93.21376476097,0.283708094846553,1.75347714446922));
#22658=CARTESIAN_POINT('Ctrl Pts',(93.2162802638395,0.246135712383341,1.75933056339864));
#22659=CARTESIAN_POINT('Ctrl Pts',(93.2180751483871,0.218749562331486,1.7629451635433));
#22660=CARTESIAN_POINT('Ctrl Pts',(93.2227096208673,0.146899423847069,1.77072813619613));
#22661=CARTESIAN_POINT('Ctrl Pts',(93.2255095900357,0.102341807918322,1.77386139570429));
#22662=CARTESIAN_POINT('Ctrl Pts',(93.2370736032073,-0.0838922325888598,
1.77991537877549));
#22663=CARTESIAN_POINT('Ctrl Pts',(93.2455785451679,-0.22553060572245,1.76756116460121));
#22664=CARTESIAN_POINT('Ctrl Pts',(93.2570031888832,-0.401287777423312,
1.73074209958905));
#22665=CARTESIAN_POINT('Ctrl Pts',(93.2594440932583,-0.438117233915936,
1.72178775120697));
#22666=CARTESIAN_POINT('Ctrl Pts',(93.2629354818483,-0.489562397813883,
1.70752242608633));
#22667=CARTESIAN_POINT('Ctrl Pts',(93.2639548771397,-0.504439354457537,
1.70318674535118));
#22668=CARTESIAN_POINT('Ctrl Pts',(93.2658312884794,-0.531547261307627,
1.69490021202221));
#22669=CARTESIAN_POINT('Ctrl Pts',(93.2666862778402,-0.543795800889764,
1.69101015131005));
#22670=CARTESIAN_POINT('Ctrl Pts',(93.2684344849686,-0.568623976363802,
1.68282723111918));
#22671=CARTESIAN_POINT('Ctrl Pts',(93.2693279523319,-0.581199769257263,
1.67852540278963));
#22672=CARTESIAN_POINT('Ctrl Pts',(93.2715773640878,-0.612570379016939,
1.66739958569441));
#22673=CARTESIAN_POINT('Ctrl Pts',(93.2729391025499,-0.631300050194068,
1.66039875847731));
#22674=CARTESIAN_POINT('Ctrl Pts',(93.278682914961,-0.709185480412747,1.62977823698092));
#22675=CARTESIAN_POINT('Ctrl Pts',(93.2831588674551,-0.767160632073596,
1.60330409336184));
#22676=CARTESIAN_POINT('Ctrl Pts',(93.297749016221,-0.947781610391456,1.50878215246473));
#22677=CARTESIAN_POINT('Ctrl Pts',(93.3081697953428,-1.06383609902388,1.42932194886656));
#22678=CARTESIAN_POINT('Ctrl Pts',(93.3209500804986,-1.19797147017989,1.31201192604106));
#22679=CARTESIAN_POINT('Ctrl Pts',(93.3236443248948,-1.22579470575232,1.28605550140802));
#22680=CARTESIAN_POINT('Ctrl Pts',(93.3271157809467,-1.26128187343392,1.25075034695414));
#22681=CARTESIAN_POINT('Ctrl Pts',(93.3279432511827,-1.26971286354833,1.2421906692488));
#22682=CARTESIAN_POINT('Ctrl Pts',(93.3292819208889,-1.28331664506931,1.22809601373978));
#22683=CARTESIAN_POINT('Ctrl Pts',(93.329796968343,-1.28854186172002,1.22261249238358));
#22684=CARTESIAN_POINT('Ctrl Pts',(93.3308164614659,-1.29887028192478,1.21163372659912));
#22685=CARTESIAN_POINT('Ctrl Pts',(93.3313209432362,-1.30397406428339,1.20613927098943));
#22686=CARTESIAN_POINT('Ctrl Pts',(93.3326035601201,-1.31692671924963,1.1920168278806));
#22687=CARTESIAN_POINT('Ctrl Pts',(93.3333780641369,-1.324725843107,1.18334338234599));
#22688=CARTESIAN_POINT('Ctrl Pts',(93.3366631962968,-1.35767785559932,1.145963169055));
#22689=CARTESIAN_POINT('Ctrl Pts',(93.339119361292,-1.38198928905391,1.11652444281191));
#22690=CARTESIAN_POINT('Ctrl Pts',(93.3463101330933,-1.45139980505251,1.02673066215157));
#22691=CARTESIAN_POINT('Ctrl Pts',(93.3509305280875,-1.49363060060257,0.964264694474558));
#22692=CARTESIAN_POINT('Ctrl Pts',(93.3626478694777,-1.59028020971078,0.799642686601972));
#22693=CARTESIAN_POINT('Ctrl Pts',(93.3697367552534,-1.63891871868585,0.694522286231583));
#22694=CARTESIAN_POINT('Ctrl Pts',(93.3787567435776,-1.68506539264836,0.562331906409825));
#22695=CARTESIAN_POINT('Ctrl Pts',(93.3803466255576,-1.692650053789,0.539071658408503));
#22696=CARTESIAN_POINT('Ctrl Pts',(93.3829757995194,-1.70428075436109,0.500734023055078));
#22697=CARTESIAN_POINT('Ctrl Pts',(93.3840057839586,-1.7086128539619,0.48574637506263));
#22698=CARTESIAN_POINT('Ctrl Pts',(93.3858788744068,-1.71608414496795,0.458560648444357));
#22699=CARTESIAN_POINT('Ctrl Pts',(93.3867196832692,-1.71929211456859,0.44638242756821));
#22700=CARTESIAN_POINT('Ctrl Pts',(93.3885418269849,-1.72592949021877,0.420051769619085));
#22701=CARTESIAN_POINT('Ctrl Pts',(93.3895245162812,-1.72931487899894,0.405889297229369));
#22702=CARTESIAN_POINT('Ctrl Pts',(93.392285060387,-1.73828315310545,0.366220483378832));
#22703=CARTESIAN_POINT('Ctrl Pts',(93.3940751050549,-1.74347813766206,0.340631208172091));
#22704=CARTESIAN_POINT('Ctrl Pts',(93.4018936776905,-1.76350125577842,0.229490071266932));
#22705=CARTESIAN_POINT('Ctrl Pts',(93.4080952562282,-1.77260764200031,0.143040757421338));
#22706=CARTESIAN_POINT('Ctrl Pts',(93.424104297921,-1.77959104605296,-0.0772390947565849));
#22707=CARTESIAN_POINT('Ctrl Pts',(93.4340248105918,-1.76874811271193,-0.210814917675523));
#22708=CARTESIAN_POINT('Ctrl Pts',(93.4446186809813,-1.73964816193103,-0.35916181805912));
#22709=CARTESIAN_POINT('Ctrl Pts',(93.4458394396303,-1.73600918469313,-0.376357686041292));
#22710=CARTESIAN_POINT('Ctrl Pts',(93.4476474962382,-1.73017954805635,-0.402018848997123));
#22711=CARTESIAN_POINT('Ctrl Pts',(93.4482446376791,-1.72818078142562,-0.410526026340157));
#22712=CARTESIAN_POINT('Ctrl Pts',(93.4493207481165,-1.72444350544355,-0.425921496159045));
#22713=CARTESIAN_POINT('Ctrl Pts',(93.4498008501261,-1.72272639017773,-0.432814409202329));
#22714=CARTESIAN_POINT('Ctrl Pts',(93.4508912563302,-1.7187127185108,-0.448523855111298));
#22715=CARTESIAN_POINT('Ctrl Pts',(93.451500049308,-1.71638963534372,-0.457333233113122));
#22716=CARTESIAN_POINT('Ctrl Pts',(93.4534034045911,-1.70887087216756,-0.48498067230348));
#22717=CARTESIAN_POINT('Ctrl Pts',(93.4546850024889,-1.7034318598969,-0.503751809866261));
#22718=CARTESIAN_POINT('Ctrl Pts',(93.4577300252228,-1.68962964951911,-0.54860332533262));
#22719=CARTESIAN_POINT('Ctrl Pts',(93.4594800312124,-1.68097076911431,-0.574588021751886));
#22720=CARTESIAN_POINT('Ctrl Pts',(93.466515811897,-1.64335272897686,-0.679335583647343));
#22721=CARTESIAN_POINT('Ctrl Pts',(93.471639356881,-1.60942924039693,-0.756203922295841));
#22722=CARTESIAN_POINT('Ctrl Pts',(93.4831735720289,-1.52160944990598,-0.922263628436107));
#22723=CARTESIAN_POINT('Ctrl Pts',(93.489584903079,-1.46505874127027,-1.00968563248125));
#22724=CARTESIAN_POINT('Ctrl Pts',(93.497863123968,-1.38606887330017,-1.11107284058865));
#22725=CARTESIAN_POINT('Ctrl Pts',(93.4994623237408,-1.37054187152664,-1.13017019179927));
#22726=CARTESIAN_POINT('Ctrl Pts',(93.5021036978561,-1.3445048728511,-1.16086839592352));
#22727=CARTESIAN_POINT('Ctrl Pts',(93.5031364127707,-1.33422916091378,-1.17266419141022));
#22728=CARTESIAN_POINT('Ctrl Pts',(93.505012394501,-1.31540058506222,-1.19371019572356));
#22729=CARTESIAN_POINT('Ctrl Pts',(93.505853330792,-1.3069024821671,-1.20300815400473));
#22730=CARTESIAN_POINT('Ctrl Pts',(93.5076734013209,-1.288390654785,-1.22283469382464));
#22731=CARTESIAN_POINT('Ctrl Pts',(93.5086538637808,-1.2783452531001,-1.23333229899567));
#22732=CARTESIAN_POINT('Ctrl Pts',(93.5114014431643,-1.24999990051939,-1.2622352855805));
#22733=CARTESIAN_POINT('Ctrl Pts',(93.513180564556,-1.23142428719495,-1.28036392024195));
#22734=CARTESIAN_POINT('Ctrl Pts',(93.5209067693397,-1.14985390140676,-1.35655404644318));
#22735=CARTESIAN_POINT('Ctrl Pts',(93.5270220766126,-1.08310942369822,-1.41041594077166));
#22736=CARTESIAN_POINT('Ctrl Pts',(93.5430902851623,-0.901298634263778,
-1.53659654082754));
#22737=CARTESIAN_POINT('Ctrl Pts',(93.5531707714034,-0.781352520423305,
-1.60092441130058));
#22738=CARTESIAN_POINT('Ctrl Pts',(93.5638748452446,-0.63928758717903,-1.6573081732651));
#22739=CARTESIAN_POINT('Ctrl Pts',(93.5650671292812,-0.623233289410249,
-1.66341195196184));
#22740=CARTESIAN_POINT('Ctrl Pts',(93.566841682871,-0.59895402814274,-1.67224194591509));
#22741=CARTESIAN_POINT('Ctrl Pts',(93.5674332879617,-0.590794040287253,
-1.67514222184071));
#22742=CARTESIAN_POINT('Ctrl Pts',(93.5684557389121,-0.576571059152577,
-1.68008058781324));
#22743=CARTESIAN_POINT('Ctrl Pts',(93.5688881199724,-0.570517969440732,
-1.68214571825519));
#22744=CARTESIAN_POINT('Ctrl Pts',(93.5699118342719,-0.556095656455988,
-1.68697936678798));
#22745=CARTESIAN_POINT('Ctrl Pts',(93.5705014481086,-0.547716818794986,
-1.68971833681279));
#22746=CARTESIAN_POINT('Ctrl Pts',(93.5722826874621,-0.522197447845928,
-1.69785062848668));
#22747=CARTESIAN_POINT('Ctrl Pts',(93.5734636011663,-0.504994567596273,
-1.70304652867212));
#22748=CARTESIAN_POINT('Ctrl Pts',(93.5794633113212,-0.416325137294466,
-1.72836614199646));
#22749=CARTESIAN_POINT('Ctrl Pts',(93.5840892859787,-0.343719100184372,
-1.74425793981282));
#22750=CARTESIAN_POINT('Ctrl Pts',(93.5972697631542,-0.132483169000386,
-1.77678444263114));
#22751=CARTESIAN_POINT('Ctrl Pts',(93.6056984043662,0.00736560038765615,
-1.78170078744151));
#22752=CARTESIAN_POINT('Ctrl Pts',(93.6163760857269,0.173059326225834,-1.76800253109418));
#22753=CARTESIAN_POINT('Ctrl Pts',(93.6181137572511,0.199716908733858,-1.76518993772296));
#22754=CARTESIAN_POINT('Ctrl Pts',(93.6209359564715,0.242435528103644,-1.75970274251314));
#22755=CARTESIAN_POINT('Ctrl Pts',(93.6220086385425,0.258541777319047,-1.75740856018637));
#22756=CARTESIAN_POINT('Ctrl Pts',(93.6239280788793,0.287114737630044,-1.75293733199359));
#22757=CARTESIAN_POINT('Ctrl Pts',(93.6247720183785,0.299594121137149,-1.75084765494246));
#22758=CARTESIAN_POINT('Ctrl Pts',(93.6265673228836,0.32595791259679,-1.74614291976344));
#22759=CARTESIAN_POINT('Ctrl Pts',(93.6275196752413,0.339835514082865,-1.74349518504779));
#22760=CARTESIAN_POINT('Ctrl Pts',(93.6301053351699,0.377214501751471,-1.73590035285499));
#22761=CARTESIAN_POINT('Ctrl Pts',(93.6317484378353,0.400648825719022,-1.73064185643832));
#22762=CARTESIAN_POINT('Ctrl Pts',(93.6354372238,0.452531851930095,-1.71788944563346));
#22763=CARTESIAN_POINT('Ctrl Pts',(93.6374898119668,0.480915020752726,-1.71016075126501));
#22764=CARTESIAN_POINT('Ctrl Pts',(93.6442070844146,0.572235747237687,-1.68284113952823));
#22765=CARTESIAN_POINT('Ctrl Pts',(93.6489494740752,0.634273448957008,-1.66045287928878));
#22766=CARTESIAN_POINT('Ctrl Pts',(93.6609455689353,0.786037517344467,-1.5959361436853));
#22767=CARTESIAN_POINT('Ctrl Pts',(93.6682500317492,0.873758085446539,-1.54964977862052));
#22768=CARTESIAN_POINT('Ctrl Pts',(93.6781763639195,0.990238545375748,-1.47513833322026));
#22769=CARTESIAN_POINT('Ctrl Pts',(93.6809596625256,1.02260385476284,-1.45288931172616));
#22770=CARTESIAN_POINT('Ctrl Pts',(93.6845254577908,1.06397539720641,-1.42238100028658));
#22771=CARTESIAN_POINT('Ctrl Pts',(93.6853615654813,1.07366947045865,-1.41507782280452));
#22772=CARTESIAN_POINT('Ctrl Pts',(93.6867106462214,1.08931179493333,-1.40304014426578));
#22773=CARTESIAN_POINT('Ctrl Pts',(93.687227575559,1.09530566104463,-1.39836595617888));
#22774=CARTESIAN_POINT('Ctrl Pts',(93.6882474037055,1.10713462570381,-1.38901866907892));
#22775=CARTESIAN_POINT('Ctrl Pts',(93.6887503698382,1.1129705645062,-1.38434694684716));
#22776=CARTESIAN_POINT('Ctrl Pts',(93.6900241067932,1.12774915105447,-1.37236268954325));
#22777=CARTESIAN_POINT('Ctrl Pts',(93.6907913461591,1.13665046274147,-1.36499935623864));
#22778=CARTESIAN_POINT('Ctrl Pts',(93.6939978552124,1.17381288887357,-1.33364226613764));
#22779=CARTESIAN_POINT('Ctrl Pts',(93.6963858510205,1.20139313028419,-1.30885193374254));
#22780=CARTESIAN_POINT('Ctrl Pts',(93.7032746749132,1.27985350078847,-1.23375661584138));
#22781=CARTESIAN_POINT('Ctrl Pts',(93.7076721859276,1.32849666361159,-1.181219021491));
#22782=CARTESIAN_POINT('Ctrl Pts',(93.719491892003,1.45052343439877,-1.0323183553378));
#22783=CARTESIAN_POINT('Ctrl Pts',(93.7268930778586,1.51743747596037,-0.931170761123306));
#22784=CARTESIAN_POINT('Ctrl Pts',(93.736253958162,1.58483166639567,-0.802473594830802));
#22785=CARTESIAN_POINT('Ctrl Pts',(93.7378344106899,1.59566760071422,-0.780704872442546));
#22786=CARTESIAN_POINT('Ctrl Pts',(93.7404512344874,1.61269830521266,-0.744654469483821));
#22787=CARTESIAN_POINT('Ctrl Pts',(93.7414784508323,1.61915843455582,-0.730501225633464));
#22788=CARTESIAN_POINT('Ctrl Pts',(93.7433486220229,1.63050890130123,-0.704743440816549));
#22789=CARTESIAN_POINT('Ctrl Pts',(93.7441893135793,1.63546338126657,-0.693168167969974));
#22790=CARTESIAN_POINT('Ctrl Pts',(93.7460136170739,1.64589405277667,-0.668064235254204));
#22791=CARTESIAN_POINT('Ctrl Pts',(93.7469986104917,1.65132736618654,-0.654518878940241));
#22792=CARTESIAN_POINT('Ctrl Pts',(93.7497725941038,1.66607201194726,-0.616407543386504));
#22793=CARTESIAN_POINT('Ctrl Pts',(93.7515739676873,1.67500582486124,-0.591700571709546));
#22794=CARTESIAN_POINT('Ctrl Pts',(93.7594892978949,1.71148069428218,-0.483371806523794));
#22795=CARTESIAN_POINT('Ctrl Pts',(93.7657814445003,1.73332768841504,-0.397976869663198));
#22796=CARTESIAN_POINT('Ctrl Pts',(93.7764962663586,1.75916937453405,-0.252820987874083));
#22797=CARTESIAN_POINT('Ctrl Pts',(93.7808533281167,1.76664216406746,-0.193831279908814));
#22798=CARTESIAN_POINT('Ctrl Pts',(93.7873138516248,1.77334623387469,-0.105601855031709));
#22799=CARTESIAN_POINT('Ctrl Pts',(93.7894295803521,1.77483613273508,-0.0765806551991079));
#22800=CARTESIAN_POINT('Ctrl Pts',(93.79153079842,1.7756136390086,-0.0475422703142009));
#22801=CARTESIAN_POINT('Origin',(88.3562164250559,0.,0.));
#22802=CARTESIAN_POINT('',(94.6900676319114,1.77561363837122,-0.0475422941192622));
#22803=CARTESIAN_POINT('',(94.5412649413994,1.77561364082572,-0.0475422024484503));
#22804=CARTESIAN_POINT('',(88.3562164250559,1.77561363837197,-0.0475422940912398));
#22805=CARTESIAN_POINT('Ctrl Pts',(94.6900676319114,1.77561363837047,-0.0475422941472846));
#22806=CARTESIAN_POINT('Ctrl Pts',(94.6893374515194,1.77532329368649,-0.0583861120561661));
#22807=CARTESIAN_POINT('Ctrl Pts',(94.6886041642756,1.77493362258899,-0.0692269101151485));
#22808=CARTESIAN_POINT('Ctrl Pts',(94.6861231269635,1.77328633428699,-0.105735780798001));
#22809=CARTESIAN_POINT('Ctrl Pts',(94.6843612362446,1.77157104388246,-0.131378821437202));
#22810=CARTESIAN_POINT('Ctrl Pts',(94.6732661564457,1.75740653431339,-0.291030668250471));
#22811=CARTESIAN_POINT('Ctrl Pts',(94.6634727861833,1.73031769151216,-0.423278290624867));
#22812=CARTESIAN_POINT('Ctrl Pts',(94.6490381426011,1.66906605814486,-0.610928612591884));
#22813=CARTESIAN_POINT('Ctrl Pts',(94.6444502734985,1.6464015994563,-0.669610258070475));
#22814=CARTESIAN_POINT('Ctrl Pts',(94.6374965125478,1.60658286213221,-0.758380334676792));
#22815=CARTESIAN_POINT('Ctrl Pts',(94.6350661121503,1.5915818465348,-0.789377488560802));
#22816=CARTESIAN_POINT('Ctrl Pts',(94.6318978470677,1.57045723920818,-0.829973818142713));
#22817=CARTESIAN_POINT('Ctrl Pts',(94.6311184460216,1.56513006046956,-0.839976422134724));
#22818=CARTESIAN_POINT('Ctrl Pts',(94.6298340962298,1.5561277531675,-0.856496609803153));
#22819=CARTESIAN_POINT('Ctrl Pts',(94.6293259141241,1.55250658654819,-0.863043065485869));
#22820=CARTESIAN_POINT('Ctrl Pts',(94.6282952337822,1.54503884003291,-0.87634437415588));
#22821=CARTESIAN_POINT('Ctrl Pts',(94.6277729419677,1.54118909821517,-0.883097190977505));
#22822=CARTESIAN_POINT('Ctrl Pts',(94.626404267074,1.53093162946895,-0.900818385219357));
#22823=CARTESIAN_POINT('Ctrl Pts',(94.6255624403535,1.5244502259585,-0.911743905312175));
#22824=CARTESIAN_POINT('Ctrl Pts',(94.6217892606524,1.49464841198525,-0.960773575382697));
#22825=CARTESIAN_POINT('Ctrl Pts',(94.6189322313152,1.47001083714337,-0.998062424214972));
#22826=CARTESIAN_POINT('Ctrl Pts',(94.6101405256078,1.38866051089384,-1.11162659655119));
#22827=CARTESIAN_POINT('Ctrl Pts',(94.6043726783083,1.32721869853184,-1.18430749471312));
#22828=CARTESIAN_POINT('Ctrl Pts',(94.5930713966691,1.19785774846736,-1.31454968153972));
#22829=CARTESIAN_POINT('Ctrl Pts',(94.5875642335257,1.13085765647851,-1.37261154852834));
#22830=CARTESIAN_POINT('Ctrl Pts',(94.5801508325271,1.03859273067365,-1.44121075572246));
#22831=CARTESIAN_POINT('Ctrl Pts',(94.5784295087121,1.01702350042697,-1.45651171768604));
#22832=CARTESIAN_POINT('Ctrl Pts',(94.5757215184839,0.982928583068523,-1.47957160759876));
#22833=CARTESIAN_POINT('Ctrl Pts',(94.5747475580119,0.970633798589597,-1.48766620870782));
#22834=CARTESIAN_POINT('Ctrl Pts',(94.5729211758183,0.947529175157864,-1.50246941530146));
#22835=CARTESIAN_POINT('Ctrl Pts',(94.5720702623001,0.936745052639939,-1.50921654294944));
#22836=CARTESIAN_POINT('Ctrl Pts',(94.5701560688634,0.912448093814269,-1.52405728910833));
#22837=CARTESIAN_POINT('Ctrl Pts',(94.5690905733052,0.898898343640544,-1.53208807980124));
#22838=CARTESIAN_POINT('Ctrl Pts',(94.5663374345393,0.863833107380073,-1.55224558014611));
#22839=CARTESIAN_POINT('Ctrl Pts',(94.5646404701187,0.842168879709873,-1.56410531932907));
#22840=CARTESIAN_POINT('Ctrl Pts',(94.5556614541638,0.72732008628012,-1.62389963563221));
#22841=CARTESIAN_POINT('Ctrl Pts',(94.548115758263,0.630289607248745,-1.66396308995811));
#22842=CARTESIAN_POINT('Ctrl Pts',(94.5344082194848,0.451082534983792,-1.72002321734563));
#22843=CARTESIAN_POINT('Ctrl Pts',(94.5283057451115,0.370213076920247,-1.73922350816295));
#22844=CARTESIAN_POINT('Ctrl Pts',(94.5203841746582,0.261368930872614,-1.75712691441568));
#22845=CARTESIAN_POINT('Ctrl Pts',(94.5184412413556,0.234342525185479,-1.76093510727185));
#22846=CARTESIAN_POINT('Ctrl Pts',(94.5151506770191,0.187845216956855,-1.76639732115271));
#22847=CARTESIAN_POINT('Ctrl Pts',(94.5137911805211,0.168415447642005,-1.76835563079447));
#22848=CARTESIAN_POINT('Ctrl Pts',(94.5118173957431,0.139827634018304,-1.77076148006389));
#22849=CARTESIAN_POINT('Ctrl Pts',(94.5111906683815,0.130692836792508,-1.77145910994884));
#22850=CARTESIAN_POINT('Ctrl Pts',(94.5100800024859,0.114394418493414,-1.77257706829787));
#22851=CARTESIAN_POINT('Ctrl Pts',(94.5095946261354,0.107233180361402,-1.77302470270061));
#22852=CARTESIAN_POINT('Ctrl Pts',(94.5085141801711,0.0912056668894408,
-1.77392908473936));
#22853=CARTESIAN_POINT('Ctrl Pts',(94.5079203775127,0.0823384688998834,
-1.77436277472453));
#22854=CARTESIAN_POINT('Ctrl Pts',(94.5061314426169,0.0554608507568541,
-1.77547542232024));
#22855=CARTESIAN_POINT('Ctrl Pts',(94.5049470565469,0.0374423872332112,
-1.77594679264801));
#22856=CARTESIAN_POINT('Ctrl Pts',(94.4976226473424,-0.0751355753381771,
-1.77717763609404));
#22857=CARTESIAN_POINT('Ctrl Pts',(94.4918022655074,-0.169634026652738,
-1.77065932009031));
#22858=CARTESIAN_POINT('Ctrl Pts',(94.4782464675659,-0.387937841560564,
-1.73795389651269));
#22859=CARTESIAN_POINT('Ctrl Pts',(94.4705389267968,-0.510341176426477,
-1.70602670806349));
#22860=CARTESIAN_POINT('Ctrl Pts',(94.4607475474385,-0.652208696669796,
-1.65237401569988));
#22861=CARTESIAN_POINT('Ctrl Pts',(94.4590838711563,-0.675893644146779,
-1.64282797224383));
#22862=CARTESIAN_POINT('Ctrl Pts',(94.4564465028495,-0.712723212967857,
-1.62705282831613));
#22863=CARTESIAN_POINT('Ctrl Pts',(94.4554844293663,-0.726011681660081,
-1.62116695666736));
#22864=CARTESIAN_POINT('Ctrl Pts',(94.4536684694263,-0.750810297153695,
-1.60981684200193));
#22865=CARTESIAN_POINT('Ctrl Pts',(94.4528159340303,-0.762336845134641,
-1.6043905032895));
#22866=CARTESIAN_POINT('Ctrl Pts',(94.4508820805722,-0.788216608979539,
-1.59186526668863));
#22867=CARTESIAN_POINT('Ctrl Pts',(94.4497983416878,-0.802534038311092,
-1.58469540857963));
#22868=CARTESIAN_POINT('Ctrl Pts',(94.4464517788779,-0.846165971533108,
-1.56210254280354));
#22869=CARTESIAN_POINT('Ctrl Pts',(94.4441672037941,-0.875146139580199,
-1.54605309898268));
#22870=CARTESIAN_POINT('Ctrl Pts',(94.4323924040923,-1.02037565184145,-1.46023198679797));
#22871=CARTESIAN_POINT('Ctrl Pts',(94.4224632205585,-1.1287959833686,-1.37813351488065));
#22872=CARTESIAN_POINT('Ctrl Pts',(94.4072430933574,-1.27952273879188,-1.23417966700966));
#22873=CARTESIAN_POINT('Ctrl Pts',(94.4019540389607,-1.32909471514766,-1.18062998039253));
#22874=CARTESIAN_POINT('Ctrl Pts',(94.3955873617998,-1.38656557139963,-1.11032439354308));
#22875=CARTESIAN_POINT('Ctrl Pts',(94.3943437695617,-1.39768260143938,-1.09629729073699));
#22876=CARTESIAN_POINT('Ctrl Pts',(94.3925053278173,-1.41397953445161,-1.07508339852437));
#22877=CARTESIAN_POINT('Ctrl Pts',(94.3919002584852,-1.41932041220726,-1.06802247802508));
#22878=CARTESIAN_POINT('Ctrl Pts',(94.3908600475587,-1.42846633488624,-1.05574130965536));
#22879=CARTESIAN_POINT('Ctrl Pts',(94.3904232530224,-1.43229592600246,-1.05053994056219));
#22880=CARTESIAN_POINT('Ctrl Pts',(94.3893954280319,-1.44128126104364,-1.03819554296366));
#22881=CARTESIAN_POINT('Ctrl Pts',(94.3888060740894,-1.44641234559371,-1.03103491387593));
#22882=CARTESIAN_POINT('Ctrl Pts',(94.3870446909205,-1.46167506337268,-1.00939699652882));
#22883=CARTESIAN_POINT('Ctrl Pts',(94.3858829284997,-1.47164449465209,-0.994805924285774));
#22884=CARTESIAN_POINT('Ctrl Pts',(94.3778842867471,-1.53944013882501,-0.892331255709796));
#22885=CARTESIAN_POINT('Ctrl Pts',(94.3714481301101,-1.58958400814105,-0.799599560930391));
#22886=CARTESIAN_POINT('Ctrl Pts',(94.3600092359002,-1.66333984383855,-0.628449063888252));
#22887=CARTESIAN_POINT('Ctrl Pts',(94.3550301136434,-1.69030649370887,-0.551824689823842));
#22888=CARTESIAN_POINT('Ctrl Pts',(94.3468206407555,-1.72502387187582,-0.42633832116108));
#22889=CARTESIAN_POINT('Ctrl Pts',(94.3436817704253,-1.73614141110801,-0.378528810246688));
#22890=CARTESIAN_POINT('Ctrl Pts',(94.3392747009371,-1.7487020001742,-0.312164897040442));
#22891=CARTESIAN_POINT('Ctrl Pts',(94.3380603739705,-1.75185512837645,-0.293954376083439));
#22892=CARTESIAN_POINT('Ctrl Pts',(94.3359702840145,-1.75675580004252,-0.262763336384444));
#22893=CARTESIAN_POINT('Ctrl Pts',(94.3350990659994,-1.75864500923082,-0.249806380547978));
#22894=CARTESIAN_POINT('Ctrl Pts',(94.3333215322251,-1.76218828575521,-0.223468708354198));
#22895=CARTESIAN_POINT('Ctrl Pts',(94.3324150010505,-1.76383359686637,-0.210087703592546));
#22896=CARTESIAN_POINT('Ctrl Pts',(94.3301191666405,-1.76759409278264,-0.176336537589576));
#22897=CARTESIAN_POINT('Ctrl Pts',(94.3287236932569,-1.76950955184938,-0.155946580303943));
#22898=CARTESIAN_POINT('Ctrl Pts',(94.3230276537799,-1.77583743956784,-0.073254593266782));
#22899=CARTESIAN_POINT('Ctrl Pts',(94.3186379483455,-1.77731456176376,-0.0107795545668774));
#22900=CARTESIAN_POINT('Ctrl Pts',(94.3043426769924,-1.77150701968772,0.18890634582484));
#22901=CARTESIAN_POINT('Ctrl Pts',(94.2941433169928,-1.75161086856034,0.325233890425397));
#22902=CARTESIAN_POINT('Ctrl Pts',(94.2813585991203,-1.7057481420427,0.49712727467627));
#22903=CARTESIAN_POINT('Ctrl Pts',(94.2784776287621,-1.69393969129844,0.535986135145742));
#22904=CARTESIAN_POINT('Ctrl Pts',(94.274803909654,-1.67681993706431,0.586081143204528));
#22905=CARTESIAN_POINT('Ctrl Pts',(94.2739538902563,-1.67270948431136,0.597711644840104));
#22906=CARTESIAN_POINT('Ctrl Pts',(94.2725846952867,-1.6658391543421,0.616525066251105));
#22907=CARTESIAN_POINT('Ctrl Pts',(94.2720614174575,-1.66315326214235,0.623734300639063));
#22908=CARTESIAN_POINT('Ctrl Pts',(94.2710306852491,-1.65774122754958,0.637977259474338));
#22909=CARTESIAN_POINT('Ctrl Pts',(94.2705231476407,-1.65501696665022,0.64501147694608));
#22910=CARTESIAN_POINT('Ctrl Pts',(94.2692393470779,-1.64797710019312,0.662850588400758));
#22911=CARTESIAN_POINT('Ctrl Pts',(94.2684666560659,-1.64359990349287,0.673631056693287));
#22912=CARTESIAN_POINT('Ctrl Pts',(94.2652467297818,-1.62478474101254,0.718694893084872));
#22913=CARTESIAN_POINT('Ctrl Pts',(94.2628510300613,-1.60937655816748,0.752565842649512));
#22914=CARTESIAN_POINT('Ctrl Pts',(94.2559421657426,-1.5611726968115,0.850264866256651));
#22915=CARTESIAN_POINT('Ctrl Pts',(94.2515325657993,-1.52556009584107,0.91262167407638));
#22916=CARTESIAN_POINT('Ctrl Pts',(94.2397399594445,-1.42037917791901,1.0733436565479));
#22917=CARTESIAN_POINT('Ctrl Pts',(94.2323765982472,-1.34443429641627,1.16706303439117));
#22918=CARTESIAN_POINT('Ctrl Pts',(94.2230516045925,-1.24238243993935,1.26970331890244));
#22919=CARTESIAN_POINT('Ctrl Pts',(94.2214641821524,-1.22480632970158,1.2866662377068));
#22920=CARTESIAN_POINT('Ctrl Pts',(94.2188328325687,-1.19538807113728,1.31390906364636));
#22921=CARTESIAN_POINT('Ctrl Pts',(94.2177981081761,-1.18374933191899,1.32440445523666));
#22922=CARTESIAN_POINT('Ctrl Pts',(94.2159119952549,-1.16241806197842,1.34313439925979));
#22923=CARTESIAN_POINT('Ctrl Pts',(94.2150628822803,-1.15277297514628,1.35142155473046));
#22924=CARTESIAN_POINT('Ctrl Pts',(94.2132174362284,-1.13172616754371,1.36911592562504));
#22925=CARTESIAN_POINT('Ctrl Pts',(94.2122196625026,-1.12029440772412,1.37848574641721));
#22926=CARTESIAN_POINT('Ctrl Pts',(94.209400296511,-1.08785505707932,1.40440398805559));
#22927=CARTESIAN_POINT('Ctrl Pts',(94.207565819018,-1.0665895317994,1.42062163221472));
#22928=CARTESIAN_POINT('Ctrl Pts',(94.1994189944927,-0.97151033826795,1.48979311437445));
#22929=CARTESIAN_POINT('Ctrl Pts',(94.1929165196412,-0.894073161718743,
1.53751250252177));
#22930=CARTESIAN_POINT('Ctrl Pts',(94.1790751612384,-0.724933105126678,
1.62463065929377));
#22931=CARTESIAN_POINT('Ctrl Pts',(94.1717385091288,-0.632860841533863,
1.66266065870763));
#22932=CARTESIAN_POINT('Ctrl Pts',(94.1618360132447,-0.501338220428661,
1.70446799208706));
#22933=CARTESIAN_POINT('Ctrl Pts',(94.159103355935,-0.46421365473568,1.71495111383151));
#22934=CARTESIAN_POINT('Ctrl Pts',(94.1555859666233,-0.414989972006551,
1.72713484271013));
#22935=CARTESIAN_POINT('Ctrl Pts',(94.1547496703116,-0.403175594999771,
1.72993089513585));
#22936=CARTESIAN_POINT('Ctrl Pts',(94.1533970134952,-0.383870142125925,
1.73429129995688));
#22937=CARTESIAN_POINT('Ctrl Pts',(94.1528767248285,-0.37639621702699,1.73592871183059));
#22938=CARTESIAN_POINT('Ctrl Pts',(94.1518465497956,-0.361496740912076,
1.73909218561173));
#22939=CARTESIAN_POINT('Ctrl Pts',(94.1513366301004,-0.354071556981567,
1.74061910282712));
#22940=CARTESIAN_POINT('Ctrl Pts',(94.1500388449784,-0.335052546802409,
1.74440343904303));
#22941=CARTESIAN_POINT('Ctrl Pts',(94.1492547100042,-0.32344533206813,1.74659288421936));
#22942=CARTESIAN_POINT('Ctrl Pts',(94.1459102440446,-0.273487489281059,
1.75550121107037));
#22943=CARTESIAN_POINT('Ctrl Pts',(94.1434065570145,-0.234940588370822,
1.76107448358309));
#22944=CARTESIAN_POINT('Ctrl Pts',(94.1360132952326,-0.118868961974354,
1.77397696013767));
#22945=CARTESIAN_POINT('Ctrl Pts',(94.1312450137954,-0.0410124122563852,
1.77748239804443));
#22946=CARTESIAN_POINT('Ctrl Pts',(94.1196087017441,0.148528879026554,1.7735517576253));
#22947=CARTESIAN_POINT('Ctrl Pts',(94.1127431696131,0.259750139340181,1.76070238192323));
#22948=CARTESIAN_POINT('Ctrl Pts',(94.1039620375275,0.393111428559367,1.73237811811083));
#22949=CARTESIAN_POINT('Ctrl Pts',(94.1023618566181,0.417090846235809,1.72676161371742));
#22950=CARTESIAN_POINT('Ctrl Pts',(94.0997137961818,0.456182855686057,1.71674363561967));
#22951=CARTESIAN_POINT('Ctrl Pts',(94.0986753269721,0.471367889458472,1.71263650389831));
#22952=CARTESIAN_POINT('Ctrl Pts',(94.096785279977,0.498729181589673,1.70484458349575));
#22953=CARTESIAN_POINT('Ctrl Pts',(94.0959360240724,0.510924333149826,1.70122960289306));
#22954=CARTESIAN_POINT('Ctrl Pts',(94.0940935758403,0.53716131431373,1.69314468279882));
#22955=CARTESIAN_POINT('Ctrl Pts',(94.0930989804083,0.551188360896928,1.6886303806519));
#22956=CARTESIAN_POINT('Ctrl Pts',(94.0902982139475,0.590297733114425,1.6755046655299));
#22957=CARTESIAN_POINT('Ctrl Pts',(94.0884794302712,0.615244844818676,1.66650560952092));
#22958=CARTESIAN_POINT('Ctrl Pts',(94.0804693826694,0.723115473339314,1.62484172722915));
#22959=CARTESIAN_POINT('Ctrl Pts',(94.0740955019575,0.803704434977019,1.58652503101406));
#22960=CARTESIAN_POINT('Ctrl Pts',(94.0606279868053,0.964542411749395,1.49464501365388));
#22961=CARTESIAN_POINT('Ctrl Pts',(94.0535384469619,1.04400664639059,1.44026251287449));
#22962=CARTESIAN_POINT('Ctrl Pts',(94.0435125864332,1.15218511719984,1.35255095345306));
#22963=CARTESIAN_POINT('Ctrl Pts',(94.0404463695849,1.1846924336517,1.324171107772));
#22964=CARTESIAN_POINT('Ctrl Pts',(94.0365790225439,1.22529120948223,1.28603392999653));
#22965=CARTESIAN_POINT('Ctrl Pts',(94.0357131195092,1.23435455506811,1.27733733687547));
#22966=CARTESIAN_POINT('Ctrl Pts',(94.0343247823576,1.24885424043248,1.26312591835201));
#22967=CARTESIAN_POINT('Ctrl Pts',(94.033798041286,1.25434791947277,1.25767058572045));
#22968=CARTESIAN_POINT('Ctrl Pts',(94.032766406138,1.26509582218615,1.24685722195689));
#22969=CARTESIAN_POINT('Ctrl Pts',(94.0322613727069,1.27035205677732,1.24150152099397));
#22970=CARTESIAN_POINT('Ctrl Pts',(94.0309925414292,1.28353883052675,1.22789377224332));
#22971=CARTESIAN_POINT('Ctrl Pts',(94.0302321473457,1.29142402201694,1.21959790829906));
#22972=CARTESIAN_POINT('Ctrl Pts',(94.0271397083271,1.32338960725514,1.18530983810032));
#22973=CARTESIAN_POINT('Ctrl Pts',(94.0248542374336,1.34677155586203,1.15867434406262));
#22974=CARTESIAN_POINT('Ctrl Pts',(94.0184116380934,1.41135837396323,1.08050128714177));
#22975=CARTESIAN_POINT('Ctrl Pts',(94.0143423418909,1.45051148641425,1.02734274289743));
#22976=CARTESIAN_POINT('Ctrl Pts',(94.0023456079645,1.55736036323134,0.8639446436584));
#22977=CARTESIAN_POINT('Ctrl Pts',(93.9944693107659,1.61607519881808,0.748377282910658));
#22978=CARTESIAN_POINT('Ctrl Pts',(93.9844457045107,1.67099695358711,0.602927308744723));
#22979=CARTESIAN_POINT('Ctrl Pts',(93.9827385154483,1.67971820255529,0.578185785918303));
#22980=CARTESIAN_POINT('Ctrl Pts',(93.9800380918145,1.69250697331467,0.539169833474381));
#22981=CARTESIAN_POINT('Ctrl Pts',(93.9790571772064,1.69694912515043,0.525021531269705));
#22982=CARTESIAN_POINT('Ctrl Pts',(93.9772244569097,1.7048695849922,0.498643544495678));
#22983=CARTESIAN_POINT('Ctrl Pts',(93.9763742497931,1.70839475732654,0.486428848790857));
#22984=CARTESIAN_POINT('Ctrl Pts',(93.9744703683221,1.71595596094587,0.45913278932863));
#22985=CARTESIAN_POINT('Ctrl Pts',(93.973414587813,1.71992484600809,0.444034092207501));
#22986=CARTESIAN_POINT('Ctrl Pts',(93.9702452912737,1.73117074183514,0.398836746340757));
#22987=CARTESIAN_POINT('Ctrl Pts',(93.9681132561072,1.73785993092249,0.368599428804067));
#22988=CARTESIAN_POINT('Ctrl Pts',(93.9630964330432,1.75157728904911,0.297873799108614));
#22989=CARTESIAN_POINT('Ctrl Pts',(93.9601947148737,1.75799738984498,0.257286882321925));
#22990=CARTESIAN_POINT('Ctrl Pts',(93.9513094686424,1.77315323233064,0.133879078515832));
#22991=CARTESIAN_POINT('Ctrl Pts',(93.9452264076527,1.7774785525948,0.0506361430331844));
#22992=CARTESIAN_POINT('Ctrl Pts',(93.9387739566831,1.77585943002973,-0.037579036994388));
#22993=CARTESIAN_POINT('Ctrl Pts',(93.9384095511236,1.77574701040699,-0.0425611044426868));
#22994=CARTESIAN_POINT('Ctrl Pts',(93.9380452419004,1.77561363825831,-0.0475422983361156));
#22995=CARTESIAN_POINT('Ctrl Pts',(93.79153079842,1.7756136390086,-0.0475422703142009));
#22996=CARTESIAN_POINT('Ctrl Pts',(93.7951001279053,1.776934385346,0.00178510077781863));
#22997=CARTESIAN_POINT('Ctrl Pts',(93.7986279292612,1.77619947883391,0.0511620355513193));
#22998=CARTESIAN_POINT('Ctrl Pts',(93.8030481184526,1.77261024993695,0.114522261575697));
#22999=CARTESIAN_POINT('Ctrl Pts',(93.8040216851538,1.77164638042591,0.128575194345392));
#23000=CARTESIAN_POINT('Ctrl Pts',(93.8055361665494,1.76987129544117,0.15061214357101));
#23001=CARTESIAN_POINT('Ctrl Pts',(93.8060829002402,1.76917299833563,0.158604314502194));
#23002=CARTESIAN_POINT('Ctrl Pts',(93.8071166449974,1.76774236346225,0.173790932308062));
#23003=CARTESIAN_POINT('Ctrl Pts',(93.8076041625932,1.76702021329073,0.180985964401413));
#23004=CARTESIAN_POINT('Ctrl Pts',(93.8087779001014,1.76516666704678,0.1983836380883));
#23005=CARTESIAN_POINT('Ctrl Pts',(93.8094616817121,1.76399070989842,0.208581442973571));
#23006=CARTESIAN_POINT('Ctrl Pts',(93.8119028513006,1.7594476584015,0.245187015983037));
#23007=CARTESIAN_POINT('Ctrl Pts',(93.8136347086749,1.75557524059647,0.27152990863758));
#23008=CARTESIAN_POINT('Ctrl Pts',(93.8180595208785,1.74402280435814,0.339465238934993));
#23009=CARTESIAN_POINT('Ctrl Pts',(93.8207171867516,1.73544689433007,0.38088939307791));
#23010=CARTESIAN_POINT('Ctrl Pts',(93.828377690126,1.70617817965795,0.500566599623081));
#23011=CARTESIAN_POINT('Ctrl Pts',(93.8332999765335,1.68160813585582,0.577759152340324));
#23012=CARTESIAN_POINT('Ctrl Pts',(93.8439103356994,1.61832881858997,0.737831319096879));
#23013=CARTESIAN_POINT('Ctrl Pts',(93.8496033183079,1.57831793249048,0.819934583248301));
#23014=CARTESIAN_POINT('Ctrl Pts',(93.8569583208778,1.5209413323599,0.917766519669438));
#23015=CARTESIAN_POINT('Ctrl Pts',(93.8584113577249,1.50934052661553,0.93672249030981));
#23016=CARTESIAN_POINT('Ctrl Pts',(93.8607845531922,1.48999031214843,0.96704811037777));
#23017=CARTESIAN_POINT('Ctrl Pts',(93.8616966430971,1.48245887022327,0.978554473786703));
#23018=CARTESIAN_POINT('Ctrl Pts',(93.8634645017353,1.46768517412862,1.00056334926166));
#23019=CARTESIAN_POINT('Ctrl Pts',(93.8643195170617,1.46046186628465,1.0110775977473));
#23020=CARTESIAN_POINT('Ctrl Pts',(93.8663277947901,1.44331841241669,1.03546456360478));
#23021=CARTESIAN_POINT('Ctrl Pts',(93.8674843711257,1.43331061953878,1.04927381295778));
#23022=CARTESIAN_POINT('Ctrl Pts',(93.871369080488,1.39926088745102,1.09486108613009));
#23023=CARTESIAN_POINT('Ctrl Pts',(93.874130672568,1.37435023564364,1.12597194470871));
#23024=CARTESIAN_POINT('Ctrl Pts',(93.881055981465,1.31019680618218,1.20078967825894));
#23025=CARTESIAN_POINT('Ctrl Pts',(93.8852609356911,1.26979416025413,1.24343604478015));
#23026=CARTESIAN_POINT('Ctrl Pts',(93.8977286388729,1.14543270153583,1.36231136470535));
#23027=CARTESIAN_POINT('Ctrl Pts',(93.9061144470148,1.05620323854568,1.43260002810284));
#23028=CARTESIAN_POINT('Ctrl Pts',(93.9168910441379,0.929728499158324,1.51394894381923));
#23029=CARTESIAN_POINT('Ctrl Pts',(93.9195131425905,0.89794894028685,1.53301162139284));
#23030=CARTESIAN_POINT('Ctrl Pts',(93.9229074179601,0.85519821914223,1.55686922931175));
#23031=CARTESIAN_POINT('Ctrl Pts',(93.9237272219086,0.844744052007549,1.56256625371961));
#23032=CARTESIAN_POINT('Ctrl Pts',(93.9250055828191,0.82822680827509,1.57135314324666));
#23033=CARTESIAN_POINT('Ctrl Pts',(93.9254683719418,0.822202137801622,1.57451389173938));
#23034=CARTESIAN_POINT('Ctrl Pts',(93.9264267841305,0.809627984207273,1.58101886921314));
#23035=CARTESIAN_POINT('Ctrl Pts',(93.9269219914552,0.80307566624127,1.58435716124668));
#23036=CARTESIAN_POINT('Ctrl Pts',(93.928148429081,0.786715607287767,1.59256475902223));
#23037=CARTESIAN_POINT('Ctrl Pts',(93.928876650081,0.776883001163696,1.59738435452997));
#23038=CARTESIAN_POINT('Ctrl Pts',(93.9316973292596,0.738364944915256,1.61582474439925));
#23039=CARTESIAN_POINT('Ctrl Pts',(93.9337526791903,0.709359084570396,1.62876713468873));
#23040=CARTESIAN_POINT('Ctrl Pts',(93.9393072948116,0.628930376417344,1.66209777837205));
#23041=CARTESIAN_POINT('Ctrl Pts',(93.9427447310023,0.5768764502547,1.68087383304231));
#23042=CARTESIAN_POINT('Ctrl Pts',(93.9547875890271,0.390278508504457,1.73848816636115));
#23043=CARTESIAN_POINT('Ctrl Pts',(93.9632476708782,0.252128709187763,1.76382727580857));
#23044=CARTESIAN_POINT('Ctrl Pts',(93.9739386976448,0.0860788704251266,
1.77435965566323));
#23045=CARTESIAN_POINT('Ctrl Pts',(93.9756518002809,0.0596850399432994,
1.77544342066861));
#23046=CARTESIAN_POINT('Ctrl Pts',(93.9784419853642,0.0171217143288013,
1.77624098129434));
#23047=CARTESIAN_POINT('Ctrl Pts',(93.9795076633116,0.000962604192458216,
1.77632323112394));
#23048=CARTESIAN_POINT('Ctrl Pts',(93.981419351571,-0.0278356676466562,
1.77607686704211));
#23049=CARTESIAN_POINT('Ctrl Pts',(93.9822626288065,-0.0404745851562134,
1.77583379171689));
#23050=CARTESIAN_POINT('Ctrl Pts',(93.9840616042502,-0.0672936444328707,
1.77503154797161));
#23051=CARTESIAN_POINT('Ctrl Pts',(93.9850183444686,-0.0814717671662096,
1.77443730845902));
#23052=CARTESIAN_POINT('Ctrl Pts',(93.987629098197,-0.119921299439404,1.77236401355179));
#23053=CARTESIAN_POINT('Ctrl Pts',(93.9892932365374,-0.14417114574734,1.77055637951881));
#23054=CARTESIAN_POINT('Ctrl Pts',(93.9930373361706,-0.198133422439832,
1.76541802088226));
#23055=CARTESIAN_POINT('Ctrl Pts',(93.9951245279484,-0.227813734626224,
1.76183380705522));
#23056=CARTESIAN_POINT('Ctrl Pts',(94.0020064016542,-0.324374436079653,
1.74769239432223));
#23057=CARTESIAN_POINT('Ctrl Pts',(94.0068831034637,-0.390738935228149,
1.73406141429018));
#23058=CARTESIAN_POINT('Ctrl Pts',(94.0193503432439,-0.556247636455101,
1.69008221509953));
#23059=CARTESIAN_POINT('Ctrl Pts',(94.026994284601,-0.653820697743124,1.65478362061564));
#23060=CARTESIAN_POINT('Ctrl Pts',(94.0367697288277,-0.777951948391084,
1.59717326568779));
#23061=CARTESIAN_POINT('Ctrl Pts',(94.0391185229558,-0.807742611733825,
1.58231598681615));
#23062=CARTESIAN_POINT('Ctrl Pts',(94.0422175355942,-0.847207640106647,
1.56122855573939));
#23063=CARTESIAN_POINT('Ctrl Pts',(94.0430059930102,-0.857262840544182,
1.55572999855696));
#23064=CARTESIAN_POINT('Ctrl Pts',(94.0442473189012,-0.873127108806972,
1.54685430590564));
#23065=CARTESIAN_POINT('Ctrl Pts',(94.0447040278569,-0.878971238317084,
1.54354098029815));
#23066=CARTESIAN_POINT('Ctrl Pts',(94.0456616317238,-0.891243343935174,
1.53649101571774));
#23067=CARTESIAN_POINT('Ctrl Pts',(94.0461620117057,-0.897666917981372,
1.53274702655251));
#23068=CARTESIAN_POINT('Ctrl Pts',(94.0474203684577,-0.913842578200213,
1.52318245146987));
#23069=CARTESIAN_POINT('Ctrl Pts',(94.0481749850471,-0.923562911254201,
1.51730834175438));
#23070=CARTESIAN_POINT('Ctrl Pts',(94.0512503075312,-0.963222456067497,
1.49281927218814));
#23071=CARTESIAN_POINT('Ctrl Pts',(94.0535248315128,-0.992662692539539,
1.47340695244934));
#23072=CARTESIAN_POINT('Ctrl Pts',(94.0599345840296,-1.07517503531732,1.41540318285753));
#23073=CARTESIAN_POINT('Ctrl Pts',(94.0639826484755,-1.12671492843033,1.37472985710406));
#23074=CARTESIAN_POINT('Ctrl Pts',(94.0760163600187,-1.27347719665078,1.24509961434019));
#23075=CARTESIAN_POINT('Ctrl Pts',(94.0839474661905,-1.36128145355664,1.14844501713842));
#23076=CARTESIAN_POINT('Ctrl Pts',(94.0940232074457,-1.45303593928849,1.0219734796882));
#23077=CARTESIAN_POINT('Ctrl Pts',(94.0957195603368,-1.46787292796113,1.00054594499747));
#23078=CARTESIAN_POINT('Ctrl Pts',(94.0984007307722,-1.49033478617992,0.966531154926721));
#23079=CARTESIAN_POINT('Ctrl Pts',(94.0993733655579,-1.49828413252358,0.954161875537906));
#23080=CARTESIAN_POINT('Ctrl Pts',(94.1011890951546,-1.51275023442366,0.931025855163851));
#23081=CARTESIAN_POINT('Ctrl Pts',(94.1020306049174,-1.51930793288489,0.920285719623472));
#23082=CARTESIAN_POINT('Ctrl Pts',(94.1039127653671,-1.5336465055089,0.896231139049658));
#23083=CARTESIAN_POINT('Ctrl Pts',(94.1049554542481,-1.5413691387209,0.882883350427976));
#23084=CARTESIAN_POINT('Ctrl Pts',(94.1080759892758,-1.56382181252274,0.842883533271501));
#23085=CARTESIAN_POINT('Ctrl Pts',(94.1101716969438,-1.57804068406961,0.815952640954332));
#23086=CARTESIAN_POINT('Ctrl Pts',(94.1210439991829,-1.64740550188712,0.675972541353107));
#23087=CARTESIAN_POINT('Ctrl Pts',(94.1302005745206,-1.69111464581896,0.557678276784016));
#23088=CARTESIAN_POINT('Ctrl Pts',(94.1457148620955,-1.74316211221659,0.352017368228739));
#23089=CARTESIAN_POINT('Ctrl Pts',(94.1520214378522,-1.75822269099445,0.266807217441393));
#23090=CARTESIAN_POINT('Ctrl Pts',(94.1593606225872,-1.76887433059878,0.16272377323222));
#23091=CARTESIAN_POINT('Ctrl Pts',(94.1606260255372,-1.77044914422218,0.144586707148865));
#23092=CARTESIAN_POINT('Ctrl Pts',(94.1624864399562,-1.77237554125064,0.117590392395109));
#23093=CARTESIAN_POINT('Ctrl Pts',(94.163092114422,-1.77294004511353,0.108748170059994));
#23094=CARTESIAN_POINT('Ctrl Pts',(94.164176593029,-1.77383771797021,0.0928128560022862));
#23095=CARTESIAN_POINT('Ctrl Pts',(94.164656633065,-1.77419454460256,0.0857216320530697));
#23096=CARTESIAN_POINT('Ctrl Pts',(94.1657382355763,-1.77490624882382,0.0696596089174864));
#23097=CARTESIAN_POINT('Ctrl Pts',(94.1663383967329,-1.77523565268846,0.060688049386925));
#23098=CARTESIAN_POINT('Ctrl Pts',(94.1681861506817,-1.77604505875409,0.0328987805694946));
#23099=CARTESIAN_POINT('Ctrl Pts',(94.1694218314036,-1.77629399169738,0.014074975118532));
#23100=CARTESIAN_POINT('Ctrl Pts',(94.1723362417095,-1.77617402467342,-0.0307849275125319));
#23101=CARTESIAN_POINT('Ctrl Pts',(94.1740030436563,-1.77553200855828,-0.0568164163390386));
#23102=CARTESIAN_POINT('Ctrl Pts',(94.1804817763263,-1.77076266237805,-0.158986852576733));
#23103=CARTESIAN_POINT('Ctrl Pts',(94.1851563792875,-1.76230713983039,-0.234845329123573));
#23104=CARTESIAN_POINT('Ctrl Pts',(94.1968509995233,-1.72906222918476,-0.422453601548267));
#23105=CARTESIAN_POINT('Ctrl Pts',(94.2038652132316,-1.69831305992961,-0.532777844206003));
#23106=CARTESIAN_POINT('Ctrl Pts',(94.2128035603766,-1.64836806490588,-0.662228512982705));
#23107=CARTESIAN_POINT('Ctrl Pts',(94.2143951616313,-1.63908094679585,-0.684892281594365));
#23108=CARTESIAN_POINT('Ctrl Pts',(94.2170265869908,-1.62311268248434,-0.721673691903877));
#23109=CARTESIAN_POINT('Ctrl Pts',(94.2180570756095,-1.61670850102209,-0.735908482348476));
#23110=CARTESIAN_POINT('Ctrl Pts',(94.2199306990669,-1.60479962043342,-0.761472817450772));
#23111=CARTESIAN_POINT('Ctrl Pts',(94.2207715305944,-1.59936037611383,-0.772831835991971));
#23112=CARTESIAN_POINT('Ctrl Pts',(94.2225932872729,-1.58737539432715,-0.797192121874985));
#23113=CARTESIAN_POINT('Ctrl Pts',(94.2235755619921,-1.58078975178258,-0.810172611451816));
#23114=CARTESIAN_POINT('Ctrl Pts',(94.2263336906443,-1.56196047538652,-0.846181850452954));
#23115=CARTESIAN_POINT('Ctrl Pts',(94.2281216997987,-1.54936850242923,-0.869023226657982));
#23116=CARTESIAN_POINT('Ctrl Pts',(94.2359229917443,-1.49280695684608,-0.966484463187603));
#23117=CARTESIAN_POINT('Ctrl Pts',(94.2421084162089,-1.44392116365872,-1.03810050837571));
#23118=CARTESIAN_POINT('Ctrl Pts',(94.2581282650563,-1.30660611156105,-1.2106995315271));
#23119=CARTESIAN_POINT('Ctrl Pts',(94.2680783984377,-1.21160243492819,-1.30576991082433));
#23120=CARTESIAN_POINT('Ctrl Pts',(94.278692807597,-1.09312175316951,-1.4001625643195));
#23121=CARTESIAN_POINT('Ctrl Pts',(94.279908373913,-1.07927203307594,-1.41086580156895));
#23122=CARTESIAN_POINT('Ctrl Pts',(94.281710327571,-1.05828459896727,-1.42659520595447));
#23123=CARTESIAN_POINT('Ctrl Pts',(94.2823064649139,-1.05126482115094,-1.43177598037084));
#23124=CARTESIAN_POINT('Ctrl Pts',(94.2833332810544,-1.03903547822782,-1.44066311313724));
#23125=CARTESIAN_POINT('Ctrl Pts',(94.2837655490933,-1.0338437983784,-1.4443932755476));
#23126=CARTESIAN_POINT('Ctrl Pts',(94.2847846872879,-1.02150089251405,-1.45316086406434));
#23127=CARTESIAN_POINT('Ctrl Pts',(94.2853698915786,-1.01433246163006,-1.45817359584425));
#23128=CARTESIAN_POINT('Ctrl Pts',(94.2871237602798,-0.992614842103307,
-1.47312261195568));
#23129=CARTESIAN_POINT('Ctrl Pts',(94.2882821884218,-0.977954084614268,
-1.48289592375008));
#23130=CARTESIAN_POINT('Ctrl Pts',(94.2940509198816,-0.903503194083136,
-1.53094266156814));
#23131=CARTESIAN_POINT('Ctrl Pts',(94.2984845150199,-0.841595962509255,
-1.56582945647219));
#23132=CARTESIAN_POINT('Ctrl Pts',(94.3108614411569,-0.661391893625565,
-1.65359566043891));
#23133=CARTESIAN_POINT('Ctrl Pts',(94.3186796817457,-0.53918478404979,-1.69737919369666));
#23134=CARTESIAN_POINT('Ctrl Pts',(94.3293390681498,-0.376219298444444,
-1.73636900249191));
#23135=CARTESIAN_POINT('Ctrl Pts',(94.3317952242991,-0.338858081628253,
-1.74404505191454));
#23136=CARTESIAN_POINT('Ctrl Pts',(94.3353011701874,-0.286028070785535,
-1.75313762786081));
#23137=CARTESIAN_POINT('Ctrl Pts',(94.3363193742529,-0.270742100845669,
-1.75556323991451));
#23138=CARTESIAN_POINT('Ctrl Pts',(94.3381942993764,-0.242713527250378,
-1.75963611172289));
#23139=CARTESIAN_POINT('Ctrl Pts',(94.3390490058336,-0.229980905755203,
-1.76134547155717));
#23140=CARTESIAN_POINT('Ctrl Pts',(94.3407973754078,-0.204033453615995,
-1.76454278383942));
#23141=CARTESIAN_POINT('Ctrl Pts',(94.3416912957212,-0.190818241230066,
-1.76602074401358));
#23142=CARTESIAN_POINT('Ctrl Pts',(94.3439433435283,-0.157662034001186,
-1.76935236682008));
#23143=CARTESIAN_POINT('Ctrl Pts',(94.3453072936736,-0.137704393111346,
-1.77101737927376));
#23144=CARTESIAN_POINT('Ctrl Pts',(94.3510767812486,-0.053830993602963,
-1.77658846035042));
#23145=CARTESIAN_POINT('Ctrl Pts',(94.355577273278,0.0102367710365958,-1.77737385486933));
#23146=CARTESIAN_POINT('Ctrl Pts',(94.3703551594012,0.216494383810738,-1.76875015293116));
#23147=CARTESIAN_POINT('Ctrl Pts',(94.3809506457999,0.357540539793017,-1.7457109125371));
#23148=CARTESIAN_POINT('Ctrl Pts',(94.3937151254229,0.52878488348619,-1.69609507560905));
#23149=CARTESIAN_POINT('Ctrl Pts',(94.3962529888944,0.562946730654938,-1.68506478965365));
#23150=CARTESIAN_POINT('Ctrl Pts',(94.3995567543169,0.60784249456448,-1.66905068142524));
#23151=CARTESIAN_POINT('Ctrl Pts',(94.4003672915372,0.618892347483565,-1.66498497183998));
#23152=CARTESIAN_POINT('Ctrl Pts',(94.4016346862455,0.636238535227415,-1.65840601964273));
#23153=CARTESIAN_POINT('Ctrl Pts',(94.4020956588359,0.642562070255365,-1.65596618005126));
#23154=CARTESIAN_POINT('Ctrl Pts',(94.4030536815524,0.655737487206398,-1.65079581111914));
#23155=CARTESIAN_POINT('Ctrl Pts',(94.4035502873442,0.662586578068556,-1.64805870387988));
#23156=CARTESIAN_POINT('Ctrl Pts',(94.4047855405379,0.679665399435131,-1.64110980368981));
#23157=CARTESIAN_POINT('Ctrl Pts',(94.4055210822748,0.689873430413712,-1.63684486392991));
#23158=CARTESIAN_POINT('Ctrl Pts',(94.408409929064,0.730082635461765,-1.61960237270646));
#23159=CARTESIAN_POINT('Ctrl Pts',(94.4105238008715,0.75976494654413,-1.60589228894177));
#23160=CARTESIAN_POINT('Ctrl Pts',(94.4162986603034,0.840944945395216,-1.5656405459852));
#23161=CARTESIAN_POINT('Ctrl Pts',(94.4198917248216,0.891550042316297,-1.53738679760621));
#23162=CARTESIAN_POINT('Ctrl Pts',(94.4323339885751,1.06288894054865,-1.4304143849655));
#23163=CARTESIAN_POINT('Ctrl Pts',(94.441054845466,1.17534282806859,-1.33954600846397));
#23164=CARTESIAN_POINT('Ctrl Pts',(94.4519422362075,1.29258283149604,-1.2185606803535));
#23165=CARTESIAN_POINT('Ctrl Pts',(94.4535345871111,1.30921412411718,-1.20067430681051));
#23166=CARTESIAN_POINT('Ctrl Pts',(94.4560872195412,1.33502222955283,-1.17174467117599));
#23167=CARTESIAN_POINT('Ctrl Pts',(94.4570372016982,1.34444338902761,-1.16092285754837));
#23168=CARTESIAN_POINT('Ctrl Pts',(94.4587487780797,1.36108341582007,-1.14133471159695));
#23169=CARTESIAN_POINT('Ctrl Pts',(94.4595082920185,1.36835134784434,-1.13261095140028));
#23170=CARTESIAN_POINT('Ctrl Pts',(94.4612985729268,1.3852080404834,-1.11197863827282));
#23171=CARTESIAN_POINT('Ctrl Pts',(94.4623320581621,1.39472754428421,-1.10001493584488));
#23172=CARTESIAN_POINT('Ctrl Pts',(94.4653958477792,1.42232068283326,-1.06440301540969));
#23173=CARTESIAN_POINT('Ctrl Pts',(94.4674430511485,1.4399549523948,-1.04042272801189));
#23174=CARTESIAN_POINT('Ctrl Pts',(94.474467851913,1.49773733161957,-0.957561861929908));
#23175=CARTESIAN_POINT('Ctrl Pts',(94.4795479971308,1.53493812033648,-0.896718831366329));
#23176=CARTESIAN_POINT('Ctrl Pts',(94.4923147950042,1.61771367677764,-0.74102002535935));
#23177=CARTESIAN_POINT('Ctrl Pts',(94.5000769950445,1.65871199671132,-0.644035723222692));
#23178=CARTESIAN_POINT('Ctrl Pts',(94.5109847202854,1.70502685167466,-0.500076256215709));
#23179=CARTESIAN_POINT('Ctrl Pts',(94.514270935289,1.71744200492499,-0.455616691109116));
#23180=CARTESIAN_POINT('Ctrl Pts',(94.5183643008631,1.73106738122804,-0.398287690991768));
#23181=CARTESIAN_POINT('Ctrl Pts',(94.5192456907559,1.73388809172322,-0.385823110128413));
#23182=CARTESIAN_POINT('Ctrl Pts',(94.5206493463459,1.73820094271484,-0.365761472941479));
#23183=CARTESIAN_POINT('Ctrl Pts',(94.5211761528115,1.7397783109951,-0.358183481934652));
#23184=CARTESIAN_POINT('Ctrl Pts',(94.5221990240581,1.74276093592466,-0.343369638293446));
#23185=CARTESIAN_POINT('Ctrl Pts',(94.522695311691,1.74417076744543,-0.336134980253873));
#23186=CARTESIAN_POINT('Ctrl Pts',(94.5236944786626,1.74693220727491,-0.32147911596434));
#23187=CARTESIAN_POINT('Ctrl Pts',(94.524197237557,1.74828166772825,-0.314057596849312));
#23188=CARTESIAN_POINT('Ctrl Pts',(94.525411204536,1.75144109941514,-0.296030218846623));
#23189=CARTESIAN_POINT('Ctrl Pts',(94.5261198851904,1.75320209134581,-0.28541593402213));
#23190=CARTESIAN_POINT('Ctrl Pts',(94.5318074522998,1.76664475776472,-0.199566997261982));
#23191=CARTESIAN_POINT('Ctrl Pts',(94.5365633824408,1.77357534152074,-0.123668924889746));
#23192=CARTESIAN_POINT('Ctrl Pts',(94.5412649413994,1.77561364082573,-0.0475422024479729));
#23193=CARTESIAN_POINT('Origin',(88.3562164250559,0.,0.));
#23194=CARTESIAN_POINT('',(95.4381488386039,1.77561363782275,-0.0475423146035081));
#23195=CARTESIAN_POINT('',(95.2889037169481,1.77561363837214,-0.0475422940850334));
#23196=CARTESIAN_POINT('',(88.3562164250559,1.77561363837197,-0.0475422940912398));
#23197=CARTESIAN_POINT('Ctrl Pts',(95.4381488398588,1.77561363782069,-0.0475423146804766));
#23198=CARTESIAN_POINT('Ctrl Pts',(95.4371673493555,1.77518568041986,-0.0635256971142646));
#23199=CARTESIAN_POINT('Ctrl Pts',(95.4361859452281,1.77454179510398,-0.0795075586954785));
#23200=CARTESIAN_POINT('Ctrl Pts',(95.4286895757639,1.76798043142665,-0.201390030257114));
#23201=CARTESIAN_POINT('Ctrl Pts',(95.4221357747288,1.75280626594391,-0.306560285918419));
#23202=CARTESIAN_POINT('Ctrl Pts',(95.4136906852217,1.72266583260142,-0.43369635086399));
#23203=CARTESIAN_POINT('Ctrl Pts',(95.412085225413,1.71648992989322,-0.457528490473432));
#23204=CARTESIAN_POINT('Ctrl Pts',(95.4095192272436,1.70593506054631,-0.49503067106221));
#23205=CARTESIAN_POINT('Ctrl Pts',(95.4085692527349,1.70188212861389,-0.508789736578343));
#23206=CARTESIAN_POINT('Ctrl Pts',(95.4067632719889,1.69390719590134,-0.534701323316748));
#23207=CARTESIAN_POINT('Ctrl Pts',(95.4059084524313,1.6900198952807,-0.546863632288354));
#23208=CARTESIAN_POINT('Ctrl Pts',(95.4039514683984,1.68086779615735,-0.574468165148865));
#23209=CARTESIAN_POINT('Ctrl Pts',(95.402846645943,1.67552075057792,-0.589881686674298));
#23210=CARTESIAN_POINT('Ctrl Pts',(95.3999171180912,1.6608754492379,-0.63029202402014));
#23211=CARTESIAN_POINT('Ctrl Pts',(95.3980809603956,1.65122552306115,-0.655156036148417));
#23212=CARTESIAN_POINT('Ctrl Pts',(95.3865169487597,1.5875710967022,-0.808817955858918));
#23213=CARTESIAN_POINT('Ctrl Pts',(95.3762999014666,1.51909945304612,-0.931070379372612));
#23214=CARTESIAN_POINT('Ctrl Pts',(95.3606835981856,1.39343576093228,-1.10404017970042));
#23215=CARTESIAN_POINT('Ctrl Pts',(95.3552972034587,1.34610869587555,-1.16127576580758));
#23216=CARTESIAN_POINT('Ctrl Pts',(95.3488288491492,1.28299642352949,-1.22853957113195));
#23217=CARTESIAN_POINT('Ctrl Pts',(95.347575452205,1.27045634253153,-1.24150313935822));
#23218=CARTESIAN_POINT('Ctrl Pts',(95.3457255077907,1.25145014069643,-1.26056156399679));
#23219=CARTESIAN_POINT('Ctrl Pts',(95.3451185600749,1.24513264638749,-1.2668021205742));
#23220=CARTESIAN_POINT('Ctrl Pts',(95.3440763856211,1.23413857505972,-1.27750059661218));
#23221=CARTESIAN_POINT('Ctrl Pts',(95.3436394845621,1.2294842032969,-1.28198065284727));
#23222=CARTESIAN_POINT('Ctrl Pts',(95.3426132321228,1.21844398021522,-1.29249196382069));
#23223=CARTESIAN_POINT('Ctrl Pts',(95.3420255357341,1.21203771329877,-1.2985013666496));
#23224=CARTESIAN_POINT('Ctrl Pts',(95.3403105965251,1.19310624920436,-1.31599785640673));
#23225=CARTESIAN_POINT('Ctrl Pts',(95.33919262212,1.18046007286718,-1.32735336225359));
#23226=CARTESIAN_POINT('Ctrl Pts',(95.3308679771558,1.08417677787222,-1.4113453066066));
#23227=CARTESIAN_POINT('Ctrl Pts',(95.3241108295041,0.994060706740887,-1.47620620847798));
#23228=CARTESIAN_POINT('Ctrl Pts',(95.3152906131993,0.870110629089963,-1.54888764775307));
#23229=CARTESIAN_POINT('Ctrl Pts',(95.3132708506961,0.841287212199349,-1.56473040189169));
#23230=CARTESIAN_POINT('Ctrl Pts',(95.3077199227652,0.761360968934005,-1.60581463858947));
#23231=CARTESIAN_POINT('Ctrl Pts',(95.3041682495723,0.709459670634261,-1.6294101537994));
#23232=CARTESIAN_POINT('Ctrl Pts',(95.2980575322972,0.620178695072255,-1.66492398051627));
#23233=CARTESIAN_POINT('Ctrl Pts',(95.2955386072899,0.583375197136572,-1.67817355998439));
#23234=CARTESIAN_POINT('Ctrl Pts',(95.2918653442918,0.529955168111838,-1.6954355871143));
#23235=CARTESIAN_POINT('Ctrl Pts',(95.2907433566947,0.513669833561855,-1.70044040733465));
#23236=CARTESIAN_POINT('Ctrl Pts',(95.2887611114122,0.484971922091875,-1.70881000125862));
#23237=CARTESIAN_POINT('Ctrl Pts',(95.2879042108289,0.472589920062627,-1.71227571908705));
#23238=CARTESIAN_POINT('Ctrl Pts',(95.2861066928904,0.446673244280947,-1.7192272658083));
#23239=CARTESIAN_POINT('Ctrl Pts',(95.2851653403585,0.43313291846677,-1.72268837406661));
#23240=CARTESIAN_POINT('Ctrl Pts',(95.2826705018581,0.397341387506327,-1.7313885798578));
#23241=CARTESIAN_POINT('Ctrl Pts',(95.2811085177059,0.375028081133695,-1.73635838637605));
#23242=CARTESIAN_POINT('Ctrl Pts',(95.272573753399,0.253673389488195,-1.76093930008252));
#23243=CARTESIAN_POINT('Ctrl Pts',(95.2653503297794,0.153208476465598,-1.77250627066225));
#23244=CARTESIAN_POINT('Ctrl Pts',(95.2524947111216,-0.0232766188042014,
-1.777706985077));
#23245=CARTESIAN_POINT('Ctrl Pts',(95.2469347538782,-0.0989381650435437,
-1.77510427009905));
#23246=CARTESIAN_POINT('Ctrl Pts',(95.2372981268782,-0.231157724342564,
-1.76207419550361));
#23247=CARTESIAN_POINT('Ctrl Pts',(95.2331963121733,-0.287813675324886,
-1.75371149143344));
#23248=CARTESIAN_POINT('Ctrl Pts',(95.2282984974795,-0.356926834026268,
-1.74006944161283));
#23249=CARTESIAN_POINT('Ctrl Pts',(95.2273871231394,-0.369853145243995,
-1.73736786649673));
#23250=CARTESIAN_POINT('Ctrl Pts',(95.2259440168215,-0.390445251720871,
-1.73282390647435));
#23251=CARTESIAN_POINT('Ctrl Pts',(95.2254073726865,-0.398130703375255,
-1.73107427182585));
#23252=CARTESIAN_POINT('Ctrl Pts',(95.2243777491388,-0.412935198287473,
-1.72760013670458));
#23253=CARTESIAN_POINT('Ctrl Pts',(95.2238844162702,-0.420055584077246,
-1.72588267819068));
#23254=CARTESIAN_POINT('Ctrl Pts',(95.2226628087831,-0.437748554545267,
-1.72149909884819));
#23255=CARTESIAN_POINT('Ctrl Pts',(95.2219375190404,-0.448307829774046,
-1.71877952312162));
#23256=CARTESIAN_POINT('Ctrl Pts',(95.2193284152843,-0.486459698973201,
-1.70857786291976));
#23257=CARTESIAN_POINT('Ctrl Pts',(95.2174738067635,-0.513897230877726,
-1.70052674397468));
#23258=CARTESIAN_POINT('Ctrl Pts',(95.2087784569228,-0.643299296123917,
-1.65913727985531));
#23259=CARTESIAN_POINT('Ctrl Pts',(95.2022685206178,-0.742307887420377,
-1.61726742379149));
#23260=CARTESIAN_POINT('Ctrl Pts',(95.1914301637065,-0.897823080502049,
-1.53419108528537));
#23261=CARTESIAN_POINT('Ctrl Pts',(95.1871635416619,-0.956755050066244,
-1.49814797876201));
#23262=CARTESIAN_POINT('Ctrl Pts',(95.1808766824735,-1.03832904654075,-1.44147684478382));
#23263=CARTESIAN_POINT('Ctrl Pts',(95.1789401966896,-1.06277296510262,-1.42355055125931));
#23264=CARTESIAN_POINT('Ctrl Pts',(95.1753900523547,-1.10622005712269,-1.38994511258567));
#23265=CARTESIAN_POINT('Ctrl Pts',(95.1737844180664,-1.12537867034144,-1.37447916773796));
#23266=CARTESIAN_POINT('Ctrl Pts',(95.1712182059507,-1.15518037168218,-1.34938064361897));
#23267=CARTESIAN_POINT('Ctrl Pts',(95.1702681950715,-1.16603921285925,-1.34000833811395));
#23268=CARTESIAN_POINT('Ctrl Pts',(95.1684621854115,-1.18634719608626,-1.32204667891708));
#23269=CARTESIAN_POINT('Ctrl Pts',(95.1676073738127,-1.19581958962775,-1.31348490103295));
#23270=CARTESIAN_POINT('Ctrl Pts',(95.1656504647123,-1.21718236025994,-1.29375318013663));
#23271=CARTESIAN_POINT('Ctrl Pts',(95.1645457099933,-1.2290126558104,-1.28252019479913));
#23272=CARTESIAN_POINT('Ctrl Pts',(95.1610614953316,-1.26559593827056,-1.24681298083359));
#23273=CARTESIAN_POINT('Ctrl Pts',(95.15865759349,-1.28978395456291,-1.2217744241541));
#23274=CARTESIAN_POINT('Ctrl Pts',(95.1468741443294,-1.40325543831654,-1.09718612430613));
#23275=CARTESIAN_POINT('Ctrl Pts',(95.1370764576979,-1.48182889672163,-0.988491527100039));
#23276=CARTESIAN_POINT('Ctrl Pts',(95.1220377431135,-1.58294661753013,-0.809055304563493));
#23277=CARTESIAN_POINT('Ctrl Pts',(95.1167940145574,-1.61456416910075,-0.74395901525983));
#23278=CARTESIAN_POINT('Ctrl Pts',(95.1104747571104,-1.64892543675146,-0.660626160949176));
#23279=CARTESIAN_POINT('Ctrl Pts',(95.1092357826179,-1.65547451529085,-0.64403898209159));
#23280=CARTESIAN_POINT('Ctrl Pts',(95.1074027617619,-1.66489532664284,-0.619084619121653));
#23281=CARTESIAN_POINT('Ctrl Pts',(95.1067985800756,-1.66795595490535,-0.610790598500431));
#23282=CARTESIAN_POINT('Ctrl Pts',(95.1057592938277,-1.67314528261916,-0.596398055070963));
#23283=CARTESIAN_POINT('Ctrl Pts',(95.1053225464353,-1.67530277300227,-0.590310426058524));
#23284=CARTESIAN_POINT('Ctrl Pts',(95.10429396303,-1.68032840724935,-0.575880472599933));
#23285=CARTESIAN_POINT('Ctrl Pts',(95.1037038138373,-1.68316767180902,-0.567528388533941));
#23286=CARTESIAN_POINT('Ctrl Pts',(95.1019375237214,-1.6915268381239,-0.542324134058072));
#23287=CARTESIAN_POINT('Ctrl Pts',(95.1007717341914,-1.69685690947472,-0.525409552605657));
#23288=CARTESIAN_POINT('Ctrl Pts',(95.0929682560156,-1.73117212989926,-0.410538918989828));
#23289=CARTESIAN_POINT('Ctrl Pts',(95.0867074481429,-1.75191715264279,-0.31030759736876));
#23290=CARTESIAN_POINT('Ctrl Pts',(95.0778737458339,-1.76883750564417,-0.167391252180866));
#23291=CARTESIAN_POINT('Ctrl Pts',(95.0753140629568,-1.7722821364723,-0.125785145551214));
#23292=CARTESIAN_POINT('Ctrl Pts',(95.0685917547937,-1.77743291750523,-0.0171151289799343));
#23293=CARTESIAN_POINT('Ctrl Pts',(95.0644026470968,-1.77681196856192,0.0499871792206389));
#23294=CARTESIAN_POINT('Ctrl Pts',(95.0580791121454,-1.77031852771257,0.148447213957664));
#23295=CARTESIAN_POINT('Ctrl Pts',(95.0560300720526,-1.76739498630451,0.17994174175725));
#23296=CARTESIAN_POINT('Ctrl Pts',(95.0529224883144,-1.76176019168303,0.226964113105994));
#23297=CARTESIAN_POINT('Ctrl Pts',(95.0518836669746,-1.75968042886069,0.242562246299189));
#23298=CARTESIAN_POINT('Ctrl Pts',(95.0499932489024,-1.75554525894066,0.270715168917963));
#23299=CARTESIAN_POINT('Ctrl Pts',(95.0491439784046,-1.75356167329921,0.283279548020821));
#23300=CARTESIAN_POINT('Ctrl Pts',(95.0473018064264,-1.7489899892575,0.310346722133862));
#23301=CARTESIAN_POINT('Ctrl Pts',(95.0463075053272,-1.74635608218016,0.324840702310841));
#23302=CARTESIAN_POINT('Ctrl Pts',(95.0435574125313,-1.73861836309575,0.364602109211037));
#23303=CARTESIAN_POINT('Ctrl Pts',(95.0417900166289,-1.73314449965041,0.389792935171712));
#23304=CARTESIAN_POINT('Ctrl Pts',(95.0291919330397,-1.69064359333954,0.566732903912166));
#23305=CARTESIAN_POINT('Ctrl Pts',(95.0177192469712,-1.63429307894147,0.713112327410821));
#23306=CARTESIAN_POINT('Ctrl Pts',(95.0011850257931,-1.52570813381402,0.912293765463015));
#23307=CARTESIAN_POINT('Ctrl Pts',(94.9960788583705,-1.48817670967008,0.97231552266737));
#23308=CARTESIAN_POINT('Ctrl Pts',(94.9901925835517,-1.43914672742977,1.04120691544465));
#23309=CARTESIAN_POINT('Ctrl Pts',(94.9892375413963,-1.43099993238571,1.05237558269419));
#23310=CARTESIAN_POINT('Ctrl Pts',(94.9877419284562,-1.41792433995297,1.06986862620894));
#23311=CARTESIAN_POINT('Ctrl Pts',(94.9871958371664,-1.41308188664874,1.07625642818078));
#23312=CARTESIAN_POINT('Ctrl Pts',(94.9861609294346,-1.40377116982851,1.08836725256927));
#23313=CARTESIAN_POINT('Ctrl Pts',(94.9856716259847,-1.39931084979218,1.09409593783311));
#23314=CARTESIAN_POINT('Ctrl Pts',(94.9844779740392,-1.38828992691172,1.10807319971657));
#23315=CARTESIAN_POINT('Ctrl Pts',(94.9837763029032,-1.38169066719397,1.11629120345719));
#23316=CARTESIAN_POINT('Ctrl Pts',(94.9817446898492,-1.36224398336196,1.14007131244078));
#23317=CARTESIAN_POINT('Ctrl Pts',(94.9804272147335,-1.34920360346218,1.15547435513978));
#23318=CARTESIAN_POINT('Ctrl Pts',(94.9707807858997,-1.25079024058236,1.267779834886));
#23319=CARTESIAN_POINT('Ctrl Pts',(94.9630093783366,-1.15532892641939,1.35534688537089));
#23320=CARTESIAN_POINT('Ctrl Pts',(94.951279670803,-1.00194349411806,1.46796047754011));
#23321=CARTESIAN_POINT('Ctrl Pts',(94.9474820629408,-0.950851815255546,
1.50155877336549));
#23322=CARTESIAN_POINT('Ctrl Pts',(94.9418155820051,-0.873845596467484,
1.54669015914483));
#23323=CARTESIAN_POINT('Ctrl Pts',(94.9400121966892,-0.849223956355684,
1.56034455138024));
#23324=CARTESIAN_POINT('Ctrl Pts',(94.9366830482413,-0.803683841019369,
1.58420246710241));
#23325=CARTESIAN_POINT('Ctrl Pts',(94.9351638030877,-0.782869245339488,
1.59459111866113));
#23326=CARTESIAN_POINT('Ctrl Pts',(94.9327035142906,-0.749156372829304,
1.61059817305142));
#23327=CARTESIAN_POINT('Ctrl Pts',(94.9317715514774,-0.736384502070001,
1.6164775259447));
#23328=CARTESIAN_POINT('Ctrl Pts',(94.9299789232367,-0.711824923907548,
1.62743172273709));
#23329=CARTESIAN_POINT('Ctrl Pts',(94.9291191881015,-0.700049335813447,
1.63253166797313));
#23330=CARTESIAN_POINT('Ctrl Pts',(94.9271394605597,-0.672947568246527,
1.64392216153924));
#23331=CARTESIAN_POINT('Ctrl Pts',(94.9260166366948,-0.657586773182371,
1.65012669393636));
#23332=CARTESIAN_POINT('Ctrl Pts',(94.9223396594687,-0.607333137269243,
1.66961203095749));
#23333=CARTESIAN_POINT('Ctrl Pts',(94.9197565978034,-0.572109983229449,
1.68200703867904));
#23334=CARTESIAN_POINT('Ctrl Pts',(94.9079552575104,-0.411628399259981,
1.73285639979874));
#23335=CARTESIAN_POINT('Ctrl Pts',(94.8983488517735,-0.282752252931157,
1.75848530785277));
#23336=CARTESIAN_POINT('Ctrl Pts',(94.8849250549699,-0.0995456483039938,
1.77424735036882));
#23337=CARTESIAN_POINT('Ctrl Pts',(94.8810826290418,-0.0466558431728965,
1.77642531440982));
#23338=CARTESIAN_POINT('Ctrl Pts',(94.8758082839818,0.0273778155928267,
1.77616460167959));
#23339=CARTESIAN_POINT('Ctrl Pts',(94.874315572671,0.0484985309680788,1.77571343770735));
#23340=CARTESIAN_POINT('Ctrl Pts',(94.8717122731435,0.0857089449389605,
1.77425412688575));
#23341=CARTESIAN_POINT('Ctrl Pts',(94.8705951424533,0.101802150352386,1.77340353499224));
#23342=CARTESIAN_POINT('Ctrl Pts',(94.8689059522415,0.126361207220014,1.77177005243482));
#23343=CARTESIAN_POINT('Ctrl Pts',(94.868325878031,0.134836238578159,1.77114524240381));
#23344=CARTESIAN_POINT('Ctrl Pts',(94.867259981052,0.150491967884848,1.76987801747836));
#23345=CARTESIAN_POINT('Ctrl Pts',(94.8667732932794,0.157673428877371,1.76925270146217));
#23346=CARTESIAN_POINT('Ctrl Pts',(94.865651562348,0.174299328095295,1.76770298628976));
#23347=CARTESIAN_POINT('Ctrl Pts',(94.865018285955,0.183740424727292,1.76674660604242));
#23348=CARTESIAN_POINT('Ctrl Pts',(94.8629324881069,0.21499912065253,1.76332682518299));
#23349=CARTESIAN_POINT('Ctrl Pts',(94.8614968053256,0.236779639654297,1.76053447082646));
#23350=CARTESIAN_POINT('Ctrl Pts',(94.8527390632201,0.370827037566415,1.7408161429651));
#23351=CARTESIAN_POINT('Ctrl Pts',(94.8458471554891,0.481320864256407,1.71356059277393));
#23352=CARTESIAN_POINT('Ctrl Pts',(94.833366047352,0.672993875978803,1.64625910565092));
#23353=CARTESIAN_POINT('Ctrl Pts',(94.8278284177559,0.755146664504372,1.61023013540792));
#23354=CARTESIAN_POINT('Ctrl Pts',(94.8200076135586,0.863001729550939,1.55285362419956));
#23355=CARTESIAN_POINT('Ctrl Pts',(94.8178976331551,0.89134805181674,1.53675788581653));
#23356=CARTESIAN_POINT('Ctrl Pts',(94.8147161836586,0.932852470792316,1.51165592143452));
#23357=CARTESIAN_POINT('Ctrl Pts',(94.813665901402,0.946359035998366,1.50323714183039));
#23358=CARTESIAN_POINT('Ctrl Pts',(94.8117710409134,0.97036583562552,1.48782168372529));
#23359=CARTESIAN_POINT('Ctrl Pts',(94.8109290072689,0.980908212262696,1.48089239396712));
#23360=CARTESIAN_POINT('Ctrl Pts',(94.8091061685265,1.00345469925942,1.46572666145408));
#23361=CARTESIAN_POINT('Ctrl Pts',(94.8081240270271,1.01543308136226,1.45745381224456));
#23362=CARTESIAN_POINT('Ctrl Pts',(94.8054415087653,1.04768237545668,1.43459034479831));
#23363=CARTESIAN_POINT('Ctrl Pts',(94.8037304481028,1.06774875663906,1.41971838730255));
#23364=CARTESIAN_POINT('Ctrl Pts',(94.7922848369348,1.19860504596151,1.31839219500686));
#23365=CARTESIAN_POINT('Ctrl Pts',(94.7820407735927,1.29909441720299,1.21948811449991));
#23366=CARTESIAN_POINT('Ctrl Pts',(94.7674146906,1.42410518327764,1.06326908561091));
#23367=CARTESIAN_POINT('Ctrl Pts',(94.7630708283233,1.45898217969909,1.0148834998749));
#23368=CARTESIAN_POINT('Ctrl Pts',(94.7564345086485,1.5094665079192,0.936848885948652));
#23369=CARTESIAN_POINT('Ctrl Pts',(94.7540834939636,1.52678122949233,0.908358073211197));
#23370=CARTESIAN_POINT('Ctrl Pts',(94.7510008735257,1.54883263863395,0.869659173160387));
#23371=CARTESIAN_POINT('Ctrl Pts',(94.7502304010801,1.55428812154426,0.85987096217953));
#23372=CARTESIAN_POINT('Ctrl Pts',(94.748956687236,1.56321869611005,0.843485006820129));
#23373=CARTESIAN_POINT('Ctrl Pts',(94.7484503191297,1.5667454694961,0.83691593964364));
#23374=CARTESIAN_POINT('Ctrl Pts',(94.747484178333,1.57343084231696,0.824273198811469));
#23375=CARTESIAN_POINT('Ctrl Pts',(94.7470239780714,1.57659584239097,0.818203199452427));
#23376=CARTESIAN_POINT('Ctrl Pts',(94.7457701592087,1.58516256159992,0.801539219495063));
#23377=CARTESIAN_POINT('Ctrl Pts',(94.7449808330366,1.59049323025127,0.790908825815355));
#23378=CARTESIAN_POINT('Ctrl Pts',(94.7418039713718,1.61167083750602,0.747596382175172));
#23379=CARTESIAN_POINT('Ctrl Pts',(94.7394648128184,1.62662150386868,0.714483127974592));
#23380=CARTESIAN_POINT('Ctrl Pts',(94.7299363124912,1.68420417403958,0.57575111017351));
#23381=CARTESIAN_POINT('Ctrl Pts',(94.7230628628197,1.71764776153717,0.466608138897889));
#23382=CARTESIAN_POINT('Ctrl Pts',(94.7116571116216,1.75458779890793,0.285510854090841));
#23383=CARTESIAN_POINT('Ctrl Pts',(94.7072338745856,1.76458718397845,0.215233541031594));
#23384=CARTESIAN_POINT('Ctrl Pts',(94.7006555627475,1.77294188471233,0.112910995989636));
#23385=CARTESIAN_POINT('Ctrl Pts',(94.6985990062708,1.77467650086268,0.0812092230829106));
#23386=CARTESIAN_POINT('Ctrl Pts',(94.6954823038842,1.77599967523665,0.0337273940316071));
#23387=CARTESIAN_POINT('Ctrl Pts',(94.6944420581689,1.77622898703791,0.0179705997162901));
#23388=CARTESIAN_POINT('Ctrl Pts',(94.692550137101,1.77626447216838,-0.0105080252660238));
#23389=CARTESIAN_POINT('Ctrl Pts',(94.6917008055914,1.77614366013113,-0.0232288134528812));
#23390=CARTESIAN_POINT('Ctrl Pts',(94.6905877131099,1.77580798056828,-0.0398123924314369));
#23391=CARTESIAN_POINT('Ctrl Pts',(94.6903278697093,1.77571711781477,-0.0436775350756413));
#23392=CARTESIAN_POINT('Ctrl Pts',(94.6900676319114,1.77561363837047,-0.0475422941472846));
#23393=CARTESIAN_POINT('Ctrl Pts',(94.5412649413993,1.77561364082569,-0.0475422024493503));
#23394=CARTESIAN_POINT('Ctrl Pts',(94.5502559495098,1.77951157462697,0.098038441105544));
#23395=CARTESIAN_POINT('Ctrl Pts',(94.5590380957431,1.76549338159589,0.243522831115066));
#23396=CARTESIAN_POINT('Ctrl Pts',(94.5696946412978,1.72953923387427,0.405162651961136));
#23397=CARTESIAN_POINT('Ctrl Pts',(94.5709887792827,1.72487570912236,0.424577995570075));
#23398=CARTESIAN_POINT('Ctrl Pts',(94.5734554249558,1.71543901027195,0.461139564574982));
#23399=CARTESIAN_POINT('Ctrl Pts',(94.5746257052108,1.71073347462111,0.478300780756946));
#23400=CARTESIAN_POINT('Ctrl Pts',(94.5766571541859,1.70218030655673,0.507751936600956));
#23401=CARTESIAN_POINT('Ctrl Pts',(94.5775142851384,1.69845532226753,0.520076271800486));
#23402=CARTESIAN_POINT('Ctrl Pts',(94.5791707182688,1.69103671048592,0.543691090814504));
#23403=CARTESIAN_POINT('Ctrl Pts',(94.5799693212022,1.68736314076384,0.554987186979495));
#23404=CARTESIAN_POINT('Ctrl Pts',(94.5820904277551,1.6773531555736,0.584749156719975));
#23405=CARTESIAN_POINT('Ctrl Pts',(94.5834191879829,1.67082527805208,0.603148424399207));
#23406=CARTESIAN_POINT('Ctrl Pts',(94.5884755603374,1.6450303496808,0.672218558225581));
#23407=CARTESIAN_POINT('Ctrl Pts',(94.5922687211216,1.62375216049124,0.722101444863878));
#23408=CARTESIAN_POINT('Ctrl Pts',(94.6043363441921,1.55014513178004,0.874888580446807));
#23409=CARTESIAN_POINT('Ctrl Pts',(94.6128273086695,1.49005336935094,0.973712499303621));
#23410=CARTESIAN_POINT('Ctrl Pts',(94.624698448276,1.39228204238029,1.10402667664025));
#23411=CARTESIAN_POINT('Ctrl Pts',(94.6281401868569,1.36223387969837,1.14089596374243));
#23412=CARTESIAN_POINT('Ctrl Pts',(94.6335497010757,1.31182967650287,1.19790739923428));
#23413=CARTESIAN_POINT('Ctrl Pts',(94.6355561502634,1.29240414132561,1.21884002025618));
#23414=CARTESIAN_POINT('Ctrl Pts',(94.6382151437266,1.26556468839836,1.24639815128867));
#23415=CARTESIAN_POINT('Ctrl Pts',(94.6388963698949,1.25858874815304,1.25344194380564));
#23416=CARTESIAN_POINT('Ctrl Pts',(94.640080319447,1.24628315255528,1.26566091039485));
#23417=CARTESIAN_POINT('Ctrl Pts',(94.6405849629846,1.24097936442515,1.27086169995238));
#23418=CARTESIAN_POINT('Ctrl Pts',(94.6416045169882,1.23014106483343,1.28135696762661));
#23419=CARTESIAN_POINT('Ctrl Pts',(94.6421192643879,1.22460466216027,1.28664919262809));
#23420=CARTESIAN_POINT('Ctrl Pts',(94.6434607628024,1.2100124586053,1.30041830527501));
#23421=CARTESIAN_POINT('Ctrl Pts',(94.6442832082423,1.20090160889034,1.30883660782394));
#23422=CARTESIAN_POINT('Ctrl Pts',(94.647875443551,1.16042134111926,1.34546123258851));
#23423=CARTESIAN_POINT('Ctrl Pts',(94.6505790629205,1.12813855705992,1.37264257454532));
#23424=CARTESIAN_POINT('Ctrl Pts',(94.6593501812457,1.01864791992076,1.45835591298329));
#23425=CARTESIAN_POINT('Ctrl Pts',(94.665229264986,0.937620006526667,1.51172635659943));
#23426=CARTESIAN_POINT('Ctrl Pts',(94.676708788289,0.774000347592944,1.60125681749302));
#23427=CARTESIAN_POINT('Ctrl Pts',(94.6822812130052,0.692224483696,1.63826816696401));
#23428=CARTESIAN_POINT('Ctrl Pts',(94.6897675460822,0.583128412913388,1.67801269352639));
#23429=CARTESIAN_POINT('Ctrl Pts',(94.6914913025692,0.558047931298493,1.68651941377115));
#23430=CARTESIAN_POINT('Ctrl Pts',(94.6941963081379,0.518824328153877,1.6988524452324));
#23431=CARTESIAN_POINT('Ctrl Pts',(94.6951647367994,0.504807599149018,1.7030700456644));
#23432=CARTESIAN_POINT('Ctrl Pts',(94.696976590368,0.478642792623929,1.71059159168385));
#23433=CARTESIAN_POINT('Ctrl Pts',(94.69781848405,0.466508543641666,1.71394057105261));
#23434=CARTESIAN_POINT('Ctrl Pts',(94.699706668907,0.439353296001084,1.72112552370746));
#23435=CARTESIAN_POINT('Ctrl Pts',(94.7007550619951,0.424315764836678,1.7248943423168));
#23436=CARTESIAN_POINT('Ctrl Pts',(94.7038435006594,0.380147020980542,1.73535172607837));
#23437=CARTESIAN_POINT('Ctrl Pts',(94.7059004526027,0.350895278964155,1.74150213484107));
#23438=CARTESIAN_POINT('Ctrl Pts',(94.7176422025601,0.184928678780679,1.77204683817166));
#23439=CARTESIAN_POINT('Ctrl Pts',(94.7278036701228,0.0458971188206476,
1.78107527401617));
#23440=CARTESIAN_POINT('Ctrl Pts',(94.7433518483741,-0.166687648977784,
1.76996133130152));
#23441=CARTESIAN_POINT('Ctrl Pts',(94.7487277392569,-0.240332713673877,
1.7614738598405));
#23442=CARTESIAN_POINT('Ctrl Pts',(94.7551796988284,-0.330905801390029,
1.74524713219039));
#23443=CARTESIAN_POINT('Ctrl Pts',(94.7564269756732,-0.348524627389978,
1.7418142403167));
#23444=CARTESIAN_POINT('Ctrl Pts',(94.7582661572736,-0.37471092852178,1.73629876869733));
#23445=CARTESIAN_POINT('Ctrl Pts',(94.7588683888926,-0.383319246085154,
1.73441865131664));
#23446=CARTESIAN_POINT('Ctrl Pts',(94.7599015200691,-0.398151335312461,
1.73106339548803));
#23447=CARTESIAN_POINT('Ctrl Pts',(94.7603340780327,-0.404381504539101,
1.72961861906444));
#23448=CARTESIAN_POINT('Ctrl Pts',(94.7613480160721,-0.419032773200892,
1.7261374948814));
#23449=CARTESIAN_POINT('Ctrl Pts',(94.7619277994183,-0.427446939058697,
1.72407315343835));
#23450=CARTESIAN_POINT('Ctrl Pts',(94.7636483532449,-0.452512394625666,
1.71772878054635));
#23451=CARTESIAN_POINT('Ctrl Pts',(94.7647794519678,-0.46911754416834,1.71326834279269));
#23452=CARTESIAN_POINT('Ctrl Pts',(94.7747314778119,-0.616043624103585,
1.67150496569941));
#23453=CARTESIAN_POINT('Ctrl Pts',(94.7828789277683,-0.741778709836186,
1.61963376317424));
#23454=CARTESIAN_POINT('Ctrl Pts',(94.7965158145034,-0.935389078075606,
1.51243458815743));
#23455=CARTESIAN_POINT('Ctrl Pts',(94.8018566878511,-1.00726520876277,1.46554614518653));
#23456=CARTESIAN_POINT('Ctrl Pts',(94.8090609716115,-1.09613288996187,1.39793802118573));
#23457=CARTESIAN_POINT('Ctrl Pts',(94.8107516775684,-1.11644616710133,1.38176910774818));
#23458=CARTESIAN_POINT('Ctrl Pts',(94.8134162119841,-1.14756491146864,1.35586503121801));
#23459=CARTESIAN_POINT('Ctrl Pts',(94.8143778503374,-1.15861803226294,1.34643211604601));
#23460=CARTESIAN_POINT('Ctrl Pts',(94.8161835747475,-1.17903424494436,1.32857102805436));
#23461=CARTESIAN_POINT('Ctrl Pts',(94.817026217257,-1.18842587279467,1.3201767525964));
#23462=CARTESIAN_POINT('Ctrl Pts',(94.8189247595603,-1.20927795213504,1.30113625739842));
#23463=CARTESIAN_POINT('Ctrl Pts',(94.8199828696199,-1.22068852365681,1.29043722307731));
#23464=CARTESIAN_POINT('Ctrl Pts',(94.823199919638,-1.25473719743749,1.25765602384183));
#23465=CARTESIAN_POINT('Ctrl Pts',(94.8253784186078,-1.27692724192742,1.23511971288841));
#23466=CARTESIAN_POINT('Ctrl Pts',(94.8371486320243,-1.39217754394153,1.11164421747947));
#23467=CARTESIAN_POINT('Ctrl Pts',(94.8471985692515,-1.47388785594181,1.00077644812121));
#23468=CARTESIAN_POINT('Ctrl Pts',(94.8625932444726,-1.5785141985714,0.81778177198603));
#23469=CARTESIAN_POINT('Ctrl Pts',(94.8679314715715,-1.61102415379445,0.75171626176366));
#23470=CARTESIAN_POINT('Ctrl Pts',(94.8743441197914,-1.64623516857952,0.667303579986147));
#23471=CARTESIAN_POINT('Ctrl Pts',(94.8755876235366,-1.65287477653436,0.650683742359493));
#23472=CARTESIAN_POINT('Ctrl Pts',(94.8774223810441,-1.6624034365569,0.625744618659666));
#23473=CARTESIAN_POINT('Ctrl Pts',(94.8780238922851,-1.66548343523797,0.617500161052013));
#23474=CARTESIAN_POINT('Ctrl Pts',(94.8790562658407,-1.67069552866741,0.60322583606297));
#23475=CARTESIAN_POINT('Ctrl Pts',(94.8794887784543,-1.67285647035351,0.597206992577164));
#23476=CARTESIAN_POINT('Ctrl Pts',(94.8805032981934,-1.67787150806881,0.582997842207014));
#23477=CARTESIAN_POINT('Ctrl Pts',(94.8810837006139,-1.68069818185487,0.574798148054284));
#23478=CARTESIAN_POINT('Ctrl Pts',(94.8828080409108,-1.68896401518246,0.55023799496343));
#23479=CARTESIAN_POINT('Ctrl Pts',(94.8839422436567,-1.69422534011304,0.533818177735953));
#23480=CARTESIAN_POINT('Ctrl Pts',(94.8938805171768,-1.73865437172299,0.387882644196613));
#23481=CARTESIAN_POINT('Ctrl Pts',(94.902014146064,-1.76314815696876,0.254344395044266));
#23482=CARTESIAN_POINT('Ctrl Pts',(94.9156436470429,-1.77800514207434,0.0336474295589285));
#23483=CARTESIAN_POINT('Ctrl Pts',(94.9209925513435,-1.77755341266031,-0.0523057006092893));
#23484=CARTESIAN_POINT('Ctrl Pts',(94.9282066195989,-1.76887356874582,-0.163784232731389));
#23485=CARTESIAN_POINT('Ctrl Pts',(94.9298984905342,-1.76628901444982,-0.189636446748442));
#23486=CARTESIAN_POINT('Ctrl Pts',(94.9325644519211,-1.76137581294171,-0.229849002382516));
#23487=CARTESIAN_POINT('Ctrl Pts',(94.9335263302914,-1.75943609631714,-0.244253802762519));
#23488=CARTESIAN_POINT('Ctrl Pts',(94.9353322685,-1.75548583193232,-0.271094471967802));
#23489=CARTESIAN_POINT('Ctrl Pts',(94.936174881674,-1.75351933468391,-0.283535972364107));
#23490=CARTESIAN_POINT('Ctrl Pts',(94.9380730438232,-1.74881538227752,-0.311373289543897));
#23491=CARTESIAN_POINT('Ctrl Pts',(94.9391307991114,-1.74600663579744,-0.326755821928492));
#23492=CARTESIAN_POINT('Ctrl Pts',(94.9418685414967,-1.73825985605987,-0.366225701290413));
#23493=CARTESIAN_POINT('Ctrl Pts',(94.9435578059455,-1.73302424047215,-0.390250519812725));
#23494=CARTESIAN_POINT('Ctrl Pts',(94.9527680006219,-1.7020518113678,-0.519424495736892));
#23495=CARTESIAN_POINT('Ctrl Pts',(94.9605724882779,-1.66724583457143,-0.622146704862753));
#23496=CARTESIAN_POINT('Ctrl Pts',(94.974367684127,-1.59057497328718,-0.794758207532667));
#23497=CARTESIAN_POINT('Ctrl Pts',(94.9802926039962,-1.55285040567036,-0.866155782714915));
#23498=CARTESIAN_POINT('Ctrl Pts',(94.9880073159767,-1.49628592561781,-0.957555286424896));
#23499=CARTESIAN_POINT('Ctrl Pts',(94.9899162743357,-1.48165312034302,-0.980044836723818));
#23500=CARTESIAN_POINT('Ctrl Pts',(94.9931533013092,-1.45565689703463,-1.01808519292341));
#23501=CARTESIAN_POINT('Ctrl Pts',(94.994492842988,-1.44453996153129,-1.03379825722877));
#23502=CARTESIAN_POINT('Ctrl Pts',(94.9964397486736,-1.42781948624641,-1.05663502960754));
#23503=CARTESIAN_POINT('Ctrl Pts',(94.9970591987383,-1.42241374574719,-1.06390094275559));
#23504=CARTESIAN_POINT('Ctrl Pts',(94.9981576510761,-1.41266995073597,-1.07679065208204));
#23505=CARTESIAN_POINT('Ctrl Pts',(94.998638053301,-1.40835347291731,-1.08243013565885));
#23506=CARTESIAN_POINT('Ctrl Pts',(94.9997074858732,-1.39862074363402,-1.09498917058392));
#23507=CARTESIAN_POINT('Ctrl Pts',(95.000295274383,-1.39318685066819,-1.10189458457978));
#23508=CARTESIAN_POINT('Ctrl Pts',(95.0020651534556,-1.37657646585032,-1.12268381733121));
#23509=CARTESIAN_POINT('Ctrl Pts',(95.0032367308741,-1.36524166833001,-1.13644048090984));
#23510=CARTESIAN_POINT('Ctrl Pts',(95.0108826985627,-1.2891760582864,-1.22597777126111));
#23511=CARTESIAN_POINT('Ctrl Pts',(95.0169994641277,-1.2183644697619,-1.29637551331948));
#23512=CARTESIAN_POINT('Ctrl Pts',(95.0300658645749,-1.0553379670686,-1.43322429567392));
#23513=CARTESIAN_POINT('Ctrl Pts',(95.0369961053692,-0.961918135203206,
-1.49752473354187));
#23514=CARTESIAN_POINT('Ctrl Pts',(95.0462086088977,-0.836446750404447,
-1.56727323021065));
#23515=CARTESIAN_POINT('Ctrl Pts',(95.0481806636035,-0.809497967192792,
-1.58136061964472));
#23516=CARTESIAN_POINT('Ctrl Pts',(95.0511886401256,-0.768365006204602,
-1.60153576569975));
#23517=CARTESIAN_POINT('Ctrl Pts',(95.0522065446111,-0.754440490662853,
-1.60814213072127));
#23518=CARTESIAN_POINT('Ctrl Pts',(95.0540669880168,-0.728994119532401,
-1.61981171086659));
#23519=CARTESIAN_POINT('Ctrl Pts',(95.0549073777346,-0.71750095312736,-1.6249353135456));
#23520=CARTESIAN_POINT('Ctrl Pts',(95.056739399634,-0.692455903334235,-1.63578277290479));
#23521=CARTESIAN_POINT('Ctrl Pts',(95.0577325078177,-0.678885497252915,
-1.64146121400739));
#23522=CARTESIAN_POINT('Ctrl Pts',(95.0605032897639,-0.641051475073493,
-1.65674318349393));
#23523=CARTESIAN_POINT('Ctrl Pts',(95.0622930108653,-0.616645247591543,
-1.66598123708717));
#23524=CARTESIAN_POINT('Ctrl Pts',(95.0730933858475,-0.469622138465437,
-1.71795801730542));
#23525=CARTESIAN_POINT('Ctrl Pts',(95.082527600122,-0.342842554481391,-1.74767621850269));
#23526=CARTESIAN_POINT('Ctrl Pts',(95.0968351122339,-0.148639526316249,
-1.771243377563));
#23527=CARTESIAN_POINT('Ctrl Pts',(95.1016452476878,-0.0829016188780032,
-1.77553513690401));
#23528=CARTESIAN_POINT('Ctrl Pts',(95.1088803682046,0.018248092511334,-1.77650748810208));
#23529=CARTESIAN_POINT('Ctrl Pts',(95.1113757133304,0.0535756369804111,
-1.77579331412681));
#23530=CARTESIAN_POINT('Ctrl Pts',(95.1146089270899,0.100211261944878,-1.77345733444665));
#23531=CARTESIAN_POINT('Ctrl Pts',(95.115390678858,0.111556182644242,-1.77277986487509));
#23532=CARTESIAN_POINT('Ctrl Pts',(95.1166743824403,0.1303127019245,-1.77147903212851));
#23533=CARTESIAN_POINT('Ctrl Pts',(95.1171796268895,0.137728133942607,-1.7709179341424));
#23534=CARTESIAN_POINT('Ctrl Pts',(95.1181990702182,0.152762308978348,-1.76968534737735));
#23535=CARTESIAN_POINT('Ctrl Pts',(95.1187131189579,0.160380628599035,-1.76901119592714));
#23536=CARTESIAN_POINT('Ctrl Pts',(95.1200506358053,0.180293038374202,-1.76711943600794));
#23537=CARTESIAN_POINT('Ctrl Pts',(95.120869845049,0.192579444904708,-1.76582271462945));
#23538=CARTESIAN_POINT('Ctrl Pts',(95.1244219453539,0.246192395568755,-1.75959809441629));
#23539=CARTESIAN_POINT('Ctrl Pts',(95.1270904947036,0.287355261314399,-1.75334643049213));
#23540=CARTESIAN_POINT('Ctrl Pts',(95.1358582453631,0.423887399228003,-1.72767205854021));
#23541=CARTESIAN_POINT('Ctrl Pts',(95.1417639101297,0.517877447058463,-1.70186268186232));
#23542=CARTESIAN_POINT('Ctrl Pts',(95.1532813190233,0.693661360920024,-1.63767111837042));
#23543=CARTESIAN_POINT('Ctrl Pts',(95.1588645057114,0.775569632689215,-1.60050676355487));
#23544=CARTESIAN_POINT('Ctrl Pts',(95.1663639452536,0.877549467464063,-1.54456257197392));
#23545=CARTESIAN_POINT('Ctrl Pts',(95.1680892110031,0.900498650895542,-1.5312964007958));
#23546=CARTESIAN_POINT('Ctrl Pts',(95.170796064066,0.935650901496785,-1.50991252943625));
#23547=CARTESIAN_POINT('Ctrl Pts',(95.1717648018356,0.948065412295002,-1.50214859732688));
#23548=CARTESIAN_POINT('Ctrl Pts',(95.173576938257,0.970971200338317,-1.48742644738552));
#23549=CARTESIAN_POINT('Ctrl Pts',(95.1744188017162,0.981487298961055,-1.48050841813491));
#23550=CARTESIAN_POINT('Ctrl Pts',(95.1763065340125,1.00478361710157,-1.4648256142169));
#23551=CARTESIAN_POINT('Ctrl Pts',(95.177354499995,1.01752431634909,-1.45600427070553));
#23552=CARTESIAN_POINT('Ctrl Pts',(95.1804404186302,1.05447138132665,-1.42970125183312));
#23553=CARTESIAN_POINT('Ctrl Pts',(95.1824952360227,1.07835328086762,-1.41177532823949));
#23554=CARTESIAN_POINT('Ctrl Pts',(95.1942369837869,1.21072528030964,-1.30709714128217));
#23555=CARTESIAN_POINT('Ctrl Pts',(95.2044009906684,1.30918069391501,-1.20846663201697));
#23556=CARTESIAN_POINT('Ctrl Pts',(95.2199526612276,1.44096817837964,-1.04123017214328));
#23557=CARTESIAN_POINT('Ctrl Pts',(95.2253294047492,1.4831311357932,-0.980241645017451));
#23558=CARTESIAN_POINT('Ctrl Pts',(95.2317822538845,1.53063028422761,-0.901419534870109));
#23559=CARTESIAN_POINT('Ctrl Pts',(95.2330296158846,1.53966159011307,-0.88590546597093));
#23560=CARTESIAN_POINT('Ctrl Pts',(95.2348688973155,1.55277350644968,-0.86257529287212));
#23561=CARTESIAN_POINT('Ctrl Pts',(95.2354711451779,1.55703332861872,-0.854861930429322));
#23562=CARTESIAN_POINT('Ctrl Pts',(95.2365042934527,1.56428579601105,-0.841495640838743));
#23563=CARTESIAN_POINT('Ctrl Pts',(95.2369368524538,1.56730549488526,-0.835857915242681));
#23564=CARTESIAN_POINT('Ctrl Pts',(95.2379507774485,1.57434391337453,-0.82254504737488));
#23565=CARTESIAN_POINT('Ctrl Pts',(95.2385305468916,1.57833701300949,-0.814856670691083));
#23566=CARTESIAN_POINT('Ctrl Pts',(95.2402510157348,1.5900855113624,-0.79182552374539));
#23567=CARTESIAN_POINT('Ctrl Pts',(95.2413820447975,1.59767484804097,-0.776398562132921));
#23568=CARTESIAN_POINT('Ctrl Pts',(95.2513343785186,1.66310620492509,-0.638371241198474));
#23569=CARTESIAN_POINT('Ctrl Pts',(95.2594821379166,1.70696831359905,-0.509617358587434));
#23570=CARTESIAN_POINT('Ctrl Pts',(95.2731191903442,1.7539539196056,-0.293353434769132));
#23571=CARTESIAN_POINT('Ctrl Pts',(95.278459884124,1.76606306780404,-0.20839727471165));
#23572=CARTESIAN_POINT('Ctrl Pts',(95.2856119107002,1.77373327222478,-0.0978113212449633));
#23573=CARTESIAN_POINT('Ctrl Pts',(95.2872495849426,1.77494044296943,-0.0726848531789911));
#23574=CARTESIAN_POINT('Ctrl Pts',(95.2889037169481,1.7756136383723,-0.0475422940788269));
#23575=CARTESIAN_POINT('Origin',(88.3562164250559,0.,0.));
#23576=CARTESIAN_POINT('',(96.1869838792616,1.77561363799551,-0.0475423081512957));
#23577=CARTESIAN_POINT('',(96.0403469426785,1.77561363837197,-0.0475422940912404));
#23578=CARTESIAN_POINT('',(88.3562164250559,1.77561363837197,-0.0475422940912398));
#23579=CARTESIAN_POINT('Ctrl Pts',(96.1869838792615,1.77561363799551,-0.0475423081512961));
#23580=CARTESIAN_POINT('Ctrl Pts',(96.1857088353678,1.7751328526159,-0.0654987160368496));
#23581=CARTESIAN_POINT('Ctrl Pts',(96.1844438750254,1.77438015889208,-0.0834375888448888));
#23582=CARTESIAN_POINT('Ctrl Pts',(96.1823242676866,1.77264711549215,-0.113754459212563));
#23583=CARTESIAN_POINT('Ctrl Pts',(96.1814642388469,1.7718096344516,-0.126128954223985));
#23584=CARTESIAN_POINT('Ctrl Pts',(96.1801014018478,1.77026563326307,-0.145871193086372));
#23585=CARTESIAN_POINT('Ctrl Pts',(96.179594454685,1.76964257776924,-0.153244801156153));
#23586=CARTESIAN_POINT('Ctrl Pts',(96.1786262717437,1.76835837252456,-0.167388763983415));
#23587=CARTESIAN_POINT('Ctrl Pts',(96.1781646595146,1.76770437146033,-0.174159677820498));
#23588=CARTESIAN_POINT('Ctrl Pts',(96.1771726197572,1.7662080619943,-0.18877329034128));
#23589=CARTESIAN_POINT('Ctrl Pts',(96.1766429424389,1.76535238795787,-0.196614408967168));
#23590=CARTESIAN_POINT('Ctrl Pts',(96.1752322386025,1.76292164292943,-0.217592250673031));
#23591=CARTESIAN_POINT('Ctrl Pts',(96.1743562844844,1.76125194886731,-0.230717804057732));
#23592=CARTESIAN_POINT('Ctrl Pts',(96.1700911093059,1.75233803313535,-0.295040694130992));
#23593=CARTESIAN_POINT('Ctrl Pts',(96.1668022704622,1.74300666365363,-0.345928356830504));
#23594=CARTESIAN_POINT('Ctrl Pts',(96.158256364338,1.71253779738013,-0.479035557129611));
#23595=CARTESIAN_POINT('Ctrl Pts',(96.153095153187,1.6877080152804,-0.56027103957452));
#23596=CARTESIAN_POINT('Ctrl Pts',(96.1423190744733,1.62466742839256,-0.723650590031361));
#23597=CARTESIAN_POINT('Ctrl Pts',(96.1367098101578,1.58579791136769,-0.805268139800113));
#23598=CARTESIAN_POINT('Ctrl Pts',(96.1291720542594,1.52763026622437,-0.906708946827627));
#23599=CARTESIAN_POINT('Ctrl Pts',(96.1274363557948,1.51384489714746,-0.929542280137061));
#23600=CARTESIAN_POINT('Ctrl Pts',(96.1247107667235,1.49163670038338,-0.964521673223268));
#23601=CARTESIAN_POINT('Ctrl Pts',(96.1237338599332,1.4835671888851,-0.97688816042699));
#23602=CARTESIAN_POINT('Ctrl Pts',(96.1219048125363,1.46826268301206,-0.999715202044005));
#23603=CARTESIAN_POINT('Ctrl Pts',(96.1210542185449,1.4610676585376,-1.01020150177066));
#23604=CARTESIAN_POINT('Ctrl Pts',(96.1191444932199,1.44474527060808,-1.03345118745846));
#23605=CARTESIAN_POINT('Ctrl Pts',(96.1180831935032,1.43556023075006,-1.04617257185017));
#23606=CARTESIAN_POINT('Ctrl Pts',(96.115348639551,1.41161076741906,-1.07843350737852));
#23607=CARTESIAN_POINT('Ctrl Pts',(96.1136662769424,1.39660899903011,-1.0977918693373));
#23608=CARTESIAN_POINT('Ctrl Pts',(96.1037764626145,1.30691234909745,-1.20872172087224));
#23609=CARTESIAN_POINT('Ctrl Pts',(96.0952246837161,1.22364023582482,-1.29295158645959));
#23610=CARTESIAN_POINT('Ctrl Pts',(96.0812315507888,1.07621568013534,-1.41498738769792));
#23611=CARTESIAN_POINT('Ctrl Pts',(96.0758633937944,1.01695292066245,-1.45816226063665));
#23612=CARTESIAN_POINT('Ctrl Pts',(96.0679159264959,0.923457335295051,-1.51779687471491));
#23613=CARTESIAN_POINT('Ctrl Pts',(96.0652522124573,0.891085313177671,-1.53702577551131));
#23614=CARTESIAN_POINT('Ctrl Pts',(96.0618344193847,0.847897330361275,-1.56085572996304));
#23615=CARTESIAN_POINT('Ctrl Pts',(96.0610305016613,0.837614744475606,-1.56639779458678));
#23616=CARTESIAN_POINT('Ctrl Pts',(96.0597168119931,0.820594429445155,-1.57535579695868));
#23617=CARTESIAN_POINT('Ctrl Pts',(96.0592035111115,0.813888407638603,-1.57883082408052));
#23618=CARTESIAN_POINT('Ctrl Pts',(96.0581736768961,0.800317343292535,-1.58575383432957));
#23619=CARTESIAN_POINT('Ctrl Pts',(96.0576572399717,0.793451717333784,-1.5892002551558));
#23620=CARTESIAN_POINT('Ctrl Pts',(96.0563219647286,0.775550792809677,-1.59804127003428));
#23621=CARTESIAN_POINT('Ctrl Pts',(96.0555072874269,0.764481295950203,-1.60336624077953));
#23622=CARTESIAN_POINT('Ctrl Pts',(96.0520628307256,0.717095850921767,-1.62555863764193));
#23623=CARTESIAN_POINT('Ctrl Pts',(96.0494923109065,0.680267620898655,-1.64131162497476));
#23624=CARTESIAN_POINT('Ctrl Pts',(96.040745218903,0.551248754837021,-1.69140851032364));
#23625=CARTESIAN_POINT('Ctrl Pts',(96.0347756888385,0.456757810873997,-1.71933498580347));
#23626=CARTESIAN_POINT('Ctrl Pts',(96.0231674592808,0.272039646143258,-1.75761425798143));
#23627=CARTESIAN_POINT('Ctrl Pts',(96.0175585140702,0.182385597518182,-1.76916542651245));
#23628=CARTESIAN_POINT('Ctrl Pts',(96.0100211468007,0.0656148744643614,
-1.77523801087929));
#23629=CARTESIAN_POINT('Ctrl Pts',(96.0082854929294,0.0389550962791041,
-1.77602299707647));
#23630=CARTESIAN_POINT('Ctrl Pts',(96.0055599584461,-0.00247689172977802,
-1.77630964778879));
#23631=CARTESIAN_POINT('Ctrl Pts',(96.0045830607841,-0.0172429363623765,
-1.77622767652045));
#23632=CARTESIAN_POINT('Ctrl Pts',(96.0027540216911,-0.0447210949801193,
-1.77573247293889));
#23633=CARTESIAN_POINT('Ctrl Pts',(96.0019034267566,-0.0574331912096921,
-1.77536678064391));
#23634=CARTESIAN_POINT('Ctrl Pts',(95.9999936878182,-0.0858184153194282,
-1.77424503920926));
#23635=CARTESIAN_POINT('Ctrl Pts',(95.9989323752868,-0.101487491118157,
-1.77341775143683));
#23636=CARTESIAN_POINT('Ctrl Pts',(95.9961977646379,-0.141579742644782,
-1.77076791137351));
#23637=CARTESIAN_POINT('Ctrl Pts',(95.9945153575012,-0.16597922630481,-1.76864767885796));
#23638=CARTESIAN_POINT('Ctrl Pts',(95.9846271332759,-0.307791652030535,
-1.75336441930909));
#23639=CARTESIAN_POINT('Ctrl Pts',(95.9760771432209,-0.423681990049061,
-1.72901914652318));
#23640=CARTESIAN_POINT('Ctrl Pts',(95.9620845491921,-0.606125472792167,
-1.67124021074423));
#23641=CARTESIAN_POINT('Ctrl Pts',(95.9567151438684,-0.674539649504443,
-1.64481887017444));
#23642=CARTESIAN_POINT('Ctrl Pts',(95.9487661112058,-0.775339942739593,
-1.59853968928132));
#23643=CARTESIAN_POINT('Ctrl Pts',(95.9461020474553,-0.809045954034763,
-1.58174785486638));
#23644=CARTESIAN_POINT('Ctrl Pts',(95.9426838827033,-0.852479740646801,
-1.55835772400399));
#23645=CARTESIAN_POINT('Ctrl Pts',(95.9418799300617,-0.862709571760135,
-1.55271784862184));
#23646=CARTESIAN_POINT('Ctrl Pts',(95.9405661984831,-0.879461208110358,
-1.54326572230753));
#23647=CARTESIAN_POINT('Ctrl Pts',(95.9400528901852,-0.886015501941521,
-1.53951214449439));
#23648=CARTESIAN_POINT('Ctrl Pts',(95.9390857932915,-0.89838490517734,-1.53232314997505));
#23649=CARTESIAN_POINT('Ctrl Pts',(95.9386314572816,-0.904204690934587,
-1.52889618828624));
#23650=CARTESIAN_POINT('Ctrl Pts',(95.9374154093264,-0.919800049902042,
-1.51959271514326));
#23651=CARTESIAN_POINT('Ctrl Pts',(95.9366575498323,-0.929538999700365,
-1.5136549860434));
#23652=CARTESIAN_POINT('Ctrl Pts',(95.9337711848109,-0.966671608829576,
-1.49052208848886));
#23653=CARTESIAN_POINT('Ctrl Pts',(95.9316806273558,-0.993652654860034,
-1.47267267332686));
#23654=CARTESIAN_POINT('Ctrl Pts',(95.922978621307,-1.10546082279982,-1.39423267999788));
#23655=CARTESIAN_POINT('Ctrl Pts',(95.9166532067125,-1.18536097272046,-1.3269707881487));
#23656=CARTESIAN_POINT('Ctrl Pts',(95.9045081739203,-1.3246962871328,-1.18698816532649));
#23657=CARTESIAN_POINT('Ctrl Pts',(95.8987241485187,-1.38517230602763,-1.11582079992327));
#23658=CARTESIAN_POINT('Ctrl Pts',(95.8909735744636,-1.45562086892164,-1.01831413005185));
#23659=CARTESIAN_POINT('Ctrl Pts',(95.8892137637703,-1.4709589032715,-0.99602989916447));
#23660=CARTESIAN_POINT('Ctrl Pts',(95.8864586657417,-1.49391587479961,-0.960988943519251));
#23661=CARTESIAN_POINT('Ctrl Pts',(95.8854768344005,-1.50189408401975,-0.948471680371219));
#23662=CARTESIAN_POINT('Ctrl Pts',(95.8836432665788,-1.5164120336636,-0.925051462949214));
#23663=CARTESIAN_POINT('Ctrl Pts',(95.8827931405099,-1.52299344540297,-0.914175374698735));
#23664=CARTESIAN_POINT('Ctrl Pts',(95.8808905592942,-1.53738687335471,-0.889802690713056));
#23665=CARTESIAN_POINT('Ctrl Pts',(95.8798360119085,-1.54513895298242,-0.876272112787254));
#23666=CARTESIAN_POINT('Ctrl Pts',(95.8771312793624,-1.56444365498687,-0.841524615788146));
#23667=CARTESIAN_POINT('Ctrl Pts',(95.8754723227704,-1.57574309682466,-0.820171458642281));
#23668=CARTESIAN_POINT('Ctrl Pts',(95.865071745911,-1.64322433047897,-0.686103649839787));
#23669=CARTESIAN_POINT('Ctrl Pts',(95.855932688856,-1.68771201773955,-0.567927819327141));
#23670=CARTESIAN_POINT('Ctrl Pts',(95.8417490813277,-1.73641358040554,-0.380211418463635));
#23671=CARTESIAN_POINT('Ctrl Pts',(95.8367726781835,-1.74970222175556,-0.313426044512158));
#23672=CARTESIAN_POINT('Ctrl Pts',(95.8293202086395,-1.76412474150759,-0.210308541965244));
#23673=CARTESIAN_POINT('Ctrl Pts',(95.8267698716343,-1.76803291358761,-0.174429987414859));
#23674=CARTESIAN_POINT('Ctrl Pts',(95.8234729399174,-1.77174328085655,-0.126974079396582));
#23675=CARTESIAN_POINT('Ctrl Pts',(95.8226806255155,-1.77252925621433,-0.115484733596155));
#23676=CARTESIAN_POINT('Ctrl Pts',(95.8213808444063,-1.77364361343896,-0.0964827459219574));
#23677=CARTESIAN_POINT('Ctrl Pts',(95.8208699891774,-1.77403612041142,-0.0889743681321824));
#23678=CARTESIAN_POINT('Ctrl Pts',(95.8198398880211,-1.77473515909593,-0.0737483946756312));
#23679=CARTESIAN_POINT('Ctrl Pts',(95.8193207894074,-1.77503905265561,-0.0660308862593962));
#23680=CARTESIAN_POINT('Ctrl Pts',(95.8179703128861,-1.77570210583479,-0.0458442284910022));
#23681=CARTESIAN_POINT('Ctrl Pts',(95.8171432743464,-1.77598027968316,-0.0333725939401568));
#23682=CARTESIAN_POINT('Ctrl Pts',(95.813549365582,-1.77662292201165,0.021244119641939));
#23683=CARTESIAN_POINT('Ctrl Pts',(95.8108484098556,-1.77561877165931,0.0633949461116137));
#23684=CARTESIAN_POINT('Ctrl Pts',(95.8020813766487,-1.76736554275527,0.202139892270353));
#23685=CARTESIAN_POINT('Ctrl Pts',(95.7962035681913,-1.75371967524114,0.298179634677757));
#23686=CARTESIAN_POINT('Ctrl Pts',(95.785292447043,-1.71453330414794,0.471071410675169));
#23687=CARTESIAN_POINT('Ctrl Pts',(95.7802986229555,-1.69144982642376,0.548204695159838));
#23688=CARTESIAN_POINT('Ctrl Pts',(95.7730926859472,-1.65195983692871,0.653545779987085));
#23689=CARTESIAN_POINT('Ctrl Pts',(95.7710148279853,-1.63988668098069,0.683275096808986));
#23690=CARTESIAN_POINT('Ctrl Pts',(95.767872295538,-1.62066802240979,0.72715165616608));
#23691=CARTESIAN_POINT('Ctrl Pts',(95.7668280295796,-1.61412718479698,0.741557667491839));
#23692=CARTESIAN_POINT('Ctrl Pts',(95.764931849606,-1.60197973373417,0.767389686379089));
#23693=CARTESIAN_POINT('Ctrl Pts',(95.7640823291062,-1.59644104046476,0.778846575315385));
#23694=CARTESIAN_POINT('Ctrl Pts',(95.7622443094546,-1.58425437049338,0.803378669922324));
#23695=CARTESIAN_POINT('Ctrl Pts',(95.7612544636352,-1.57756661614441,0.816432940798284));
#23696=CARTESIAN_POINT('Ctrl Pts',(95.7585291912953,-1.55881944883748,0.851936226078057));
#23697=CARTESIAN_POINT('Ctrl Pts',(95.7567825024734,-1.54643780892014,0.87421015381732));
#23698=CARTESIAN_POINT('Ctrl Pts',(95.7450241734097,-1.46071040510407,1.02090582666248));
#23699=CARTESIAN_POINT('Ctrl Pts',(95.7344729536275,-1.37291393775626,1.13622862133275));
#23700=CARTESIAN_POINT('Ctrl Pts',(95.7183986448979,-1.219367518874,1.29380380818812));
#23701=CARTESIAN_POINT('Ctrl Pts',(95.7129027913528,-1.16316742806164,1.34455536621618));
#23702=CARTESIAN_POINT('Ctrl Pts',(95.7063203577418,-1.08964929001053,1.40287535192581));
#23703=CARTESIAN_POINT('Ctrl Pts',(95.705056114969,-1.07522756662815,1.41395918343043));
#23704=CARTESIAN_POINT('Ctrl Pts',(95.7031934580536,-1.0534910329906,1.43013988049136));
#23705=CARTESIAN_POINT('Ctrl Pts',(95.7025844425084,-1.04630448431426,1.43540599450567));
#23706=CARTESIAN_POINT('Ctrl Pts',(95.7015400961272,-1.03383781301543,1.44439786437568));
#23707=CARTESIAN_POINT('Ctrl Pts',(95.7011030674611,-1.02857666156881,1.44814911844296));
#23708=CARTESIAN_POINT('Ctrl Pts',(95.7000784966573,-1.01613804981689,1.45691598604226));
#23709=CARTESIAN_POINT('Ctrl Pts',(95.699492586269,-1.00894383613061,1.46190733985422));
#23710=CARTESIAN_POINT('Ctrl Pts',(95.697788036691,-0.987787033792288,1.47635537900139));
#23711=CARTESIAN_POINT('Ctrl Pts',(95.6966784986424,-0.973725903815361,
1.48566696951904));
#23712=CARTESIAN_POINT('Ctrl Pts',(95.6882267718352,-0.86458844862292,1.55572493940772));
#23713=CARTESIAN_POINT('Ctrl Pts',(95.6813523267443,-0.764038928621692,
1.60749640850409));
#23714=CARTESIAN_POINT('Ctrl Pts',(95.667498007156,-0.554481991437766,1.69125469372554));
#23715=CARTESIAN_POINT('Ctrl Pts',(95.6605430926195,-0.445981092520281,
1.72304653740317));
#23716=CARTESIAN_POINT('Ctrl Pts',(95.6517109121644,-0.311962272368679,
1.74880067202562));
#23717=CARTESIAN_POINT('Ctrl Pts',(95.6501658080794,-0.288633266760026,
1.75280204270756));
#23718=CARTESIAN_POINT('Ctrl Pts',(95.6476738186553,-0.251245585136907,
1.75844812363736));
#23719=CARTESIAN_POINT('Ctrl Pts',(95.6467364491784,-0.237234649738997,
1.76039309501794));
#23720=CARTESIAN_POINT('Ctrl Pts',(95.6449400323858,-0.210493808185803,
1.76378017804981));
#23721=CARTESIAN_POINT('Ctrl Pts',(95.6440819941082,-0.197768557752873,
1.76525231693797));
#23722=CARTESIAN_POINT('Ctrl Pts',(95.6421155307026,-0.168719434020354,
1.76829486450532));
#23723=CARTESIAN_POINT('Ctrl Pts',(95.6410044038167,-0.152387711550758,
1.76977708457753));
#23724=CARTESIAN_POINT('Ctrl Pts',(95.6374089023799,-0.09981889961668,1.77381505042585));
#23725=CARTESIAN_POINT('Ctrl Pts',(95.6348973814402,-0.063525191819601,
1.77548524671327));
#23726=CARTESIAN_POINT('Ctrl Pts',(95.6231038350541,0.104856772634574,1.77806476654996));
#23727=CARTESIAN_POINT('Ctrl Pts',(95.6134218673755,0.236718578700988,1.7653507731331));
#23728=CARTESIAN_POINT('Ctrl Pts',(95.5985429796091,0.436147228549847,1.72336559272204));
#23729=CARTESIAN_POINT('Ctrl Pts',(95.5933395357185,0.505413324934643,1.70433937581619));
#23730=CARTESIAN_POINT('Ctrl Pts',(95.5870624641416,0.590165793088469,1.67543555114067));
#23731=CARTESIAN_POINT('Ctrl Pts',(95.5858276220592,0.606901412779942,1.66944622096831));
#23732=CARTESIAN_POINT('Ctrl Pts',(95.5839994542171,0.631812225563644,1.66010702244092));
#23733=CARTESIAN_POINT('Ctrl Pts',(95.5833960685007,0.640056364220105,1.65694594761901));
#23734=CARTESIAN_POINT('Ctrl Pts',(95.5823087803806,0.654958849483811,1.65110401824517));
#23735=CARTESIAN_POINT('Ctrl Pts',(95.5818237222529,0.661624816911754,1.64844416927022));
#23736=CARTESIAN_POINT('Ctrl Pts',(95.5807213507672,0.676813498223356,1.64227661520591));
#23737=CARTESIAN_POINT('Ctrl Pts',(95.5801055890829,0.685325247178726,1.63874290453633));
#23738=CARTESIAN_POINT('Ctrl Pts',(95.5781767647745,0.712059049960596,1.62739945507824));
#23739=CARTESIAN_POINT('Ctrl Pts',(95.5768770499164,0.730178778358473,1.61935052067257));
#23740=CARTESIAN_POINT('Ctrl Pts',(95.5670202812097,0.868016880735461,1.55533742030664));
#23741=CARTESIAN_POINT('Ctrl Pts',(95.5590722976478,0.981302431900621,1.48646647756767));
#23742=CARTESIAN_POINT('Ctrl Pts',(95.5471334822186,1.1346001753285,1.36803957326225));
#23743=CARTESIAN_POINT('Ctrl Pts',(95.5433111014641,1.18130134629904,1.32792173966354));
#23744=CARTESIAN_POINT('Ctrl Pts',(95.5367914287634,1.25563475894926,1.25703705903914));
#23745=CARTESIAN_POINT('Ctrl Pts',(95.5341422734579,1.28444510922151,1.22758346575362));
#23746=CARTESIAN_POINT('Ctrl Pts',(95.5303137582553,1.32390746776737,1.18432875825583));
#23747=CARTESIAN_POINT('Ctrl Pts',(95.5291708018469,1.33542174283353,1.17133015169096));
#23748=CARTESIAN_POINT('Ctrl Pts',(95.5271644550749,1.3551583480396,1.14837993674027));
#23749=CARTESIAN_POINT('Ctrl Pts',(95.5263046860705,1.3634663318484,1.13850348011373));
#23750=CARTESIAN_POINT('Ctrl Pts',(95.5245137057603,1.38045893542429,1.11785004956742));
#23751=CARTESIAN_POINT('Ctrl Pts',(95.5235818915888,1.38912666775141,1.10706038126636));
#23752=CARTESIAN_POINT('Ctrl Pts',(95.5211412928642,1.41137427847528,1.07869367359434));
#23753=CARTESIAN_POINT('Ctrl Pts',(95.5196246701492,1.42475174350624,1.06096172722781));
#23754=CARTESIAN_POINT('Ctrl Pts',(95.5121583516474,1.488414479755,0.973200273630984));
#23755=CARTESIAN_POINT('Ctrl Pts',(95.5060301775853,1.53388114915522,0.899833935221259));
#23756=CARTESIAN_POINT('Ctrl Pts',(95.4921639787674,1.62261690690744,0.730239192960171));
#23757=CARTESIAN_POINT('Ctrl Pts',(95.4843916851545,1.66301443226564,0.632864401789094));
#23758=CARTESIAN_POINT('Ctrl Pts',(95.4746051898091,1.70372718705269,0.503302718569362));
#23759=CARTESIAN_POINT('Ctrl Pts',(95.472419549125,1.71214324211356,0.47388361867349));
#23760=CARTESIAN_POINT('Ctrl Pts',(95.4687681982979,1.72510549850677,0.423704850839405));
#23761=CARTESIAN_POINT('Ctrl Pts',(95.4672872024097,1.73004674409583,0.403054765023951));
#23762=CARTESIAN_POINT('Ctrl Pts',(95.465172997492,1.73665430994928,0.373075699939175));
#23763=CARTESIAN_POINT('Ctrl Pts',(95.4645248216293,1.73861792765303,0.36381503815655));
#23764=CARTESIAN_POINT('Ctrl Pts',(95.4633914734083,1.74194294042276,0.347491835791105));
#23765=CARTESIAN_POINT('Ctrl Pts',(95.4629046089788,1.74333560496434,0.340436129825559));
#23766=CARTESIAN_POINT('Ctrl Pts',(95.4618390161632,1.74630494913922,0.324896206123856));
#23767=CARTESIAN_POINT('Ctrl Pts',(95.4612613393909,1.74786270369423,0.316408749828724));
#23768=CARTESIAN_POINT('Ctrl Pts',(95.4596042938894,1.75217779793138,0.291892996066376));
#23769=CARTESIAN_POINT('Ctrl Pts',(95.4585332800772,1.75477702331477,0.275837272882306));
#23770=CARTESIAN_POINT('Ctrl Pts',(95.4507634051892,1.77219199933964,0.158027365034681));
#23771=CARTESIAN_POINT('Ctrl Pts',(95.4444585957157,1.77836486843091,0.0552108353318123));
#23772=CARTESIAN_POINT('Ctrl Pts',(95.4381488398588,1.77561363782069,-0.0475423146804777));
#23773=CARTESIAN_POINT('Ctrl Pts',(95.2889037169481,1.7756136383723,-0.0475422940788269));
#23774=CARTESIAN_POINT('Ctrl Pts',(95.2889567569751,1.77563522449855,-0.0467360936017572));
#23775=CARTESIAN_POINT('Ctrl Pts',(95.2890098138606,1.77565626160278,-0.0459298765760937));
#23776=CARTESIAN_POINT('Ctrl Pts',(95.2900191314892,1.77604588821666,-0.030597539362922));
#23777=CARTESIAN_POINT('Ctrl Pts',(95.2909807644722,1.77623675511927,-0.0160678287640855));
#23778=CARTESIAN_POINT('Ctrl Pts',(95.292786484101,1.77626023938196,0.0110584591401438));
#23779=CARTESIAN_POINT('Ctrl Pts',(95.2936291272694,1.77613715526875,0.0236541558387008));
#23780=CARTESIAN_POINT('Ctrl Pts',(95.2955276780908,1.77556092417017,0.0518857780285321));
#23781=CARTESIAN_POINT('Ctrl Pts',(95.2965857960983,1.77503517899466,0.0675190001902518));
#23782=CARTESIAN_POINT('Ctrl Pts',(95.2993251477812,1.77315133809973,0.107720967200315));
#23783=CARTESIAN_POINT('Ctrl Pts',(95.3010156772862,1.77148910383564,0.132271403366321));
#23784=CARTESIAN_POINT('Ctrl Pts',(95.3100389491564,1.76000280663643,0.26189966955908));
#23785=CARTESIAN_POINT('Ctrl Pts',(95.317639745967,1.74133979125052,0.365965209429774));
#23786=CARTESIAN_POINT('Ctrl Pts',(95.3313800827805,1.69178020528202,0.54752442454029));
#23787=CARTESIAN_POINT('Ctrl Pts',(95.3374587743909,1.66445716285109,0.625688772466514));
#23788=CARTESIAN_POINT('Ctrl Pts',(95.3453486436257,1.62105031371086,0.726635141924815));
#23789=CARTESIAN_POINT('Ctrl Pts',(95.3472834545113,1.60974170785838,0.751355136635535));
#23790=CARTESIAN_POINT('Ctrl Pts',(95.3505592873381,1.58938214784155,0.793288141020426));
#23791=CARTESIAN_POINT('Ctrl Pts',(95.3519121247525,1.58060791319242,0.810629624762761));
#23792=CARTESIAN_POINT('Ctrl Pts',(95.353874481689,1.56731387071871,0.835867170273672));
#23793=CARTESIAN_POINT('Ctrl Pts',(95.3544963506445,1.56301553476532,0.84387744540039));
#23794=CARTESIAN_POINT('Ctrl Pts',(95.3555973085542,1.55524937915512,0.85808733931189));
#23795=CARTESIAN_POINT('Ctrl Pts',(95.3560778260503,1.55180565123194,0.864299565729837));
#23796=CARTESIAN_POINT('Ctrl Pts',(95.3571453502307,1.54403351899381,0.878123693241679));
#23797=CARTESIAN_POINT('Ctrl Pts',(95.3577311410998,1.53968599991507,0.885724425640546));
#23798=CARTESIAN_POINT('Ctrl Pts',(95.3594886364846,1.52639876248971,0.908560900650809));
#23799=CARTESIAN_POINT('Ctrl Pts',(95.3606500423319,1.51728751014733,0.923696249839533));
#23800=CARTESIAN_POINT('Ctrl Pts',(95.3704647085506,1.43761189875432,1.05169001771807));
#23801=CARTESIAN_POINT('Ctrl Pts',(95.3784742427342,1.35478459329991,1.1564378834565));
#23802=CARTESIAN_POINT('Ctrl Pts',(95.3920387478449,1.19968572964695,1.31278430215599));
#23803=CARTESIAN_POINT('Ctrl Pts',(95.397460708626,1.13389482277488,1.37001041091376));
#23804=CARTESIAN_POINT('Ctrl Pts',(95.4047637773581,1.04324417362927,1.43784186419669));
#23805=CARTESIAN_POINT('Ctrl Pts',(95.4064661838775,1.02196834910212,1.45304102179414));
#23806=CARTESIAN_POINT('Ctrl Pts',(95.4091450488351,0.988327214095373,1.47596938510215));
#23807=CARTESIAN_POINT('Ctrl Pts',(95.41010909565,0.976188565537531,1.48402566390425));
#23808=CARTESIAN_POINT('Ctrl Pts',(95.4119169751055,0.953375225851697,1.4987656002174));
#23809=CARTESIAN_POINT('Ctrl Pts',(95.4127593329812,0.942725826917928,1.50548684711106));
#23810=CARTESIAN_POINT('Ctrl Pts',(95.4146541083425,0.918733523813713,1.5202749294355));
#23811=CARTESIAN_POINT('Ctrl Pts',(95.4157086968476,0.905354201517406,1.52828037073147));
#23812=CARTESIAN_POINT('Ctrl Pts',(95.4188338191507,0.865643058637727,1.5513368422232));
#23813=CARTESIAN_POINT('Ctrl Pts',(95.4209218709622,0.839030299551189,1.56589011837562));
#23814=CARTESIAN_POINT('Ctrl Pts',(95.4326637930602,0.689018250436116,1.64300255133708));
#23815=CARTESIAN_POINT('Ctrl Pts',(95.4427884366524,0.559026885822932,1.69165001133641));
#23816=CARTESIAN_POINT('Ctrl Pts',(95.4582859577275,0.352994575201968,1.74238870317995));
#23817=CARTESIAN_POINT('Ctrl Pts',(95.4636494593696,0.280209969315898,1.755564870218));
#23818=CARTESIAN_POINT('Ctrl Pts',(95.4700884913032,0.189001250514819,1.7662570887508));
#23819=CARTESIAN_POINT('Ctrl Pts',(95.4713345295017,0.171160936196939,1.76807510357048));
#23820=CARTESIAN_POINT('Ctrl Pts',(95.4731722589091,0.144520660305005,1.77038284380619));
#23821=CARTESIAN_POINT('Ctrl Pts',(95.4737742541813,0.135740233241383,1.77107770362842));
#23822=CARTESIAN_POINT('Ctrl Pts',(95.4748071366485,0.120575778910655,1.7721643390175));
#23823=CARTESIAN_POINT('Ctrl Pts',(95.47523967959,0.114194424307764,1.77258697953274));
#23824=CARTESIAN_POINT('Ctrl Pts',(95.476253807791,0.0991600884922154,1.7735011833066));
#23825=CARTESIAN_POINT('Ctrl Pts',(95.4768337937103,0.0905056281993163,
1.77396389745605));
#23826=CARTESIAN_POINT('Ctrl Pts',(95.478555586038,0.0646582664232599,1.7751561856315));
#23827=CARTESIAN_POINT('Ctrl Pts',(95.4796876999827,0.0474572288909502,
1.77569931019369));
#23828=CARTESIAN_POINT('Ctrl Pts',(95.4896352351377,-0.10520247665701,1.77829954263295));
#23829=CARTESIAN_POINT('Ctrl Pts',(95.4977781717089,-0.240493755347008,
1.76510343682338));
#23830=CARTESIAN_POINT('Ctrl Pts',(95.5114126433726,-0.456831123819215,
1.71864017195717));
#23831=CARTESIAN_POINT('Ctrl Pts',(95.5167561370058,-0.539255165748686,
1.69458554633152));
#23832=CARTESIAN_POINT('Ctrl Pts',(95.5239636132052,-0.643949959118246,
1.65561673851572));
#23833=CARTESIAN_POINT('Ctrl Pts',(95.5256546994125,-0.668082972303091,
1.64602653817489));
#23834=CARTESIAN_POINT('Ctrl Pts',(95.5283196995966,-0.705380083268758,
1.63024973017905));
#23835=CARTESIAN_POINT('Ctrl Pts',(95.529281416297,-0.718693702021668,1.62442438610772));
#23836=CARTESIAN_POINT('Ctrl Pts',(95.5310872104721,-0.74341101328943,1.61324604133307));
#23837=CARTESIAN_POINT('Ctrl Pts',(95.5319298433819,-0.754832206891317,
1.60793378280441));
#23838=CARTESIAN_POINT('Ctrl Pts',(95.533828261477,-0.780305862201823,1.59575419011407));
#23839=CARTESIAN_POINT('Ctrl Pts',(95.5348862556368,-0.794325908626361,
1.58882188976646));
#23840=CARTESIAN_POINT('Ctrl Pts',(95.5376250578013,-0.830156982302269,
1.5705121959691));
#23841=CARTESIAN_POINT('Ctrl Pts',(95.539315155324,-0.851825866566442,1.55886553642567));
#23842=CARTESIAN_POINT('Ctrl Pts',(95.5484254009532,-0.966242777113065,
1.49427041779988));
#23843=CARTESIAN_POINT('Ctrl Pts',(95.5561207371852,-1.05430147796885,1.43349602441605));
#23844=CARTESIAN_POINT('Ctrl Pts',(95.5698862838805,-1.19918587652719,1.31289740833896));
#23845=CARTESIAN_POINT('Ctrl Pts',(95.5758932017624,-1.25833059591255,1.25632453254595));
#23846=CARTESIAN_POINT('Ctrl Pts',(95.5837013943358,-1.33155823116844,1.17590244557733));
#23847=CARTESIAN_POINT('Ctrl Pts',(95.5856242166804,-1.34928941567765,1.15551378754126));
#23848=CARTESIAN_POINT('Ctrl Pts',(95.5888820635261,-1.37890838680442,1.11984373617836));
#23849=CARTESIAN_POINT('Ctrl Pts',(95.5902287441765,-1.39102395060464,1.10475824404048));
#23850=CARTESIAN_POINT('Ctrl Pts',(95.5921839484508,-1.40845705758532,1.08231008662252));
#23851=CARTESIAN_POINT('Ctrl Pts',(95.5928046992405,-1.41396804478474,1.0751003599824));
#23852=CARTESIAN_POINT('Ctrl Pts',(95.5939044971344,-1.42369348697048,1.0621729430886));
#23853=CARTESIAN_POINT('Ctrl Pts',(95.5943849595714,-1.42792918040901,1.05647184856721));
#23854=CARTESIAN_POINT('Ctrl Pts',(95.5954533580801,-1.43731874894874,1.04367417808829));
#23855=CARTESIAN_POINT('Ctrl Pts',(95.596040066375,-1.44245438550155,1.03656467717824));
#23856=CARTESIAN_POINT('Ctrl Pts',(95.5978032427166,-1.45781674004315,1.014962570548));
#23857=CARTESIAN_POINT('Ctrl Pts',(95.5989693139755,-1.46787958669407,1.00035405976913));
#23858=CARTESIAN_POINT('Ctrl Pts',(95.6087621676403,-1.55136118722488,0.875188621493969));
#23859=CARTESIAN_POINT('Ctrl Pts',(95.616749833043,-1.61240478340171,0.756860218467986));
#23860=CARTESIAN_POINT('Ctrl Pts',(95.6303031327307,-1.69080498883349,0.551240022642908));
#23861=CARTESIAN_POINT('Ctrl Pts',(95.635738147226,-1.71585017495635,0.467485571504157));
#23862=CARTESIAN_POINT('Ctrl Pts',(95.6430571171658,-1.74026808789838,0.356673740675966));
#23863=CARTESIAN_POINT('Ctrl Pts',(95.644761394455,-1.74533472498702,0.330992081121534));
#23864=CARTESIAN_POINT('Ctrl Pts',(95.6474425503943,-1.75233620935234,0.290850980786398));
#23865=CARTESIAN_POINT('Ctrl Pts',(95.6484069818381,-1.75466366536883,0.276463168926865));
#23866=CARTESIAN_POINT('Ctrl Pts',(95.6502152074162,-1.75867150712158,0.249593997069679));
#23867=CARTESIAN_POINT('Ctrl Pts',(95.6510575218129,-1.76039672802214,0.237120178823154));
#23868=CARTESIAN_POINT('Ctrl Pts',(95.6529517052858,-1.76395984030129,0.209171180553178));
#23869=CARTESIAN_POINT('Ctrl Pts',(95.6540057391991,-1.76572697637211,0.193688200059735));
#23870=CARTESIAN_POINT('Ctrl Pts',(95.6567269893385,-1.7697381345931,0.153904242847135));
#23871=CARTESIAN_POINT('Ctrl Pts',(95.6584032945087,-1.77168541033969,0.129577331701055));
#23872=CARTESIAN_POINT('Ctrl Pts',(95.6682799282808,-1.78012561000926,-0.0126552740673993));
#23873=CARTESIAN_POINT('Ctrl Pts',(95.6768242920583,-1.77534785518076,-0.13091404682957));
#23874=CARTESIAN_POINT('Ctrl Pts',(95.6908325577483,-1.7486190217658,-0.320631832753723));
#23875=CARTESIAN_POINT('Ctrl Pts',(95.6962229262214,-1.7338447082113,-0.392755283832904));
#23876=CARTESIAN_POINT('Ctrl Pts',(95.7041929795941,-1.70480804625936,-0.500111891028008));
#23877=CARTESIAN_POINT('Ctrl Pts',(95.7068580308758,-1.69382078244656,-0.536147370772488));
#23878=CARTESIAN_POINT('Ctrl Pts',(95.7102722677517,-1.6779569328271,-0.582803086805409));
#23879=CARTESIAN_POINT('Ctrl Pts',(95.7110714577312,-1.67411088460751,-0.593760617247399));
#23880=CARTESIAN_POINT('Ctrl Pts',(95.7123760738497,-1.66760841364111,-0.611720779228909));
#23881=CARTESIAN_POINT('Ctrl Pts',(95.7128850017494,-1.66501473709595,-0.618745557040854));
#23882=CARTESIAN_POINT('Ctrl Pts',(95.7139040863731,-1.65970411830595,-0.632853736697608));
#23883=CARTESIAN_POINT('Ctrl Pts',(95.7144141683819,-1.65698607423378,-0.639936534062021));
#23884=CARTESIAN_POINT('Ctrl Pts',(95.7157290334178,-1.6498264013224,-0.658242034933834));
#23885=CARTESIAN_POINT('Ctrl Pts',(95.7165298199042,-1.6453155323066,-0.669437487859746));
#23886=CARTESIAN_POINT('Ctrl Pts',(95.7198650187112,-1.62591156038618,-0.716214669699074));
#23887=CARTESIAN_POINT('Ctrl Pts',(95.7223444979818,-1.60997452978397,-0.7513550160481));
#23888=CARTESIAN_POINT('Ctrl Pts',(95.7336227994741,-1.53112981094059,-0.911151326632204));
#23889=CARTESIAN_POINT('Ctrl Pts',(95.7419603957487,-1.45480748555993,-1.02863789231543));
#23890=CARTESIAN_POINT('Ctrl Pts',(95.7546477826124,-1.32482782509322,-1.18488034935258));
#23891=CARTESIAN_POINT('Ctrl Pts',(95.7586811772971,-1.28155381786269,-1.23155540312163));
#23892=CARTESIAN_POINT('Ctrl Pts',(95.7641204709636,-1.22151773540648,-1.28971235158172));
#23893=CARTESIAN_POINT('Ctrl Pts',(95.7654308678538,-1.20692898869114,-1.30337480831913));
#23894=CARTESIAN_POINT('Ctrl Pts',(95.7676300889238,-1.18226136993859,-1.32570687810135));
#23895=CARTESIAN_POINT('Ctrl Pts',(95.7685129864217,-1.17230990650838,-1.33451494568973));
#23896=CARTESIAN_POINT('Ctrl Pts',(95.7702590175617,-1.15254162724532,-1.35162015635374));
#23897=CARTESIAN_POINT('Ctrl Pts',(95.7711217948082,-1.14273172177401,-1.35992405912022));
#23898=CARTESIAN_POINT('Ctrl Pts',(95.7730348533302,-1.12089395174406,-1.37800619462187));
#23899=CARTESIAN_POINT('Ctrl Pts',(95.7740870541833,-1.10882657378586,-1.38773481836656));
#23900=CARTESIAN_POINT('Ctrl Pts',(95.7777356205297,-1.06680023153331,-1.42071798097195));
#23901=CARTESIAN_POINT('Ctrl Pts',(95.7803628946681,-1.03622664760975,-1.44316882991483));
#23902=CARTESIAN_POINT('Ctrl Pts',(95.7921189217657,-0.898136643439155,
-1.53792014364113));
#23903=CARTESIAN_POINT('Ctrl Pts',(95.8016211782258,-0.783627371509781,
-1.59930192188895));
#23904=CARTESIAN_POINT('Ctrl Pts',(95.8162594180626,-0.597602680518702,
-1.6742101222443));
#23905=CARTESIAN_POINT('Ctrl Pts',(95.8214073029766,-0.530180878403013,
-1.69676712207639));
#23906=CARTESIAN_POINT('Ctrl Pts',(95.8276207821158,-0.444567243197875,
-1.71980654548467));
#23907=CARTESIAN_POINT('Ctrl Pts',(95.8288448671336,-0.427482890095324,
-1.72413254277283));
#23908=CARTESIAN_POINT('Ctrl Pts',(95.8306568320006,-0.40182520859577,-1.73022457642646));
#23909=CARTESIAN_POINT('Ctrl Pts',(95.8312546154195,-0.393299177310323,
-1.73218253899933));
#23910=CARTESIAN_POINT('Ctrl Pts',(95.832283089745,-0.378517749760222,-1.73546225656846));
#23911=CARTESIAN_POINT('Ctrl Pts',(95.8327153889454,-0.372269336219983,
-1.73681331051157));
#23912=CARTESIAN_POINT('Ctrl Pts',(95.8337330207187,-0.357477166869674,
-1.73992822746252));
#23913=CARTESIAN_POINT('Ctrl Pts',(95.8343167064039,-0.348927549244659,
-1.74166292231038));
#23914=CARTESIAN_POINT('Ctrl Pts',(95.8360612059315,-0.323191439976269,
-1.74668759047755));
#23915=CARTESIAN_POINT('Ctrl Pts',(95.8372119438464,-0.305968200185593,
-1.74978677634062));
#23916=CARTESIAN_POINT('Ctrl Pts',(95.8470757825022,-0.156505527743785,
-1.77440693285009));
#23917=CARTESIAN_POINT('Ctrl Pts',(95.8551346510661,-0.0222519488528085,
-1.78115945505472));
#23918=CARTESIAN_POINT('Ctrl Pts',(95.86872470928,0.197921036881598,-1.76731141462302));
#23919=CARTESIAN_POINT('Ctrl Pts',(95.8741174196764,0.28382058694742,-1.75556423829484));
#23920=CARTESIAN_POINT('Ctrl Pts',(95.8813848559755,0.394026871901089,-1.7321913853027));
#23921=CARTESIAN_POINT('Ctrl Pts',(95.8830830576458,0.419414942951327,-1.72621990571574));
#23922=CARTESIAN_POINT('Ctrl Pts',(95.8857567729684,0.458752965389729,-1.71604825970502));
#23923=CARTESIAN_POINT('Ctrl Pts',(95.8867199548095,0.472798910454391,-1.71223160873554));
#23924=CARTESIAN_POINT('Ctrl Pts',(95.8885270578465,0.498907941972941,-1.70479134780101));
#23925=CARTESIAN_POINT('Ctrl Pts',(95.8893695154734,0.510982533524763,-1.70121118924979));
#23926=CARTESIAN_POINT('Ctrl Pts',(95.8912656315735,0.53793498192917,-1.6929068685143));
#23927=CARTESIAN_POINT('Ctrl Pts',(95.8923214750549,0.552790529390272,-1.68811442553147));
#23928=CARTESIAN_POINT('Ctrl Pts',(95.8950507405519,0.590789138473322,-1.67530061332203));
#23929=CARTESIAN_POINT('Ctrl Pts',(95.8967333428618,0.61383227082159,-1.66699543803297));
#23930=CARTESIAN_POINT('Ctrl Pts',(95.9063472607885,0.743293026964865,-1.61728718471595));
#23931=CARTESIAN_POINT('Ctrl Pts',(95.9145978230967,0.845678409672861,-1.56618080532499));
#23932=CARTESIAN_POINT('Ctrl Pts',(95.9285195167745,1.00712684056962,-1.46512257049888));
#23933=CARTESIAN_POINT('Ctrl Pts',(95.9341182687157,1.0691429145886,-1.42050095619035));
#23934=CARTESIAN_POINT('Ctrl Pts',(95.9414592995003,1.14821880294892,-1.35548373379674));
#23935=CARTESIAN_POINT('Ctrl Pts',(95.9433112967371,1.16797394824887,-1.33849899911817));
#23936=CARTESIAN_POINT('Ctrl Pts',(95.9464625537674,1.20135449122553,-1.30849762554876));
#23937=CARTESIAN_POINT('Ctrl Pts',(95.9477725475971,1.21515931674008,-1.29568767661392));
#23938=CARTESIAN_POINT('Ctrl Pts',(95.9496850503181,1.23524206220112,-1.27644887287705));
#23939=CARTESIAN_POINT('Ctrl Pts',(95.9502990688375,1.24167863245428,-1.27018851348149));
#23940=CARTESIAN_POINT('Ctrl Pts',(95.9513919490235,1.25311975636645,-1.25889052425667));
#23941=CARTESIAN_POINT('Ctrl Pts',(95.9518721462221,1.25814187298278,-1.25387140813795));
#23942=CARTESIAN_POINT('Ctrl Pts',(95.9529461021718,1.26936222072975,-1.24252247040516));
#23943=CARTESIAN_POINT('Ctrl Pts',(95.9535385585971,1.27554334277323,-1.23617625197792));
#23944=CARTESIAN_POINT('Ctrl Pts',(95.9553375761283,1.29427529917168,-1.21665386605456));
#23945=CARTESIAN_POINT('Ctrl Pts',(95.9565331108233,1.3066718025701,-1.20333039657947));
#23946=CARTESIAN_POINT('Ctrl Pts',(95.9633972034397,1.37736840248741,-1.12496627388031));
#23947=CARTESIAN_POINT('Ctrl Pts',(95.9687956673541,1.43101906050624,-1.05587921425144));
#23948=CARTESIAN_POINT('Ctrl Pts',(95.9793254826991,1.52583142595219,-0.913207675557202));
#23949=CARTESIAN_POINT('Ctrl Pts',(95.9844471332954,1.56727508045992,-0.840094022792539));
#23950=CARTESIAN_POINT('Ctrl Pts',(95.9934777140294,1.62940089865141,-0.709767542782186));
#23951=CARTESIAN_POINT('Ctrl Pts',(95.9973173968418,1.65260504635709,-0.653920992698155));
#23952=CARTESIAN_POINT('Ctrl Pts',(96.0025331444676,1.67953018389623,-0.578471802134207));
#23953=CARTESIAN_POINT('Ctrl Pts',(96.0038237967921,1.6858352068965,-0.559831107542047));
#23954=CARTESIAN_POINT('Ctrl Pts',(96.0059991081082,1.69585849454098,-0.52849124562871));
#23955=CARTESIAN_POINT('Ctrl Pts',(96.0068781186967,1.69974697748888,-0.515848065441243));
#23956=CARTESIAN_POINT('Ctrl Pts',(96.008623586272,1.70714797954547,-0.490791447347547));
#23957=CARTESIAN_POINT('Ctrl Pts',(96.0094897625665,1.71066719104934,-0.478380826411765));
#23958=CARTESIAN_POINT('Ctrl Pts',(96.0114193483744,1.71816656864189,-0.450792509157177));
#23959=CARTESIAN_POINT('Ctrl Pts',(96.0124848000822,1.72208138749042,-0.435598336943335));
#23960=CARTESIAN_POINT('Ctrl Pts',(96.0162287471553,1.73504945879935,-0.382357055584056));
#23961=CARTESIAN_POINT('Ctrl Pts',(96.018940331047,1.74304649795113,-0.344066903755196));
#23962=CARTESIAN_POINT('Ctrl Pts',(96.0277751294322,1.76467137305711,-0.22022774968932));
#23963=CARTESIAN_POINT('Ctrl Pts',(96.0340324368832,1.77329886426809,-0.133994673959963));
#23964=CARTESIAN_POINT('Ctrl Pts',(96.0403469426785,1.77561363837197,-0.0475422940912497));
#23965=CARTESIAN_POINT('Origin',(88.3562164250559,0.,0.));
#23966=CARTESIAN_POINT('',(96.9396785576437,1.77561363837197,-0.0475422940912381));
#23967=CARTESIAN_POINT('',(96.7921246220486,1.77561363841954,-0.0475422923145644));
#23968=CARTESIAN_POINT('',(88.3562164250559,1.77561363837197,-0.0475422940912398));
#23969=CARTESIAN_POINT('Ctrl Pts',(96.9396785576437,1.77561363837197,-0.0475422940912364));
#23970=CARTESIAN_POINT('Ctrl Pts',(96.9356232072411,1.77407956665634,-0.104836934843796));
#23971=CARTESIAN_POINT('Ctrl Pts',(96.9314956087136,1.76977293665518,-0.162037019091112));
#23972=CARTESIAN_POINT('Ctrl Pts',(96.9203869456945,1.75093773171991,-0.313679217648223));
#23973=CARTESIAN_POINT('Ctrl Pts',(96.9133474279507,1.73155256903901,-0.407312457551113));
#23974=CARTESIAN_POINT('Ctrl Pts',(96.9032963462726,1.69235891828376,-0.541227561636571));
#23975=CARTESIAN_POINT('Ctrl Pts',(96.9001618640205,1.6784100288131,-0.583049271579781));
#23976=CARTESIAN_POINT('Ctrl Pts',(96.8962234037238,1.6584755768458,-0.636146695932724));
#23977=CARTESIAN_POINT('Ctrl Pts',(96.8953517914793,1.6539061735443,-0.64793383143922));
#23978=CARTESIAN_POINT('Ctrl Pts',(96.8939565745305,1.64632941285726,-0.666876102598521));
#23979=CARTESIAN_POINT('Ctrl Pts',(96.8934285884521,1.64340041862677,-0.674061823398139));
#23980=CARTESIAN_POINT('Ctrl Pts',(96.8923965670982,1.63755149970169,-0.688146248823345));
#23981=CARTESIAN_POINT('Ctrl Pts',(96.8918923726934,1.63463486935379,-0.695046056870477));
#23982=CARTESIAN_POINT('Ctrl Pts',(96.8906286294507,1.62717751841793,-0.712381142724191));
#23983=CARTESIAN_POINT('Ctrl Pts',(96.8898724275367,1.62257989923515,-0.722791848643906));
#23984=CARTESIAN_POINT('Ctrl Pts',(96.8868220628516,1.60349758386567,-0.764901383893432));
#23985=CARTESIAN_POINT('Ctrl Pts',(96.8845728957466,1.58818052951521,-0.796217062990812));
#23986=CARTESIAN_POINT('Ctrl Pts',(96.8782783112472,1.54207879072632,-0.883839855467505));
#23987=CARTESIAN_POINT('Ctrl Pts',(96.8743160080936,1.50915069326266,-0.938959638045275));
#23988=CARTESIAN_POINT('Ctrl Pts',(96.8622380739791,1.39940510139645,-1.10192330390906));
#23989=CARTESIAN_POINT('Ctrl Pts',(96.8541870796653,1.31347879053693,-1.20305403662124));
#23990=CARTESIAN_POINT('Ctrl Pts',(96.8439816841957,1.19823149971852,-1.31147941733016));
#23991=CARTESIAN_POINT('Ctrl Pts',(96.8422929274682,1.17895161599672,-1.32883782466348));
#23992=CARTESIAN_POINT('Ctrl Pts',(96.8396152696973,1.14811150398895,-1.35540476904008));
#23993=CARTESIAN_POINT('Ctrl Pts',(96.8386383424385,1.13680424710619,-1.36490226579022));
#23994=CARTESIAN_POINT('Ctrl Pts',(96.8368092764201,1.11554103092052,-1.38231472511466));
#23995=CARTESIAN_POINT('Ctrl Pts',(96.8359586845422,1.10561587078853,-1.39026591797298));
#23996=CARTESIAN_POINT('Ctrl Pts',(96.8340489897373,1.08325654407973,-1.40778744865554));
#23997=CARTESIAN_POINT('Ctrl Pts',(96.8329877187508,1.07077935444391,-1.41730088103467));
#23998=CARTESIAN_POINT('Ctrl Pts',(96.8297841041277,1.03297298845034,-1.44534275452274));
#23999=CARTESIAN_POINT('Ctrl Pts',(96.8276226358796,1.00727834127237,-1.46336564074575));
#24000=CARTESIAN_POINT('Ctrl Pts',(96.8185664509998,0.898917599066307,-1.53516627141331));
#24001=CARTESIAN_POINT('Ctrl Pts',(96.811455655941,0.81233261622961,-1.58268724357425));
#24002=CARTESIAN_POINT('Ctrl Pts',(96.7959342835873,0.618097373257478,-1.66913755217854));
#24003=CARTESIAN_POINT('Ctrl Pts',(96.787527262531,0.509700516808075,-1.70536615208122));
#24004=CARTESIAN_POINT('Ctrl Pts',(96.7783701481369,0.382235149323251,-1.73471652008209));
#24005=CARTESIAN_POINT('Ctrl Pts',(96.7772064725435,0.365844861631656,-1.7382470200084));
#24006=CARTESIAN_POINT('Ctrl Pts',(96.7754547019485,0.340841890758904,-1.74326336792976));
#24007=CARTESIAN_POINT('Ctrl Pts',(96.7748579231204,0.332264672024242,-1.74491849675535));
#24008=CARTESIAN_POINT('Ctrl Pts',(96.7738258132042,0.317320833625288,-1.74768799218558));
#24009=CARTESIAN_POINT('Ctrl Pts',(96.7733889280089,0.310960023286738,-1.74883095138706));
#24010=CARTESIAN_POINT('Ctrl Pts',(96.7723529463956,0.295793426421174,-1.75147083497368));
#24011=CARTESIAN_POINT('Ctrl Pts',(96.7717556252265,0.286982412952275,-1.75293609127932));
#24012=CARTESIAN_POINT('Ctrl Pts',(96.7699447204414,0.260081762698165,-1.75720135335226));
#24013=CARTESIAN_POINT('Ctrl Pts',(96.7687422729645,0.24195894002122,-1.75978835517912));
#24014=CARTESIAN_POINT('Ctrl Pts',(96.7625597454069,0.147636856093194,-1.77176792695457));
#24015=CARTESIAN_POINT('Ctrl Pts',(96.7577851106945,0.0709192489455892,
-1.7764941094718));
#24016=CARTESIAN_POINT('Ctrl Pts',(96.7441089652802,-0.151044211140708,
-1.77576046135922));
#24017=CARTESIAN_POINT('Ctrl Pts',(96.735325674491,-0.29559556672042,-1.757486540941));
#24018=CARTESIAN_POINT('Ctrl Pts',(96.7243516674893,-0.46018271977652,-1.71578043049605));
#24019=CARTESIAN_POINT('Ctrl Pts',(96.7227455294568,-0.483927164842429,
-1.70923521602991));
#24020=CARTESIAN_POINT('Ctrl Pts',(96.7201786996517,-0.52127452056922,-1.69809974207909));
#24021=CARTESIAN_POINT('Ctrl Pts',(96.7192285837694,-0.534971580149367,
-1.69383448067292));
#24022=CARTESIAN_POINT('Ctrl Pts',(96.7174224905945,-0.560758845091712,
-1.6854603528706));
#24023=CARTESIAN_POINT('Ctrl Pts',(96.7165677019335,-0.572859391300981,
-1.68138609085725));
#24024=CARTESIAN_POINT('Ctrl Pts',(96.7146110089703,-0.600315581739159,
-1.67181078479785));
#24025=CARTESIAN_POINT('Ctrl Pts',(96.7135064496511,-0.615641290931902,
-1.66622803593303));
#24026=CARTESIAN_POINT('Ctrl Pts',(96.7100235335237,-0.663411453859677,
-1.64807761402416));
#24027=CARTESIAN_POINT('Ctrl Pts',(96.7076207609489,-0.695563154064766,
-1.63476792936696));
#24028=CARTESIAN_POINT('Ctrl Pts',(96.6937390335091,-0.876686123266674,
-1.55347876953772));
#24029=CARTESIAN_POINT('Ctrl Pts',(96.6815930563486,-1.01606866320442,-1.46610413578739));
#24030=CARTESIAN_POINT('Ctrl Pts',(96.6661110590931,-1.18011048251419,-1.32851252615373));
#24031=CARTESIAN_POINT('Ctrl Pts',(96.6625100550054,-1.21734797909129,-1.29447717529465));
#24032=CARTESIAN_POINT('Ctrl Pts',(96.6580900043349,-1.26241103564533,-1.24962210628938));
#24033=CARTESIAN_POINT('Ctrl Pts',(96.6571823650173,-1.27162924224538,-1.2402403507054));
#24034=CARTESIAN_POINT('Ctrl Pts',(96.6557437545782,-1.28619605233158,-1.22508192362801));
#24035=CARTESIAN_POINT('Ctrl Pts',(96.6552079220928,-1.29161173312698,-1.21937079740525));
#24036=CARTESIAN_POINT('Ctrl Pts',(96.6541728136703,-1.30205756909306,-1.2082074208869));
#24037=CARTESIAN_POINT('Ctrl Pts',(96.6536732582095,-1.30709179193982,-1.20275938366372));
#24038=CARTESIAN_POINT('Ctrl Pts',(96.6524385004021,-1.31951275176329,-1.18914732869402));
#24039=CARTESIAN_POINT('Ctrl Pts',(96.651706323875,-1.32685815605473,-1.18094568906797));
#24040=CARTESIAN_POINT('Ctrl Pts',(96.6488848347251,-1.35506155260926,-1.14885932101553));
#24041=CARTESIAN_POINT('Ctrl Pts',(96.6468324401498,-1.37535607572425,-1.12448455208884));
#24042=CARTESIAN_POINT('Ctrl Pts',(96.6412985837889,-1.42904987669197,-1.05636546342158));
#24043=CARTESIAN_POINT('Ctrl Pts',(96.6378781070863,-1.46108743043736,-1.01159077213557));
#24044=CARTESIAN_POINT('Ctrl Pts',(96.625895426446,-1.56668879639517,-0.848496135349694));
#24045=CARTESIAN_POINT('Ctrl Pts',(96.6174789699763,-1.62836431512253,-0.723108821659154));
#24046=CARTESIAN_POINT('Ctrl Pts',(96.6068065877054,-1.68374202177313,-0.566395027436137));
#24047=CARTESIAN_POINT('Ctrl Pts',(96.6050595035203,-1.69214216132003,-0.540782124792592));
#24048=CARTESIAN_POINT('Ctrl Pts',(96.6022195674877,-1.70470915709253,-0.49929903048888));
#24049=CARTESIAN_POINT('Ctrl Pts',(96.6011386633855,-1.70924474836109,-0.483544405806046));
#24050=CARTESIAN_POINT('Ctrl Pts',(96.5992026814816,-1.71692595921063,-0.455403734900474));
#24051=CARTESIAN_POINT('Ctrl Pts',(96.5983504495468,-1.72015725176205,-0.443042126367992));
#24052=CARTESIAN_POINT('Ctrl Pts',(96.5965353242905,-1.72672115443602,-0.4167763521796));
#24053=CARTESIAN_POINT('Ctrl Pts',(96.595571401331,-1.73001978891778,-0.402864719259183));
#24054=CARTESIAN_POINT('Ctrl Pts',(96.5929478934363,-1.7384916303543,-0.365111052016149));
#24055=CARTESIAN_POINT('Ctrl Pts',(96.5912781628921,-1.74334199502644,-0.341200548374984));
#24056=CARTESIAN_POINT('Ctrl Pts',(96.5817055613514,-1.7680890875309,-0.204849284669015));
#24057=CARTESIAN_POINT('Ctrl Pts',(96.5734788508433,-1.77759572881467,-0.0908146220477611));
#24058=CARTESIAN_POINT('Ctrl Pts',(96.5571171173897,-1.77465459210713,0.133152362411942));
#24059=CARTESIAN_POINT('Ctrl Pts',(96.5490302069568,-1.76302821151447,0.24261845888245));
#24060=CARTESIAN_POINT('Ctrl Pts',(96.5401427424422,-1.7380023145234,0.367018082674013));
#24061=CARTESIAN_POINT('Ctrl Pts',(96.5389597378287,-1.73440197901315,0.383671925961179));
#24062=CARTESIAN_POINT('Ctrl Pts',(96.5371849554004,-1.72858113267848,0.408838149382176));
#24063=CARTESIAN_POINT('Ctrl Pts',(96.5365841627788,-1.72653622047425,0.417389569006045));
#24064=CARTESIAN_POINT('Ctrl Pts',(96.5355482086114,-1.72287884313549,0.432197042775446));
#24065=CARTESIAN_POINT('Ctrl Pts',(96.5351114445457,-1.72129566806455,0.438459825230202));
#24066=CARTESIAN_POINT('Ctrl Pts',(96.5340796085663,-1.71745742429487,0.453302042837895));
#24067=CARTESIAN_POINT('Ctrl Pts',(96.5334862631617,-1.71517221410322,0.461873392487705));
#24068=CARTESIAN_POINT('Ctrl Pts',(96.5317001716538,-1.70805928496215,0.487771512037753));
#24069=CARTESIAN_POINT('Ctrl Pts',(96.5305181217489,-1.70303235320524,0.505043002069628));
#24070=CARTESIAN_POINT('Ctrl Pts',(96.5245505631103,-1.67606501526009,0.592711473787468));
#24071=CARTESIAN_POINT('Ctrl Pts',(96.519954996623,-1.65001653625175,0.661776890872312));
#24072=CARTESIAN_POINT('Ctrl Pts',(96.5068822695579,-1.56302711957404,0.85504869015209));
#24073=CARTESIAN_POINT('Ctrl Pts',(96.4985313059506,-1.4918003819241,0.974007725420844));
#24074=CARTESIAN_POINT('Ctrl Pts',(96.4877152114919,-1.38894045266001,1.10762581092684));
#24075=CARTESIAN_POINT('Ctrl Pts',(96.4857420444112,-1.36975760484689,1.13126232407069));
#24076=CARTESIAN_POINT('Ctrl Pts',(96.4827142410135,-1.33977131520348,1.1663290797827));
#24077=CARTESIAN_POINT('Ctrl Pts',(96.4816774162574,-1.32940720942422,1.17812866210799));
#24078=CARTESIAN_POINT('Ctrl Pts',(96.4797890995996,-1.31036930358091,1.19923229620853));
#24079=CARTESIAN_POINT('Ctrl Pts',(96.4789399092411,-1.30174934812967,1.20858364716928));
#24080=CARTESIAN_POINT('Ctrl Pts',(96.4770961581717,-1.28291336977222,1.22858254266602));
#24081=CARTESIAN_POINT('Ctrl Pts',(96.4761001779779,-1.27266366454852,1.23919689819363));
#24082=CARTESIAN_POINT('Ctrl Pts',(96.4732913139656,-1.24355764176133,1.26859641044473));
#24083=CARTESIAN_POINT('Ctrl Pts',(96.4714656991539,-1.2244102876338,1.28708654517838));
#24084=CARTESIAN_POINT('Ctrl Pts',(96.4633963602737,-1.13882490605257,1.366095794733));
#24085=CARTESIAN_POINT('Ctrl Pts',(96.4569667847527,-1.06827307513788,1.42194525163768));
#24086=CARTESIAN_POINT('Ctrl Pts',(96.4433371859864,-0.912941161386405,
1.52680127853941));
#24087=CARTESIAN_POINT('Ctrl Pts',(96.4361404218093,-0.827713155058399,
1.57463487062948));
#24088=CARTESIAN_POINT('Ctrl Pts',(96.4261688189721,-0.701580409632603,
1.6323422453525));
#24089=CARTESIAN_POINT('Ctrl Pts',(96.4232485465996,-0.663586414707914,
1.64815349117786));
#24090=CARTESIAN_POINT('Ctrl Pts',(96.4195336166109,-0.613482778854462,
1.66699019298297));
#24091=CARTESIAN_POINT('Ctrl Pts',(96.4186801307191,-0.601845341461083,
1.67122698344178));
#24092=CARTESIAN_POINT('Ctrl Pts',(96.417306757995,-0.582898082576699,1.67790143775753));
#24093=CARTESIAN_POINT('Ctrl Pts',(96.4167827245249,-0.575615275422439,
1.68041377938165));
#24094=CARTESIAN_POINT('Ctrl Pts',(96.4157518178152,-0.56117800374746,1.68528931496328));
#24095=CARTESIAN_POINT('Ctrl Pts',(96.4152448489529,-0.55402444100427,1.68765451138728));
#24096=CARTESIAN_POINT('Ctrl Pts',(96.4139644220206,-0.535827106669778,
1.69354295640146));
#24097=CARTESIAN_POINT('Ctrl Pts',(96.4131944978607,-0.524763260831761,
1.69700382183262));
#24098=CARTESIAN_POINT('Ctrl Pts',(96.4100038060226,-0.478445366633006,
1.71099614012119));
#24099=CARTESIAN_POINT('Ctrl Pts',(96.4076334123019,-0.442899790959773,
1.72054002336557));
#24100=CARTESIAN_POINT('Ctrl Pts',(96.4008339555867,-0.338578973672684,
1.74510198813008));
#24101=CARTESIAN_POINT('Ctrl Pts',(96.3965046475898,-0.269174501310736,
1.75714629565119));
#24102=CARTESIAN_POINT('Ctrl Pts',(96.3846705863581,-0.0776647030914143,
1.77876354208276));
#24103=CARTESIAN_POINT('Ctrl Pts',(96.3771914645592,0.044983665069589,1.77988877837057));
#24104=CARTESIAN_POINT('Ctrl Pts',(96.3677409052407,0.191008860547269,1.76611791284723));
#24105=CARTESIAN_POINT('Ctrl Pts',(96.3661583834715,0.21519832509185,1.76333390372538));
#24106=CARTESIAN_POINT('Ctrl Pts',(96.3635334544907,0.2548285964531,1.75794520631995));
#24107=CARTESIAN_POINT('Ctrl Pts',(96.3625001708429,0.270306194993132,1.75563193658893));
#24108=CARTESIAN_POINT('Ctrl Pts',(96.3606155653953,0.298300232662472,1.75106901804026));
#24109=CARTESIAN_POINT('Ctrl Pts',(96.3597665013136,0.31082704559568,1.74888886668231));
#24110=CARTESIAN_POINT('Ctrl Pts',(96.3579198721308,0.337880542826909,1.74388067319088));
#24111=CARTESIAN_POINT('Ctrl Pts',(96.3569208516996,0.352397356328795,1.74100521069526));
#24112=CARTESIAN_POINT('Ctrl Pts',(96.3540941761324,0.393127212887685,1.7324072507934));
#24113=CARTESIAN_POINT('Ctrl Pts',(96.3522535279206,0.4192480019455,1.72627195541064));
#24114=CARTESIAN_POINT('Ctrl Pts',(96.3440523731365,0.533819771847705,1.69660747711912));
#24115=CARTESIAN_POINT('Ctrl Pts',(96.3374987069675,0.620502449168482,1.66685714959223));
#24116=CARTESIAN_POINT('Ctrl Pts',(96.3235070215871,0.797011289586751,1.59059541409464));
#24117=CARTESIAN_POINT('Ctrl Pts',(96.3160705031135,0.885956855749489,1.54282270175741));
#24118=CARTESIAN_POINT('Ctrl Pts',(96.3062131562096,1.00118573274527,1.46766637619235));
#24119=CARTESIAN_POINT('Ctrl Pts',(96.3036096164551,1.03137014099969,1.44661450672097));
#24120=CARTESIAN_POINT('Ctrl Pts',(96.3002303851703,1.07046138216396,1.41750455676896));
#24121=CARTESIAN_POINT('Ctrl Pts',(96.2994078450249,1.0799697658581,1.41027375486372));
#24122=CARTESIAN_POINT('Ctrl Pts',(96.2981232201638,1.09481969916538,1.39874261022068));
#24123=CARTESIAN_POINT('Ctrl Pts',(96.2976568923052,1.10021032251459,1.39450647671594));
#24124=CARTESIAN_POINT('Ctrl Pts',(96.2966887355916,1.11140468636307,1.38560424972168));
#24125=CARTESIAN_POINT('Ctrl Pts',(96.2961873526501,1.11720382714097,1.38093270114255));
#24126=CARTESIAN_POINT('Ctrl Pts',(96.2949409812768,1.13161898218803,1.36917020583847));
#24127=CARTESIAN_POINT('Ctrl Pts',(96.2941991468169,1.14019807023773,1.36203412219907));
#24128=CARTESIAN_POINT('Ctrl Pts',(96.2912880446905,1.17383069700094,1.33351801322075));
#24129=CARTESIAN_POINT('Ctrl Pts',(96.2891587559039,1.1983564231411,1.31152239921838));
#24130=CARTESIAN_POINT('Ctrl Pts',(96.2833354685803,1.26467847131537,1.24862734835433));
#24131=CARTESIAN_POINT('Ctrl Pts',(96.2797104551052,1.3050900172544,1.20632618976675));
#24132=CARTESIAN_POINT('Ctrl Pts',(96.2673226776806,1.43669522453664,1.05419633114055));
#24133=CARTESIAN_POINT('Ctrl Pts',(96.2586804255489,1.51669502649027,0.935443912564588));
#24134=CARTESIAN_POINT('Ctrl Pts',(96.2478686974002,1.59286224310267,0.786424385262114));
#24135=CARTESIAN_POINT('Ctrl Pts',(96.2462595860244,1.60363719519756,0.764212724515875));
#24136=CARTESIAN_POINT('Ctrl Pts',(96.2436803695459,1.61999837073896,0.728614730398607));
#24137=CARTESIAN_POINT('Ctrl Pts',(96.2427207925812,1.62588978183821,0.715371611745342));
#24138=CARTESIAN_POINT('Ctrl Pts',(96.2409918423764,1.63615184356162,0.691522067783552));
#24139=CARTESIAN_POINT('Ctrl Pts',(96.2402245927433,1.64058311021227,0.680942488945931));
#24140=CARTESIAN_POINT('Ctrl Pts',(96.2384157300193,1.65074135086279,0.656015016335219));
#24141=CARTESIAN_POINT('Ctrl Pts',(96.2373713403672,1.65638414220848,0.641634051628717));
#24142=CARTESIAN_POINT('Ctrl Pts',(96.2342725213628,1.67247030227617,0.59901067821534));
#24143=CARTESIAN_POINT('Ctrl Pts',(96.2322007862062,1.68238347140754,0.570575470139431));
#24144=CARTESIAN_POINT('Ctrl Pts',(96.2273542462392,1.70363730076587,0.504230979717622));
#24145=CARTESIAN_POINT('Ctrl Pts',(96.2245640897837,1.71444323059226,0.466168368994196));
#24146=CARTESIAN_POINT('Ctrl Pts',(96.2103175552787,1.76253107758018,0.272372181807902));
#24147=CARTESIAN_POINT('Ctrl Pts',(96.1983478358472,1.77989868591278,0.112495978105697));
#24148=CARTESIAN_POINT('Ctrl Pts',(96.1869838792615,1.77561363799549,-0.047542308152177));
#24149=CARTESIAN_POINT('Ctrl Pts',(96.0403469426785,1.77561363837197,-0.0475422940912497));
#24150=CARTESIAN_POINT('Ctrl Pts',(96.0433876696981,1.77672830932013,-0.00591146882942374));
#24151=CARTESIAN_POINT('Ctrl Pts',(96.0464401059596,1.77637919693629,0.0357703223646982));
#24152=CARTESIAN_POINT('Ctrl Pts',(96.0546368358133,1.77148391667716,0.147967372245616));
#24153=CARTESIAN_POINT('Ctrl Pts',(96.0597534565257,1.7642023552637,0.218269494084479));
#24154=CARTESIAN_POINT('Ctrl Pts',(96.0659341402809,1.74990412066124,0.305300748148632));
#24155=CARTESIAN_POINT('Ctrl Pts',(96.0671549786533,1.74679738129867,0.322601837170153));
#24156=CARTESIAN_POINT('Ctrl Pts',(96.0689631289445,1.7417622012224,0.348432004388496));
#24157=CARTESIAN_POINT('Ctrl Pts',(96.0695602857837,1.74002688401859,0.356997028436484));
#24158=CARTESIAN_POINT('Ctrl Pts',(96.070588108326,1.73691281003247,0.371804810633909));
#24159=CARTESIAN_POINT('Ctrl Pts',(96.0710203752537,1.73556349610133,0.378053278305842));
#24160=CARTESIAN_POINT('Ctrl Pts',(96.0720385473342,1.7322911826648,0.392820024996573));
#24161=CARTESIAN_POINT('Ctrl Pts',(96.0726227983545,1.73033906837447,0.401331571240553));
#24162=CARTESIAN_POINT('Ctrl Pts',(96.0743707824079,1.72427664982682,0.426897929467039));
#24163=CARTESIAN_POINT('Ctrl Pts',(96.0755243800255,1.71997625030062,0.443907155502213));
#24164=CARTESIAN_POINT('Ctrl Pts',(96.0853751304822,1.68072435477487,0.590014484111818));
#24165=CARTESIAN_POINT('Ctrl Pts',(96.0934208631937,1.63154246615937,0.714864172440539));
#24166=CARTESIAN_POINT('Ctrl Pts',(96.1070040804877,1.52813008816765,0.909617282520516));
#24167=CARTESIAN_POINT('Ctrl Pts',(96.112404552365,1.4819079180233,0.983123405205661));
#24168=CARTESIAN_POINT('Ctrl Pts',(96.1196814438005,1.41503649597352,1.07397244150562));
#24169=CARTESIAN_POINT('Ctrl Pts',(96.121380762951,1.39910597314861,1.09464489762381));
#24170=CARTESIAN_POINT('Ctrl Pts',(96.1240558468793,1.37358794487497,1.1262913368892));
#24171=CARTESIAN_POINT('Ctrl Pts',(96.1250192586575,1.36431065498018,1.13751150910192));
#24172=CARTESIAN_POINT('Ctrl Pts',(96.1268265678247,1.34675290542148,1.15822246489308));
#24173=CARTESIAN_POINT('Ctrl Pts',(96.1276689986667,1.33850734416403,1.16774172742074));
#24174=CARTESIAN_POINT('Ctrl Pts',(96.1295647570431,1.31981993366253,1.18885781453425));
#24175=CARTESIAN_POINT('Ctrl Pts',(96.1306202658558,1.30932519381584,1.20040621048101));
#24176=CARTESIAN_POINT('Ctrl Pts',(96.1338209049152,1.27724161463002,1.23478960843855));
#24177=CARTESIAN_POINT('Ctrl Pts',(96.135985300139,1.25519864763659,1.25719038166149));
#24178=CARTESIAN_POINT('Ctrl Pts',(96.1477549634364,1.13355718658271,1.37441704113651));
#24179=CARTESIAN_POINT('Ctrl Pts',(96.157821035613,1.02380768668753,1.4580053342488));
#24180=CARTESIAN_POINT('Ctrl Pts',(96.1732379316871,0.842205515268603,1.56562277283818));
#24181=CARTESIAN_POINT('Ctrl Pts',(96.1785816332144,0.776587420662064,1.59918693063103));
#24182=CARTESIAN_POINT('Ctrl Pts',(96.184999997342,0.692655181488947,1.63573022676487));
#24183=CARTESIAN_POINT('Ctrl Pts',(96.1862440509095,0.676132737364651,1.64262873409602));
#24184=CARTESIAN_POINT('Ctrl Pts',(96.1880794531956,0.651335127631088,1.65254473206552));
#24185=CARTESIAN_POINT('Ctrl Pts',(96.1886810694911,0.643137810137824,1.65575218720448));
#24186=CARTESIAN_POINT('Ctrl Pts',(96.1897135534512,0.628944183604309,1.66118456939699));
#24187=CARTESIAN_POINT('Ctrl Pts',(96.1901460725971,0.622959349878934,1.66343818991849));
#24188=CARTESIAN_POINT('Ctrl Pts',(96.1911605071167,0.608830551604378,1.66867151256132));
#24189=CARTESIAN_POINT('Ctrl Pts',(96.1917408189518,0.600676784961151,1.67162396049337));
#24190=CARTESIAN_POINT('Ctrl Pts',(96.1934646049107,0.576255166025127,1.68026516813738));
#24191=CARTESIAN_POINT('Ctrl Pts',(96.1945983531944,0.559925278218729,1.68577720611461));
#24192=CARTESIAN_POINT('Ctrl Pts',(96.2045386443326,0.414666030370205,1.73246466599179));
#24193=CARTESIAN_POINT('Ctrl Pts',(96.2126743007798,0.281485631032072,1.75902191816467));
#24194=CARTESIAN_POINT('Ctrl Pts',(96.2248460825533,0.0846217228168619,
1.77532154072611));
#24195=CARTESIAN_POINT('Ctrl Pts',(96.2287060933793,0.0224549346748234,
1.77719508028112));
#24196=CARTESIAN_POINT('Ctrl Pts',(96.2344516118664,-0.0680520708919391,
1.77517278840987));
#24197=CARTESIAN_POINT('Ctrl Pts',(96.2362691830766,-0.0964049428039959,
1.7738589203888));
#24198=CARTESIAN_POINT('Ctrl Pts',(96.2396191519547,-0.148019174782241,
1.77022604542378));
#24199=CARTESIAN_POINT('Ctrl Pts',(96.2411448299046,-0.171289706317521,
1.76812603663042));
#24200=CARTESIAN_POINT('Ctrl Pts',(96.2436070434258,-0.208418346636026,
1.7640356038368));
#24201=CARTESIAN_POINT('Ctrl Pts',(96.2445343259482,-0.222306562133279,
1.76233923871774));
#24202=CARTESIAN_POINT('Ctrl Pts',(96.2463121651587,-0.248744028302583,
1.75879258206465));
#24203=CARTESIAN_POINT('Ctrl Pts',(96.2471617438501,-0.261296381246172,
1.75697157775804));
#24204=CARTESIAN_POINT('Ctrl Pts',(96.2491095719971,-0.289883074080024,
1.75251131530876));
#24205=CARTESIAN_POINT('Ctrl Pts',(96.250210481592,-0.305902653254055,1.74978617064578));
#24206=CARTESIAN_POINT('Ctrl Pts',(96.2537739408441,-0.35729954370982,1.74031551234671));
#24207=CARTESIAN_POINT('Ctrl Pts',(96.2562631869044,-0.392507867695139,
1.73271414088731));
#24208=CARTESIAN_POINT('Ctrl Pts',(96.2680562970163,-0.556012279196441,
1.69217503082626));
#24209=CARTESIAN_POINT('Ctrl Pts',(96.2777641414023,-0.680581183691712,
1.64602699985076));
#24210=CARTESIAN_POINT('Ctrl Pts',(96.2926867390598,-0.86313744528844,1.5541041965456));
#24211=CARTESIAN_POINT('Ctrl Pts',(96.2979070116048,-0.925411846684418,
1.51784748875361));
#24212=CARTESIAN_POINT('Ctrl Pts',(96.3041963347968,-1.00006800558042,1.46807434499025));
#24213=CARTESIAN_POINT('Ctrl Pts',(96.3054278745845,-1.01466997481802,1.45802030169281));
#24214=CARTESIAN_POINT('Ctrl Pts',(96.3072485941074,-1.03626610921513,1.44266887800989));
#24215=CARTESIAN_POINT('Ctrl Pts',(96.3078478126449,-1.04337504487847,1.43753590028861));
#24216=CARTESIAN_POINT('Ctrl Pts',(96.3088777837763,-1.05560161226745,1.42856927621761));
#24217=CARTESIAN_POINT('Ctrl Pts',(96.3093101608457,-1.0607368512459,1.42476042781098));
#24218=CARTESIAN_POINT('Ctrl Pts',(96.3103265740201,-1.07281431573213,1.41570097896848));
#24219=CARTESIAN_POINT('Ctrl Pts',(96.3109089796608,-1.07973864910677,1.41042698339383));
#24220=CARTESIAN_POINT('Ctrl Pts',(96.312645604051,-1.10038632688025,1.39445927286749));
#24221=CARTESIAN_POINT('Ctrl Pts',(96.3137898806864,-1.11399206816059,1.38361427421799));
#24222=CARTESIAN_POINT('Ctrl Pts',(96.3236830509232,-1.23137028798669,1.28719917402009));
#24223=CARTESIAN_POINT('Ctrl Pts',(96.3317713689111,-1.32528550275458,1.19028701106267));
#24224=CARTESIAN_POINT('Ctrl Pts',(96.3453768613518,-1.46001872358041,1.01531125352363));
#24225=CARTESIAN_POINT('Ctrl Pts',(96.3507522415374,-1.50761113602867,0.943195547056151));
#24226=CARTESIAN_POINT('Ctrl Pts',(96.3579985654031,-1.56249522315527,0.845192756360054));
#24227=CARTESIAN_POINT('Ctrl Pts',(96.3596942673656,-1.57471695663431,0.822197367381114));
#24228=CARTESIAN_POINT('Ctrl Pts',(96.3623649211322,-1.59297145358098,0.785950142298659));
#24229=CARTESIAN_POINT('Ctrl Pts',(96.363327588463,-1.59935455688939,0.772878165226385));
#24230=CARTESIAN_POINT('Ctrl Pts',(96.365134230964,-1.61096321881567,0.74834497333285));
#24231=CARTESIAN_POINT('Ctrl Pts',(96.3659767492329,-1.61622884697976,0.736903651485344));
#24232=CARTESIAN_POINT('Ctrl Pts',(96.3678736692495,-1.62775133562321,0.711149517456909));
#24233=CARTESIAN_POINT('Ctrl Pts',(96.3689302643824,-1.63394189280763,0.69680837430314));
#24234=CARTESIAN_POINT('Ctrl Pts',(96.3716628616095,-1.64936603126019,0.659740454729706));
#24235=CARTESIAN_POINT('Ctrl Pts',(96.3733480820901,-1.65831913977624,0.636901325841086));
#24236=CARTESIAN_POINT('Ctrl Pts',(96.3828308320086,-1.70559024865233,0.508552713885142));
#24237=CARTESIAN_POINT('Ctrl Pts',(96.3909356923378,-1.73430634666039,0.399797134784209));
#24238=CARTESIAN_POINT('Ctrl Pts',(96.4048153245524,-1.7652170892738,0.212397340106992));
#24239=CARTESIAN_POINT('Ctrl Pts',(96.4105192306627,-1.77281950760008,0.134966303210488));
#24240=CARTESIAN_POINT('Ctrl Pts',(96.4188796824323,-1.77657836423367,0.0184727949455617));
#24241=CARTESIAN_POINT('Ctrl Pts',(96.4216299180277,-1.77655774068567,-0.020372277207449));
#24242=CARTESIAN_POINT('Ctrl Pts',(96.4251344145167,-1.77487271739594,-0.0709118418405051));
#24243=CARTESIAN_POINT('Ctrl Pts',(96.4259418866715,-1.77436572233193,-0.0826314368179974));
#24244=CARTESIAN_POINT('Ctrl Pts',(96.4272564624798,-1.77334359385232,-0.101847955948175));
#24245=CARTESIAN_POINT('Ctrl Pts',(96.4277671680262,-1.7728969338977,-0.109347956134689));
#24246=CARTESIAN_POINT('Ctrl Pts',(96.4287250655545,-1.77196497090298,-0.123484739922586));
#24247=CARTESIAN_POINT('Ctrl Pts',(96.4291728358794,-1.77148993859981,-0.130122020595905));
#24248=CARTESIAN_POINT('Ctrl Pts',(96.4303630914379,-1.77012193802916,-0.147837422565275));
#24249=CARTESIAN_POINT('Ctrl Pts',(96.4311019554302,-1.76916226152398,-0.158910311858289));
#24250=CARTESIAN_POINT('Ctrl Pts',(96.4338576862862,-1.76516804958806,-0.200458834120121));
#24251=CARTESIAN_POINT('Ctrl Pts',(96.4358406527299,-1.76144927286057,-0.230865134721124));
#24252=CARTESIAN_POINT('Ctrl Pts',(96.4454400694956,-1.73934312049414,-0.379582379965967));
#24253=CARTESIAN_POINT('Ctrl Pts',(96.4526573165571,-1.70981173014821,-0.495929869578268));
#24254=CARTESIAN_POINT('Ctrl Pts',(96.4637288019037,-1.64833128176214,-0.664557910971128));
#24255=CARTESIAN_POINT('Ctrl Pts',(96.4674452769705,-1.62504982414338,-0.719614846062477));
#24256=CARTESIAN_POINT('Ctrl Pts',(96.4738015453543,-1.58148570479922,-0.809686700392552));
#24257=CARTESIAN_POINT('Ctrl Pts',(96.4763962804471,-1.56270156170168,-0.845371532595011));
#24258=CARTESIAN_POINT('Ctrl Pts',(96.4801534427757,-1.5342314550302,-0.895260447356261));
#24259=CARTESIAN_POINT('Ctrl Pts',(96.4812811005627,-1.52552769655476,-0.910012439086788));
#24260=CARTESIAN_POINT('Ctrl Pts',(96.4832628764201,-1.50996609696092,-0.935536987169152));
#24261=CARTESIAN_POINT('Ctrl Pts',(96.484113496306,-1.50320278989333,-0.946365905034824));
#24262=CARTESIAN_POINT('Ctrl Pts',(96.4858873889435,-1.48892937979577,-0.968680371648061));
#24263=CARTESIAN_POINT('Ctrl Pts',(96.4868112745153,-1.48140175994041,-0.980153644933));
#24264=CARTESIAN_POINT('Ctrl Pts',(96.4892349744694,-1.46141612195033,-1.00985867771676));
#24265=CARTESIAN_POINT('Ctrl Pts',(96.4907425631872,-1.44875006570373,-1.02794688618169));
#24266=CARTESIAN_POINT('Ctrl Pts',(96.49818793437,-1.38508582745041,-1.11535033611063));
#24267=CARTESIAN_POINT('Ctrl Pts',(96.5043037030689,-1.32944107081139,-1.18112303845155));
#24268=CARTESIAN_POINT('Ctrl Pts',(96.5118167459577,-1.25688101990635,-1.25523988945663));
#24269=CARTESIAN_POINT('Ctrl Pts',(96.5131024092744,-1.24431617937507,-1.26769645646042));
#24270=CARTESIAN_POINT('Ctrl Pts',(96.5221645659548,-1.15466056927883,-1.3539621794663));
#24271=CARTESIAN_POINT('Ctrl Pts',(96.530043952294,-1.07123923731331,-1.42088091225778));
#24272=CARTESIAN_POINT('Ctrl Pts',(96.5397276826587,-0.957863715944365,
-1.49613578613419));
#24273=CARTESIAN_POINT('Ctrl Pts',(96.5417919842727,-0.933014410136437,
-1.51175710276556));
#24274=CARTESIAN_POINT('Ctrl Pts',(96.5445784839781,-0.898387234334779,
-1.5323459308134));
#24275=CARTESIAN_POINT('Ctrl Pts',(96.5453301387442,-0.888934962664311,
-1.53784860176916));
#24276=CARTESIAN_POINT('Ctrl Pts',(96.5465730130397,-0.873108762295881,
-1.54686719589485));
#24277=CARTESIAN_POINT('Ctrl Pts',(96.5470672177115,-0.866763066909204,
-1.55043181908437));
#24278=CARTESIAN_POINT('Ctrl Pts',(96.5480822799548,-0.853616688444252,
-1.55771070791429));
#24279=CARTESIAN_POINT('Ctrl Pts',(96.5486028097194,-0.846813321125198,
-1.56141964419779));
#24280=CARTESIAN_POINT('Ctrl Pts',(96.5499772098976,-0.82869249927194,-1.57114514878173));
#24281=CARTESIAN_POINT('Ctrl Pts',(96.5508263816818,-0.817333581725103,
-1.57708407407204));
#24282=CARTESIAN_POINT('Ctrl Pts',(96.5551020271408,-0.759374605681323,
-1.60659306537321));
#24283=CARTESIAN_POINT('Ctrl Pts',(96.5584248076811,-0.711811154827843,
-1.62822512342973));
#24284=CARTESIAN_POINT('Ctrl Pts',(96.5714322160051,-0.519039592306961,
-1.7058328833121));
#24285=CARTESIAN_POINT('Ctrl Pts',(96.5806989043514,-0.367715596809096,
-1.74472237467166));
#24286=CARTESIAN_POINT('Ctrl Pts',(96.5930611443431,-0.174662267186891,
-1.76806910819083));
#24287=CARTESIAN_POINT('Ctrl Pts',(96.5955637586065,-0.135928738473593,
-1.77146783994708));
#24288=CARTESIAN_POINT('Ctrl Pts',(96.5991229796369,-0.0815787027146657,
-1.774443896111));
#24289=CARTESIAN_POINT('Ctrl Pts',(96.6001465887385,-0.0660303159480231,
-1.77509047577077));
#24290=CARTESIAN_POINT('Ctrl Pts',(96.6020282643681,-0.0376133813468859,
-1.77589832832862));
#24291=CARTESIAN_POINT('Ctrl Pts',(96.6028842613908,-0.0247476284584036,
-1.77612420146555));
#24292=CARTESIAN_POINT('Ctrl Pts',(96.6046319301138,0.00138780180533268,
-1.77629901797108));
#24293=CARTESIAN_POINT('Ctrl Pts',(96.605523824763,0.0146566984927439,-1.77623908633274));
#24294=CARTESIAN_POINT('Ctrl Pts',(96.6077640674554,0.0478053536630558,
-1.77571791160041));
#24295=CARTESIAN_POINT('Ctrl Pts',(96.6091181104532,0.0676799444655246,
-1.77507149782045));
#24296=CARTESIAN_POINT('Ctrl Pts',(96.6147739406371,0.150001128646456,-1.77100953250991));
#24297=CARTESIAN_POINT('Ctrl Pts',(96.6191659716135,0.212249872353845,-1.76463126019965));
#24298=CARTESIAN_POINT('Ctrl Pts',(96.6331581257644,0.405555032149858,-1.73444822129257));
#24299=CARTESIAN_POINT('Ctrl Pts',(96.6430303293577,0.534342874064152,-1.69919340268804));
#24300=CARTESIAN_POINT('Ctrl Pts',(96.655876815425,0.699883962047843,-1.63317543163726));
#24301=CARTESIAN_POINT('Ctrl Pts',(96.6590881093104,0.741142795399371,-1.61487078335525));
#24302=CARTESIAN_POINT('Ctrl Pts',(96.6631040800162,0.793064946139255,-1.58942545474513));
#24303=CARTESIAN_POINT('Ctrl Pts',(96.6639797182553,0.804406910224268,-1.58371551458119));
#24304=CARTESIAN_POINT('Ctrl Pts',(96.6653764441158,0.822547079259722,-1.57433795632047));
#24305=CARTESIAN_POINT('Ctrl Pts',(96.6659019966978,0.829384054015543,-1.57074689081819));
#24306=CARTESIAN_POINT('Ctrl Pts',(96.6669243759083,0.842710641585863,-1.56363593437802));
#24307=CARTESIAN_POINT('Ctrl Pts',(96.6674214063263,0.849202070046048,-1.56011999787408));
#24308=CARTESIAN_POINT('Ctrl Pts',(96.6686593057921,0.865395468100679,-1.55121819094696));
#24309=CARTESIAN_POINT('Ctrl Pts',(96.6693970401735,0.875069456169091,-1.54578156760805));
#24310=CARTESIAN_POINT('Ctrl Pts',(96.6723066555768,0.913283222007781,-1.52383232481876));
#24311=CARTESIAN_POINT('Ctrl Pts',(96.6744383799482,0.941413649170928,-1.50661603066987));
#24312=CARTESIAN_POINT('Ctrl Pts',(96.6802815351733,1.01827539865973,-1.45658133462302));
#24313=CARTESIAN_POINT('Ctrl Pts',(96.6839230924121,1.06588414887998,-1.42211318219492));
#24314=CARTESIAN_POINT('Ctrl Pts',(96.69631499456,1.22283334070916,-1.29616607858894));
#24315=CARTESIAN_POINT('Ctrl Pts',(96.7049467586127,1.32282044426029,-1.19394722468504));
#24316=CARTESIAN_POINT('Ctrl Pts',(96.7157432994021,1.42451295597466,-1.06133588654701));
#24317=CARTESIAN_POINT('Ctrl Pts',(96.7173492678694,1.4390958717733,-1.04147683657097));
#24318=CARTESIAN_POINT('Ctrl Pts',(96.7199187398832,1.46153734585777,-1.00954438249589));
#24319=CARTESIAN_POINT('Ctrl Pts',(96.7208717053221,1.46967050890309,-0.997667203171026));
#24320=CARTESIAN_POINT('Ctrl Pts',(96.7226618598118,1.48458956479065,-0.975301952876253));
#24321=CARTESIAN_POINT('Ctrl Pts',(96.7234976402743,1.49141095618452,-0.964838546688172));
#24322=CARTESIAN_POINT('Ctrl Pts',(96.725398302095,1.50659549054344,-0.941000999097562));
#24323=CARTESIAN_POINT('Ctrl Pts',(96.7264655730623,1.51489187641334,-0.927585805821953));
#24324=CARTESIAN_POINT('Ctrl Pts',(96.7297408577931,1.53964693316766,-0.886338992089204));
#24325=CARTESIAN_POINT('Ctrl Pts',(96.7319694919433,1.55552450219238,-0.858168266225254));
#24326=CARTESIAN_POINT('Ctrl Pts',(96.7403645968453,1.61174598138914,-0.75172569841525));
#24327=CARTESIAN_POINT('Ctrl Pts',(96.7466945303134,1.64701713193903,-0.670930299409452));
#24328=CARTESIAN_POINT('Ctrl Pts',(96.7611247440834,1.71255543260793,-0.484063713797703));
#24329=CARTESIAN_POINT('Ctrl Pts',(96.7692472197254,1.73924085386397,-0.377103476463024));
#24330=CARTESIAN_POINT('Ctrl Pts',(96.7788481038222,1.75970956422427,-0.24317732411605));
#24331=CARTESIAN_POINT('Ctrl Pts',(96.7806338299924,1.7630162474474,-0.217914742085545));
#24332=CARTESIAN_POINT('Ctrl Pts',(96.7831088341323,1.76690185795227,-0.182288854331869));
#24333=CARTESIAN_POINT('Ctrl Pts',(96.7838199674651,1.7679350852835,-0.171979502887705));
#24334=CARTESIAN_POINT('Ctrl Pts',(96.7850202134992,1.76953761293301,-0.154444852038142));
#24335=CARTESIAN_POINT('Ctrl Pts',(96.7855117906169,1.7701529981727,-0.147224138254561));
#24336=CARTESIAN_POINT('Ctrl Pts',(96.7865394568458,1.77135327007756,-0.132043011563271));
#24337=CARTESIAN_POINT('Ctrl Pts',(96.7870750331009,1.77192872025303,-0.124082153946712));
#24338=CARTESIAN_POINT('Ctrl Pts',(96.7885351515605,1.77335877469186,-0.102253395420015));
#24339=CARTESIAN_POINT('Ctrl Pts',(96.7894539095615,1.77410438136053,-0.0883785851909835));
#24340=CARTESIAN_POINT('Ctrl Pts',(96.7909547797782,1.77506420704411,-0.0655130360673177));
#24341=CARTESIAN_POINT('Ctrl Pts',(96.7915411706753,1.77537303872842,-0.0565282306894022));
#24342=CARTESIAN_POINT('Ctrl Pts',(96.7921246220486,1.77561363846711,-0.047542290537889));
#24343=CARTESIAN_POINT('Origin',(88.3562164250559,0.,0.));
#24344=CARTESIAN_POINT('',(97.6892780533294,1.77561363837197,-0.0475422940912403));
#24345=CARTESIAN_POINT('',(97.5395352881717,1.77561363837197,-0.0475422940912395));
#24346=CARTESIAN_POINT('',(88.3562164250559,1.77561363837197,-0.0475422940912398));
#24347=CARTESIAN_POINT('Ctrl Pts',(97.6892780533294,1.77561363837197,-0.0475422940912433));
#24348=CARTESIAN_POINT('Ctrl Pts',(97.6872059749121,1.77472582019844,-0.080700602655293));
#24349=CARTESIAN_POINT('Ctrl Pts',(97.6851152451758,1.77290879404315,-0.113849259557775));
#24350=CARTESIAN_POINT('Ctrl Pts',(97.6806364708754,1.7670940076383,-0.183894415182408));
#24351=CARTESIAN_POINT('Ctrl Pts',(97.6782450379417,1.76287138399518,-0.220731882255648));
#24352=CARTESIAN_POINT('Ctrl Pts',(97.6747361193426,1.75510518458071,-0.273756943199008));
#24353=CARTESIAN_POINT('Ctrl Pts',(97.6736474005101,1.75248279157628,-0.290070866414429));
#24354=CARTESIAN_POINT('Ctrl Pts',(97.6717006908093,1.74742110409714,-0.318979729331859));
#24355=CARTESIAN_POINT('Ctrl Pts',(97.6708456224853,1.74507220682892,-0.331589446336467));
#24356=CARTESIAN_POINT('Ctrl Pts',(97.669042604046,1.73985854588832,-0.357986854608185));
#24357=CARTESIAN_POINT('Ctrl Pts',(97.668093819272,1.73696598277814,-0.371768076281808));
#24358=CARTESIAN_POINT('Ctrl Pts',(97.6655566998686,1.72883910770633,-0.408320061348677));
#24359=CARTESIAN_POINT('Ctrl Pts',(97.6639593385852,1.72331900063188,-0.431023739565304));
#24360=CARTESIAN_POINT('Ctrl Pts',(97.6603949302854,1.71012270780295,-0.480984368508529));
#24361=CARTESIAN_POINT('Ctrl Pts',(97.6584217520089,1.70223942238302,-0.508179528390899));
#24362=CARTESIAN_POINT('Ctrl Pts',(97.6520898680133,1.67512629676021,-0.59398680048482));
#24363=CARTESIAN_POINT('Ctrl Pts',(97.6476633667186,1.65349353828367,-0.651786997527286));
#24364=CARTESIAN_POINT('Ctrl Pts',(97.6335112575606,1.57575405025281,-0.830556815984747));
#24365=CARTESIAN_POINT('Ctrl Pts',(97.6236126737745,1.50902138815495,-0.946404820769795));
#24366=CARTESIAN_POINT('Ctrl Pts',(97.6129231006762,1.4187223644381,-1.06894789901965));
#24367=CARTESIAN_POINT('Ctrl Pts',(97.6116053584319,1.40724356906661,-1.08401492949707));
#24368=CARTESIAN_POINT('Ctrl Pts',(97.6096801718675,1.38992531466666,-1.10600796578824));
#24369=CARTESIAN_POINT('Ctrl Pts',(97.6090611096744,1.38427077678759,-1.11307700823375));
#24370=CARTESIAN_POINT('Ctrl Pts',(97.6079582936657,1.37403887302606,-1.12566988621387));
#24371=CARTESIAN_POINT('Ctrl Pts',(97.6074731939136,1.36948182745627,-1.13120955020389));
#24372=CARTESIAN_POINT('Ctrl Pts',(97.6063863084202,1.35914454050102,-1.14362179648143));
#24373=CARTESIAN_POINT('Ctrl Pts',(97.6057858764029,1.35334560902482,-1.15047832078638));
#24374=CARTESIAN_POINT('Ctrl Pts',(97.603955411395,1.33540497343696,-1.17136755068604));
#24375=CARTESIAN_POINT('Ctrl Pts',(97.6027368675409,1.32309474437322,-1.18525471775049));
#24376=CARTESIAN_POINT('Ctrl Pts',(97.5998748291708,1.29337237119081,-1.21774423169152));
#24377=CARTESIAN_POINT('Ctrl Pts',(97.5982426183236,1.27577286867829,-1.23617022497075));
#24378=CARTESIAN_POINT('Ctrl Pts',(97.5920008791105,1.20624964612288,-1.30589134202646));
#24379=CARTESIAN_POINT('Ctrl Pts',(97.5875181803793,1.15157744389617,-1.3543490075586));
#24380=CARTESIAN_POINT('Ctrl Pts',(97.5757606191815,1.00069315986174,-1.47232075007208));
#24381=CARTESIAN_POINT('Ctrl Pts',(97.5685006649299,0.900247588891457,-1.53579477853656));
#24382=CARTESIAN_POINT('Ctrl Pts',(97.5592883796332,0.772338233827302,-1.59973653764129));
#24383=CARTESIAN_POINT('Ctrl Pts',(97.5576974749325,0.750218651166703,-1.61022831287166));
#24384=CARTESIAN_POINT('Ctrl Pts',(97.5550615636616,0.713580035458728,-1.62668795506153));
#24385=CARTESIAN_POINT('Ctrl Pts',(97.5540258162919,0.699185784466034,-1.63292663111069));
#24386=CARTESIAN_POINT('Ctrl Pts',(97.5521386309304,0.672976875088629,-1.64387588136404));
#24387=CARTESIAN_POINT('Ctrl Pts',(97.5512894811523,0.661190549053708,-1.64865182227883));
#24388=CARTESIAN_POINT('Ctrl Pts',(97.5494448649821,0.63560814548388,-1.65869962647025));
#24389=CARTESIAN_POINT('Ctrl Pts',(97.5484479682849,0.621795653474599,-1.66392677356525));
#24390=CARTESIAN_POINT('Ctrl Pts',(97.5456337397525,0.582851037159355,-1.67811220152573));
#24391=CARTESIAN_POINT('Ctrl Pts',(97.5438035982459,0.557580840590902,-1.68667701826366));
#24392=CARTESIAN_POINT('Ctrl Pts',(97.5356947627728,0.445916840385493,-1.72173967235312));
#24393=CARTESIAN_POINT('Ctrl Pts',(97.5292280445423,0.357777737364824,-1.74218831686148));
#24394=CARTESIAN_POINT('Ctrl Pts',(97.5154906050832,0.171087062149514,-1.77073429190682));
#24395=CARTESIAN_POINT('Ctrl Pts',(97.5082226129462,0.0726266187703843,
-1.77749726256714));
#24396=CARTESIAN_POINT('Ctrl Pts',(97.4982865671146,-0.0657028737945895,
-1.77548100536618));
#24397=CARTESIAN_POINT('Ctrl Pts',(97.4954623440966,-0.105491033016684,
-1.77356190921816));
#24398=CARTESIAN_POINT('Ctrl Pts',(97.4918482775702,-0.157405191377807,
-1.76930439050472));
#24399=CARTESIAN_POINT('Ctrl Pts',(97.4910033791617,-0.169615947802007,
-1.76817557724141));
#24400=CARTESIAN_POINT('Ctrl Pts',(97.4896403558562,-0.189451448365353,
-1.76613452273223));
#24401=CARTESIAN_POINT('Ctrl Pts',(97.4891181939661,-0.197083449343026,
-1.76529915973207));
#24402=CARTESIAN_POINT('Ctrl Pts',(97.4880876951923,-0.212216245105763,
-1.76354343023716));
#24403=CARTESIAN_POINT('Ctrl Pts',(97.4875792935411,-0.219717022735083,
-1.76262463370563));
#24404=CARTESIAN_POINT('Ctrl Pts',(97.4862903944107,-0.23881477204022,-1.76016147962614));
#24405=CARTESIAN_POINT('Ctrl Pts',(97.4855135265019,-0.25040300953272,-1.758550335021));
#24406=CARTESIAN_POINT('Ctrl Pts',(97.4822488346855,-0.299382631131891,
-1.75124657307073));
#24407=CARTESIAN_POINT('Ctrl Pts',(97.4798143526546,-0.336605825583204,
-1.74447456493271));
#24408=CARTESIAN_POINT('Ctrl Pts',(97.4727348916702,-0.445812056599596,
-1.72098039604626));
#24409=CARTESIAN_POINT('Ctrl Pts',(97.4681995612666,-0.517002094852825,
-1.70095038621736));
#24410=CARTESIAN_POINT('Ctrl Pts',(97.456465972274,-0.697422097458739,-1.63780859854279));
#24411=CARTESIAN_POINT('Ctrl Pts',(97.4492796176422,-0.803982434135849,
-1.58821377609273));
#24412=CARTESIAN_POINT('Ctrl Pts',(97.4401477387012,-0.925968296669926,
-1.51599725511932));
#24413=CARTESIAN_POINT('Ctrl Pts',(97.4385547338565,-0.946800645888214,
-1.5030746513076));
#24414=CARTESIAN_POINT('Ctrl Pts',(97.4359160716854,-0.980523463569613,
-1.48117663037636));
#24415=CARTESIAN_POINT('Ctrl Pts',(97.4348797076883,-0.993574523347515,
-1.47245377283426));
#24416=CARTESIAN_POINT('Ctrl Pts',(97.4329918750813,-1.01698677046804,-1.45635287971364));
#24417=CARTESIAN_POINT('Ctrl Pts',(97.4321427023145,-1.0273876826591,-1.44903427723535));
#24418=CARTESIAN_POINT('Ctrl Pts',(97.430298582419,-1.04968874435795,-1.43298132699448));
#24419=CARTESIAN_POINT('Ctrl Pts',(97.4293022111883,-1.06156032244852,-1.42420911469984));
#24420=CARTESIAN_POINT('Ctrl Pts',(97.4264910588254,-1.09454981975061,-1.39919070027944));
#24421=CARTESIAN_POINT('Ctrl Pts',(97.4246635131647,-1.11541276598836,-1.38261641498715));
#24422=CARTESIAN_POINT('Ctrl Pts',(97.416577347391,-1.20514525780377,-1.3079766182692));
#24423=CARTESIAN_POINT('Ctrl Pts',(97.4101319519,-1.26990434962579,-1.24519742111886));
#24424=CARTESIAN_POINT('Ctrl Pts',(97.3964564160723,-1.39458129060194,-1.10444835506477));
#24425=CARTESIAN_POINT('Ctrl Pts',(97.3892293069433,-1.45336672559103,-1.02585997100196));
#24426=CARTESIAN_POINT('Ctrl Pts',(97.3792729241883,-1.52690890717147,-0.908437954332116));
#24427=CARTESIAN_POINT('Ctrl Pts',(97.3763936824957,-1.54726285173968,-0.873320421127474));
#24428=CARTESIAN_POINT('Ctrl Pts',(97.3727217778804,-1.57221259036916,-0.826658166702527));
#24429=CARTESIAN_POINT('Ctrl Pts',(97.37187191239,-1.57791438770333,-0.815721987251617));
#24430=CARTESIAN_POINT('Ctrl Pts',(97.3705029029085,-1.58698712218242,-0.797869107188291));
#24431=CARTESIAN_POINT('Ctrl Pts',(97.3699796586266,-1.5904277268772,-0.790988552047881));
#24432=CARTESIAN_POINT('Ctrl Pts',(97.368948933866,-1.59715352074858,-0.777316922696418));
#24433=CARTESIAN_POINT('Ctrl Pts',(97.3684413707099,-1.60044034370457,-0.770526883092213));
#24434=CARTESIAN_POINT('Ctrl Pts',(97.3671574189369,-1.60868708293115,-0.753210023192963));
#24435=CARTESIAN_POINT('Ctrl Pts',(97.3663846039688,-1.61358710124694,-0.742654801724874));
#24436=CARTESIAN_POINT('Ctrl Pts',(97.3631633602325,-1.63372155593118,-0.698142567250437));
#24437=CARTESIAN_POINT('Ctrl Pts',(97.360766519699,-1.64799166739871,-0.663756793432768));
#24438=CARTESIAN_POINT('Ctrl Pts',(97.3538526883113,-1.686595543225,-0.561796150403388));
#24439=CARTESIAN_POINT('Ctrl Pts',(97.3494394367805,-1.70792610792445,-0.49316249557375));
#24440=CARTESIAN_POINT('Ctrl Pts',(97.3376486367997,-1.75370725297439,-0.306647598850043));
#24441=CARTESIAN_POINT('Ctrl Pts',(97.3302904810495,-1.77043637693051,-0.187277883783365));
#24442=CARTESIAN_POINT('Ctrl Pts',(97.3209711507413,-1.77590400877838,-0.0427287498799004));
#24443=CARTESIAN_POINT('Ctrl Pts',(97.3193835348976,-1.77632365132989,-0.0183026660531491));
#24444=CARTESIAN_POINT('Ctrl Pts',(97.3167519319475,-1.77618541557409,0.0217959979527274));
#24445=CARTESIAN_POINT('Ctrl Pts',(97.3157171507233,-1.77592395982576,0.03746676737239));
#24446=CARTESIAN_POINT('Ctrl Pts',(97.3138309782691,-1.77507480664552,0.0658422154165484));
#24447=CARTESIAN_POINT('Ctrl Pts',(97.3129818632966,-1.77455795980832,0.0785480701765516));
#24448=CARTESIAN_POINT('Ctrl Pts',(97.3111364635747,-1.77314548069506,0.106007639902053));
#24449=CARTESIAN_POINT('Ctrl Pts',(97.310138738753,-1.77220203153463,0.120757822955018));
#24450=CARTESIAN_POINT('Ctrl Pts',(97.3073196593275,-1.76903501638525,0.162154598168923));
#24451=CARTESIAN_POINT('Ctrl Pts',(97.3054854237162,-1.76639376137816,0.188764263306146));
#24452=CARTESIAN_POINT('Ctrl Pts',(97.2973407224382,-1.75214545687766,0.305446082672367));
#24453=CARTESIAN_POINT('Ctrl Pts',(97.2908402468761,-1.73424281787076,0.394599184517063));
#24454=CARTESIAN_POINT('Ctrl Pts',(97.2770047110806,-1.68263807558025,0.577643171424734));
#24455=CARTESIAN_POINT('Ctrl Pts',(97.2696719100604,-1.64768724992194,0.670872396629719));
#24456=CARTESIAN_POINT('Ctrl Pts',(97.2597675593518,-1.58857683900526,0.795600517175361));
#24457=CARTESIAN_POINT('Ctrl Pts',(97.2570298003482,-1.57089613344093,0.829965294096662));
#24458=CARTESIAN_POINT('Ctrl Pts',(97.2535070094585,-1.54620057919384,0.874342827559403));
#24459=CARTESIAN_POINT('Ctrl Pts',(97.2526702215721,-1.54018500197428,0.884896486325083));
#24460=CARTESIAN_POINT('Ctrl Pts',(97.2513169723814,-1.53020391956021,0.901996999300388));
#24461=CARTESIAN_POINT('Ctrl Pts',(97.2507965767226,-1.52630365180364,0.90858119632006));
#24462=CARTESIAN_POINT('Ctrl Pts',(97.2497663855819,-1.51845612724343,0.921635769876499));
#24463=CARTESIAN_POINT('Ctrl Pts',(97.2492565549594,-1.5145097787729,0.928106479612119));
#24464=CARTESIAN_POINT('Ctrl Pts',(97.2479592888655,-1.50431117307256,0.944590550038746));
#24465=CARTESIAN_POINT('Ctrl Pts',(97.2471755779381,-1.49800016638621,0.954567406163399));
#24466=CARTESIAN_POINT('Ctrl Pts',(97.2438358350591,-1.47048517816666,0.9971199113172));
#24467=CARTESIAN_POINT('Ctrl Pts',(97.2413362485873,-1.44831297389702,1.0290601595754));
#24468=CARTESIAN_POINT('Ctrl Pts',(97.2339619328085,-1.37878588131345,1.12251330870453));
#24469=CARTESIAN_POINT('Ctrl Pts',(97.2292077771675,-1.32842920507166,1.18167850176388));
#24470=CARTESIAN_POINT('Ctrl Pts',(97.2175659236551,-1.19630020488104,1.31775821212839));
#24471=CARTESIAN_POINT('Ctrl Pts',(97.2106811198566,-1.11081606362786,1.39057718012086));
#24472=CARTESIAN_POINT('Ctrl Pts',(97.2018789256366,-0.998881716832708,
1.46898113449752));
#24473=CARTESIAN_POINT('Ctrl Pts',(97.2002791064077,-0.978424934848719,
1.48268500023095));
#24474=CARTESIAN_POINT('Ctrl Pts',(97.1976315196005,-0.944443945374345,
1.50443912808453));
#24475=CARTESIAN_POINT('Ctrl Pts',(97.1965931564276,-0.931085496684032,
1.51274294821485));
#24476=CARTESIAN_POINT('Ctrl Pts',(97.1947032211352,-0.906728151337016,
1.52743900287166));
#24477=CARTESIAN_POINT('Ctrl Pts',(97.1938539695854,-0.895767402797125,
1.53389262777006));
#24478=CARTESIAN_POINT('Ctrl Pts',(97.1920114379733,-0.871960020407261,
1.5475680775706));
#24479=CARTESIAN_POINT('Ctrl Pts',(97.1910167537556,-0.859091006703501,
1.55474880648389));
#24480=CARTESIAN_POINT('Ctrl Pts',(97.1882154683958,-0.822812517113445,
1.57440375694013));
#24481=CARTESIAN_POINT('Ctrl Pts',(97.1863962470377,-0.799211634499652,
1.58651450011723));
#24482=CARTESIAN_POINT('Ctrl Pts',(97.1783824117319,-0.695124533531911,
1.6370146566962));
#24483=CARTESIAN_POINT('Ctrl Pts',(97.1720049753289,-0.612094162819844,
1.66983583021668));
#24484=CARTESIAN_POINT('Ctrl Pts',(97.1585270858967,-0.43506842514852,1.72483011750404));
#24485=CARTESIAN_POINT('Ctrl Pts',(97.1514306723062,-0.341007551365627,
1.74586297560811));
#24486=CARTESIAN_POINT('Ctrl Pts',(97.1414082978119,-0.203113291364408,
1.7651228170062));
#24487=CARTESIAN_POINT('Ctrl Pts',(97.1383514679536,-0.160314922159936,
1.76952348048217));
#24488=CARTESIAN_POINT('Ctrl Pts',(97.1344939003206,-0.104873976243193,
1.77319569920614));
#24489=CARTESIAN_POINT('Ctrl Pts',(97.1336287794512,-0.0923435747748574,
1.77389239396708));
#24490=CARTESIAN_POINT('Ctrl Pts',(97.1322413848747,-0.0720747270036096,
1.77480398802844));
#24491=CARTESIAN_POINT('Ctrl Pts',(97.1317148143736,-0.0643406747606824,
1.77510119305181));
#24492=CARTESIAN_POINT('Ctrl Pts',(97.1306832296948,-0.0491027974133395,
1.77558703367662));
#24493=CARTESIAN_POINT('Ctrl Pts',(97.1301780788872,-0.0415993020025549,
1.77577867441447));
#24494=CARTESIAN_POINT('Ctrl Pts',(97.1289085389308,-0.0226430246713958,
1.77614260265007));
#24495=CARTESIAN_POINT('Ctrl Pts',(97.1281475614745,-0.0111891226172256,
1.77625169170191));
#24496=CARTESIAN_POINT('Ctrl Pts',(97.1250492133195,0.0357787533883522,
1.7762446737839));
#24497=CARTESIAN_POINT('Ctrl Pts',(97.1227586406784,0.0712867991049795,
1.7751743152286));
#24498=CARTESIAN_POINT('Ctrl Pts',(97.1162950305329,0.172845117764904,1.76906024427386));
#24499=CARTESIAN_POINT('Ctrl Pts',(97.1122105058241,0.238679117805502,1.76138668741203));
#24500=CARTESIAN_POINT('Ctrl Pts',(97.1002246383258,0.430868106740661,1.72800891534555));
#24501=CARTESIAN_POINT('Ctrl Pts',(97.0923726650692,0.55501253424185,1.69222314860588));
#24502=CARTESIAN_POINT('Ctrl Pts',(97.0823745223659,0.698493225962655,1.63335890088485));
#24503=CARTESIAN_POINT('Ctrl Pts',(97.0806650065087,0.722570553588963,1.62285112223711));
#24504=CARTESIAN_POINT('Ctrl Pts',(97.0779617095857,0.759868485290847,1.60557904907658));
#24505=CARTESIAN_POINT('Ctrl Pts',(97.0769802924953,0.773252909511442,1.59917607325386));
#24506=CARTESIAN_POINT('Ctrl Pts',(97.0751471079851,0.797953545575903,1.58697694172729));
#24507=CARTESIAN_POINT('Ctrl Pts',(97.0742969456289,0.809290845786817,1.58122546997481));
#24508=CARTESIAN_POINT('Ctrl Pts',(97.0723937785026,0.834402295125258,1.56814549233746));
#24509=CARTESIAN_POINT('Ctrl Pts',(97.0713386752196,0.848143445752201,1.56075627294693));
#24510=CARTESIAN_POINT('Ctrl Pts',(97.0681735957177,0.888816656263697,1.53818876349456));
#24511=CARTESIAN_POINT('Ctrl Pts',(97.0660451740991,0.915450476266847,1.52248807480269));
#24512=CARTESIAN_POINT('Ctrl Pts',(97.0610386058693,0.976415652249444,1.48437081837268));
#24513=CARTESIAN_POINT('Ctrl Pts',(97.0581436265264,1.01040655970784,1.46144531268299));
#24514=CARTESIAN_POINT('Ctrl Pts',(97.049258427071,1.11102903602351,1.38839029939366));
#24515=CARTESIAN_POINT('Ctrl Pts',(97.0431680248593,1.17494992942416,1.33472986932186));
#24516=CARTESIAN_POINT('Ctrl Pts',(97.0307192152893,1.29730785162441,1.21638951963325));
#24517=CARTESIAN_POINT('Ctrl Pts',(97.0243771319298,1.35524452362216,1.15148867475972));
#24518=CARTESIAN_POINT('Ctrl Pts',(97.0169997496471,1.4193385354125,1.0681179724614));
#24519=CARTESIAN_POINT('Ctrl Pts',(97.0157295545419,1.43025070804374,1.05346137012385));
#24520=CARTESIAN_POINT('Ctrl Pts',(97.0138599260109,1.44615416754452,1.03139800501371));
#24521=CARTESIAN_POINT('Ctrl Pts',(97.0132497800798,1.45131853483857,1.02411827448091));
#24522=CARTESIAN_POINT('Ctrl Pts',(97.012155890293,1.46053464249223,1.01091744804623));
#24523=CARTESIAN_POINT('Ctrl Pts',(97.0116709082636,1.46460559487596,1.00501044000254));
#24524=CARTESIAN_POINT('Ctrl Pts',(97.0105756303623,1.47376438546499,0.991547060228764));
#24525=CARTESIAN_POINT('Ctrl Pts',(97.0099667970941,1.47883001295977,0.983976035451259));
#24526=CARTESIAN_POINT('Ctrl Pts',(97.0080828446287,1.49441571386986,0.960289589506029));
#24527=CARTESIAN_POINT('Ctrl Pts',(97.0068202079099,1.5047326768303,0.944041347951515));
#24528=CARTESIAN_POINT('Ctrl Pts',(97.0038335954327,1.52875814735824,0.904808589507813));
#24529=CARTESIAN_POINT('Ctrl Pts',(97.0021222800539,1.54221559549797,0.88167526036637));
#24530=CARTESIAN_POINT('Ctrl Pts',(96.9953707256256,1.59377530975649,0.78824875730905));
#24531=CARTESIAN_POINT('Ctrl Pts',(96.9904792453346,1.62763744376648,0.715719130817615));
#24532=CARTESIAN_POINT('Ctrl Pts',(96.978889146187,1.69579252162487,0.539631291163661));
#24533=CARTESIAN_POINT('Ctrl Pts',(96.9721904887946,1.72566616018116,0.434726319353921));
#24534=CARTESIAN_POINT('Ctrl Pts',(96.9635918250881,1.75030149880858,0.303508253355444));
#24535=CARTESIAN_POINT('Ctrl Pts',(96.9619890049453,1.75434757062463,0.279172174149227));
#24536=CARTESIAN_POINT('Ctrl Pts',(96.9593374885332,1.76014328628504,0.23918089587824));
#24537=CARTESIAN_POINT('Ctrl Pts',(96.9582982457689,1.76219389142332,0.223572251439364));
#24538=CARTESIAN_POINT('Ctrl Pts',(96.9564073833407,1.76552582789372,0.19530596532271));
#24539=CARTESIAN_POINT('Ctrl Pts',(96.9555580951217,1.76687916796851,0.182657768429895));
#24540=CARTESIAN_POINT('Ctrl Pts',(96.9537162525086,1.76950588575419,0.155337834371209));
#24541=CARTESIAN_POINT('Ctrl Pts',(96.9527223026571,1.77073287188001,0.140662703501392));
#24542=CARTESIAN_POINT('Ctrl Pts',(96.9499253081035,1.77365474898305,0.0995677215331412));
#24543=CARTESIAN_POINT('Ctrl Pts',(96.9481097057095,1.77494160268787,0.0731236978369465));
#24544=CARTESIAN_POINT('Ctrl Pts',(96.944100004836,1.77646235425336,0.0152542663560143));
#24545=CARTESIAN_POINT('Ctrl Pts',(96.941899944293,1.77645395205389,-0.0161581873154769));
#24546=CARTESIAN_POINT('Ctrl Pts',(96.9396785576437,1.77561363837197,-0.0475422940912364));
#24547=CARTESIAN_POINT('Ctrl Pts',(96.7921246220486,1.77561363846711,-0.047542290537889));
#24548=CARTESIAN_POINT('Ctrl Pts',(96.7964447788134,1.77739515555032,0.0189939657997468));
#24549=CARTESIAN_POINT('Ctrl Pts',(96.8006048204907,1.77543573913087,0.0855923702015854));
#24550=CARTESIAN_POINT('Ctrl Pts',(96.812453165962,1.75903281059313,0.276651251963474));
#24551=CARTESIAN_POINT('Ctrl Pts',(96.8200135814896,1.73517407008014,0.399877807502835));
#24552=CARTESIAN_POINT('Ctrl Pts',(96.8306304720267,1.68616500917452,0.560095940657845));
#24553=CARTESIAN_POINT('Ctrl Pts',(96.8333516475131,1.67232381214624,0.600160416610597));
#24554=CARTESIAN_POINT('Ctrl Pts',(96.8372865232963,1.65062767335898,0.656362528423919));
#24555=CARTESIAN_POINT('Ctrl Pts',(96.8384618042765,1.64394012962833,0.67293706732107));
#24556=CARTESIAN_POINT('Ctrl Pts',(96.8404906809162,1.6320511108791,0.701167645391426));
#24557=CARTESIAN_POINT('Ctrl Pts',(96.8413400898277,1.62697192878429,0.712873918648169));
#24558=CARTESIAN_POINT('Ctrl Pts',(96.8430925787236,1.61628800597513,0.736788696637372));
#24559=CARTESIAN_POINT('Ctrl Pts',(96.8439960697155,1.61067002940363,0.748990347658202));
#24560=CARTESIAN_POINT('Ctrl Pts',(96.8463034153427,1.59604883355745,0.779820645789451));
#24561=CARTESIAN_POINT('Ctrl Pts',(96.8477137014826,1.58685773829916,0.798357422382559));
#24562=CARTESIAN_POINT('Ctrl Pts',(96.8540677960926,1.54433598719296,0.880479525270836));
#24563=CARTESIAN_POINT('Ctrl Pts',(96.8591329785776,1.50749654764157,0.942162202374973));
#24564=CARTESIAN_POINT('Ctrl Pts',(96.8695931636956,1.42548878223303,1.06229706485265));
#24565=CARTESIAN_POINT('Ctrl Pts',(96.8749834812004,1.38020197212018,1.12050645596623));
#24566=CARTESIAN_POINT('Ctrl Pts',(96.8865198422848,1.27577202841406,1.2387660736924));
#24567=CARTESIAN_POINT('Ctrl Pts',(96.8926515950852,1.21569810877325,1.29777362695381));
#24568=CARTESIAN_POINT('Ctrl Pts',(96.8998280586781,1.13780835196938,1.36410682875712));
#24569=CARTESIAN_POINT('Ctrl Pts',(96.9010931926984,1.12377132544589,1.3756937735119));
#24570=CARTESIAN_POINT('Ctrl Pts',(96.9029532923447,1.1026399741394,1.3925974415513));
#24571=CARTESIAN_POINT('Ctrl Pts',(96.9035589159462,1.09568043352037,1.39807973407652));
#24572=CARTESIAN_POINT('Ctrl Pts',(96.9046433439711,1.08306969366155,1.40786168167976));
#24573=CARTESIAN_POINT('Ctrl Pts',(96.9051233836791,1.07743345136915,1.4121797471655));
#24574=CARTESIAN_POINT('Ctrl Pts',(96.9062050355867,1.06461167078221,1.421881379454));
#24575=CARTESIAN_POINT('Ctrl Pts',(96.9068052458399,1.05741104328753,1.42724439428766));
#24576=CARTESIAN_POINT('Ctrl Pts',(96.9086533129944,1.03498551854855,1.44368400586207));
#24577=CARTESIAN_POINT('Ctrl Pts',(96.909889252023,1.01962440202222,1.45457371095675));
#24578=CARTESIAN_POINT('Ctrl Pts',(96.9128043924381,0.982610088426438,1.47993908084542));
#24579=CARTESIAN_POINT('Ctrl Pts',(96.9144716581201,0.960805583072234,1.49418708381056));
#24580=CARTESIAN_POINT('Ctrl Pts',(96.920953376074,0.873932328040859,1.54826539454819));
#24581=CARTESIAN_POINT('Ctrl Pts',(96.925630371973,0.806635854375908,1.58436851892709));
#24582=CARTESIAN_POINT('Ctrl Pts',(96.9373240046006,0.633304977635761,1.66344073482572));
#24583=CARTESIAN_POINT('Ctrl Pts',(96.9443349296379,0.525069159632757,1.70070835108507));
#24584=CARTESIAN_POINT('Ctrl Pts',(96.9532696817117,0.390193324115174,1.73303580662048));
#24585=CARTESIAN_POINT('Ctrl Pts',(96.9548613558169,0.366261030807749,1.73825104666723));
#24586=CARTESIAN_POINT('Ctrl Pts',(96.9574928765716,0.326912764294527,1.74597701949301));
#24587=CARTESIAN_POINT('Ctrl Pts',(96.95852338655,0.311557519845261,1.74878231747823));
#24588=CARTESIAN_POINT('Ctrl Pts',(96.9603970325971,0.283749893352351,1.75348472249315));
#24589=CARTESIAN_POINT('Ctrl Pts',(96.9612378650935,0.27131039042699,1.75545245791126));
#24590=CARTESIAN_POINT('Ctrl Pts',(96.9630596054171,0.244451534714864,1.75940881024588));
#24591=CARTESIAN_POINT('Ctrl Pts',(96.9640418626066,0.230026644514653,1.76135278556069));
#24592=CARTESIAN_POINT('Ctrl Pts',(96.966799889143,0.189693454588111,1.76628439955327));
#24593=CARTESIAN_POINT('Ctrl Pts',(96.9685878122483,0.163741755030993,1.76887893836206));
#24594=CARTESIAN_POINT('Ctrl Pts',(96.9763883743647,0.0514064580066014,
1.77761655614586));
#24595=CARTESIAN_POINT('Ctrl Pts',(96.982573116723,-0.035293795279772,1.77800836838871));
#24596=CARTESIAN_POINT('Ctrl Pts',(96.9985934246228,-0.255340920855718,
1.76290052340124));
#24597=CARTESIAN_POINT('Ctrl Pts',(97.0085448120822,-0.387550199956913,
1.73862725078292));
#24598=CARTESIAN_POINT('Ctrl Pts',(97.0191600894515,-0.532520608749415,
1.69463626370219));
#24599=CARTESIAN_POINT('Ctrl Pts',(97.0203754351104,-0.549190095965706,
1.68930771652308));
#24600=CARTESIAN_POINT('Ctrl Pts',(97.0221771293506,-0.57404809235193,1.68095477367118));
#24601=CARTESIAN_POINT('Ctrl Pts',(97.0227732239686,-0.582296947066406,
1.67811514413915));
#24602=CARTESIAN_POINT('Ctrl Pts',(97.0237999986401,-0.596553967283767,
1.67308944619742));
#24603=CARTESIAN_POINT('Ctrl Pts',(97.0242322674264,-0.602571579418622,
1.67093160418261));
#24604=CARTESIAN_POINT('Ctrl Pts',(97.0252514473587,-0.616795775604597,
1.66574414372838));
#24605=CARTESIAN_POINT('Ctrl Pts',(97.0258366921472,-0.624991787644568,
1.66268633681345));
#24606=CARTESIAN_POINT('Ctrl Pts',(97.0275908110972,-0.649628707404103,
1.65328675975727));
#24607=CARTESIAN_POINT('Ctrl Pts',(97.0287494446904,-0.665998711690172,
1.64676055976514));
#24608=CARTESIAN_POINT('Ctrl Pts',(97.0345202515308,-0.747839619869079,
1.6127130873036));
#24609=CARTESIAN_POINT('Ctrl Pts',(97.0389555749711,-0.811722108132453,
1.58152363764978));
#24610=CARTESIAN_POINT('Ctrl Pts',(97.0513395237855,-0.986347753285769,
1.48288855856811));
#24611=CARTESIAN_POINT('Ctrl Pts',(97.0591630340525,-1.09181179150756,1.40704864269163));
#24612=CARTESIAN_POINT('Ctrl Pts',(97.0698164253239,-1.21629494828761,1.29504056451034));
#24613=CARTESIAN_POINT('Ctrl Pts',(97.072260109002,-1.24367609972905,1.26876826021332));
#24614=CARTESIAN_POINT('Ctrl Pts',(97.0757548194568,-1.28103053732408,1.23055481926915));
#24615=CARTESIAN_POINT('Ctrl Pts',(97.0767746761328,-1.29172150084308,1.21932765897184));
#24616=CARTESIAN_POINT('Ctrl Pts',(97.0786516633516,-1.31100480635862,1.19853897021191));
#24617=CARTESIAN_POINT('Ctrl Pts',(97.0795067625237,-1.31964300433458,1.18902127470431));
#24618=CARTESIAN_POINT('Ctrl Pts',(97.0812549079677,-1.33700048530506,1.16947439184729));
#24619=CARTESIAN_POINT('Ctrl Pts',(97.0821482008997,-1.3457120103945,1.15943944183592));
#24620=CARTESIAN_POINT('Ctrl Pts',(97.0843965969524,-1.3672393828856,1.13407223300584));
#24621=CARTESIAN_POINT('Ctrl Pts',(97.0857574831402,-1.37991034479923,1.11862001730415));
#24622=CARTESIAN_POINT('Ctrl Pts',(97.0914914487322,-1.43178841421404,1.05313180080035));
#24623=CARTESIAN_POINT('Ctrl Pts',(97.0959579958422,-1.4685516512384,1.00122875218225));
#24624=CARTESIAN_POINT('Ctrl Pts',(97.1104778902586,-1.57677748651851,0.829610029613119));
#24625=CARTESIAN_POINT('Ctrl Pts',(97.1208335988343,-1.63696940836888,0.70342456580508));
#24626=CARTESIAN_POINT('Ctrl Pts',(97.1336208900391,-1.69429936580948,0.534718315285902));
#24627=CARTESIAN_POINT('Ctrl Pts',(97.13637485676,-1.70559240627777,0.497522928713749));
#24628=CARTESIAN_POINT('Ctrl Pts',(97.1399096889589,-1.71878972359002,0.448299338157641));
#24629=CARTESIAN_POINT('Ctrl Pts',(97.1407430485851,-1.72180317668285,0.43658246831632));
#24630=CARTESIAN_POINT('Ctrl Pts',(97.142088816883,-1.72651266650006,0.417463432082526));
#24631=CARTESIAN_POINT('Ctrl Pts',(97.1426051472756,-1.72828130547131,0.410079796341151));
#24632=CARTESIAN_POINT('Ctrl Pts',(97.1436248591873,-1.73169894858246,0.395397021229398));
#24633=CARTESIAN_POINT('Ctrl Pts',(97.1441282981559,-1.73334927295381,0.388098383428364));
#24634=CARTESIAN_POINT('Ctrl Pts',(97.1454048150938,-1.73743737471039,0.369472165279576));
#24635=CARTESIAN_POINT('Ctrl Pts',(97.1461743304743,-1.7398105796098,0.358130530412814));
#24636=CARTESIAN_POINT('Ctrl Pts',(97.1494052162996,-1.74937621171833,0.310075008072325));
#24637=CARTESIAN_POINT('Ctrl Pts',(97.1518143351096,-1.75551932797031,0.273159269936031));
#24638=CARTESIAN_POINT('Ctrl Pts',(97.1587955145102,-1.77015237298934,0.164035246997141));
#24639=CARTESIAN_POINT('Ctrl Pts',(97.1632609839627,-1.77538230794254,0.0914662706970687));
#24640=CARTESIAN_POINT('Ctrl Pts',(97.1750475747397,-1.77741189813986,-0.100518833926835));
#24641=CARTESIAN_POINT('Ctrl Pts',(97.1823522785257,-1.76665170757841,-0.219624527224935));
#24642=CARTESIAN_POINT('Ctrl Pts',(97.1916080995304,-1.73941698698552,-0.360675059840408));
#24643=CARTESIAN_POINT('Ctrl Pts',(97.1931920252482,-1.73430511803478,-0.384504380974449));
#24644=CARTESIAN_POINT('Ctrl Pts',(97.1958133984703,-1.72512569111611,-0.423376840570269));
#24645=CARTESIAN_POINT('Ctrl Pts',(97.1968416349678,-1.72134746753916,-0.438485426767537));
#24646=CARTESIAN_POINT('Ctrl Pts',(97.1987128806093,-1.71415599149307,-0.46571649676011));
#24647=CARTESIAN_POINT('Ctrl Pts',(97.1995536139837,-1.71081152139738,-0.47785619461491));
#24648=CARTESIAN_POINT('Ctrl Pts',(97.2013771146071,-1.70331603933357,-0.503975365254594));
#24649=CARTESIAN_POINT('Ctrl Pts',(97.2023612533175,-1.69912140310034,-0.517941245732923));
#24650=CARTESIAN_POINT('Ctrl Pts',(97.2051302485903,-1.68690724117204,-0.556861766518304));
#24651=CARTESIAN_POINT('Ctrl Pts',(97.2069274165484,-1.67850689142334,-0.581691976034354));
#24652=CARTESIAN_POINT('Ctrl Pts',(97.2148067121049,-1.63966350286731,-0.688649913801664));
#24653=CARTESIAN_POINT('Ctrl Pts',(97.2210651056521,-1.60372282088699,-0.76863793066768));
#24654=CARTESIAN_POINT('Ctrl Pts',(97.2370371008279,-1.49907257137219,-0.961944159257952));
#24655=CARTESIAN_POINT('Ctrl Pts',(97.2468546196268,-1.42331572932107,-1.07085487533517));
#24656=CARTESIAN_POINT('Ctrl Pts',(97.257376592498,-1.32442397590784,-1.18375796618308));
#24657=CARTESIAN_POINT('Ctrl Pts',(97.2586151093142,-1.31247760969416,-1.19698971390143));
#24658=CARTESIAN_POINT('Ctrl Pts',(97.2604440171926,-1.29434748833199,-1.21647271009461));
#24659=CARTESIAN_POINT('Ctrl Pts',(97.2610445743363,-1.28831363990794,-1.22286109122872));
#24660=CARTESIAN_POINT('Ctrl Pts',(97.2621240053079,-1.27731783872516,-1.23433125113996));
#24661=CARTESIAN_POINT('Ctrl Pts',(97.2626040534628,-1.27237259472514,-1.23942828873989));
#24662=CARTESIAN_POINT('Ctrl Pts',(97.2636908072777,-1.26105210343334,-1.25095709592858));
#24663=CARTESIAN_POINT('Ctrl Pts',(97.2642960468508,-1.25465809460004,-1.25736992885211));
#24664=CARTESIAN_POINT('Ctrl Pts',(97.2661763810441,-1.23452415238336,-1.2772566269728));
#24665=CARTESIAN_POINT('Ctrl Pts',(97.2674389524133,-1.2206136181369,-1.29055679571444));
#24666=CARTESIAN_POINT('Ctrl Pts',(97.2704296508956,-1.18680397253319,-1.32184711531286));
#24667=CARTESIAN_POINT('Ctrl Pts',(97.2721449911464,-1.16670776540666,-1.33961808275311));
#24668=CARTESIAN_POINT('Ctrl Pts',(97.2789432514273,-1.08462189308028,-1.40895714980607));
#24669=CARTESIAN_POINT('Ctrl Pts',(97.283874780039,-1.01955282429897,-1.45673561465998));
#24670=CARTESIAN_POINT('Ctrl Pts',(97.2954711895805,-0.860026200855641,
-1.55792901095098));
#24671=CARTESIAN_POINT('Ctrl Pts',(97.3021365298245,-0.763492444096923,
-1.6074400867708));
#24672=CARTESIAN_POINT('Ctrl Pts',(97.3106933950468,-0.640248316684155,
-1.65703067764064));
#24673=CARTESIAN_POINT('Ctrl Pts',(97.3122910454977,-0.617251624051435,
-1.66573374581545));
#24674=CARTESIAN_POINT('Ctrl Pts',(97.3149303912862,-0.579346533057907,
-1.67918615956426));
#24675=CARTESIAN_POINT('Ctrl Pts',(97.3159626525256,-0.564542491003731,
-1.68422098122485));
#24676=CARTESIAN_POINT('Ctrl Pts',(97.3178381530711,-0.537696704700965,
-1.69295746327319));
#24677=CARTESIAN_POINT('Ctrl Pts',(97.3186790673972,-0.525678266957292,
-1.69672775196515));
#24678=CARTESIAN_POINT('Ctrl Pts',(97.3204994785212,-0.49970721178704,-1.70457268039935));
#24679=CARTESIAN_POINT('Ctrl Pts',(97.3214803078673,-0.485742726433725,
-1.70860448965804));
#24680=CARTESIAN_POINT('Ctrl Pts',(97.3242300216845,-0.446684123924979,
-1.71936392022173));
#24681=CARTESIAN_POINT('Ctrl Pts',(97.3260109410571,-0.421490431045736,
-1.72571280599883));
#24682=CARTESIAN_POINT('Ctrl Pts',(97.3337522880547,-0.312474011707557,
-1.75065569791172));
#24683=CARTESIAN_POINT('Ctrl Pts',(97.3398817255156,-0.22751398002855,-1.76370888235658));
#24684=CARTESIAN_POINT('Ctrl Pts',(97.3559399967528,-0.00706829237110624,
-1.78138294563386));
#24685=CARTESIAN_POINT('Ctrl Pts',(97.3659939781483,0.128613232912918,-1.77674882383763));
#24686=CARTESIAN_POINT('Ctrl Pts',(97.3766799138629,0.279507850834532,-1.75420542811582));
#24687=CARTESIAN_POINT('Ctrl Pts',(97.3778769871444,0.296522648170575,-1.75140963144019));
#24688=CARTESIAN_POINT('Ctrl Pts',(97.3796571816436,0.322031709003508,-1.74683567134944));
#24689=CARTESIAN_POINT('Ctrl Pts',(97.3802497230266,0.33055751129651,-1.74524239691463));
#24690=CARTESIAN_POINT('Ctrl Pts',(97.3812730700376,0.345348963089256,-1.74236593535558));
#24691=CARTESIAN_POINT('Ctrl Pts',(97.3817054220512,0.35161967246017,-1.7411113026109));
#24692=CARTESIAN_POINT('Ctrl Pts',(97.3827281659052,0.366503789168647,-1.73804962048148));
#24693=CARTESIAN_POINT('Ctrl Pts',(97.3833168496211,0.375110709306221,-1.73621239331826));
#24694=CARTESIAN_POINT('Ctrl Pts',(97.3850922947925,0.401175619673715,-1.73044571994207));
#24695=CARTESIAN_POINT('Ctrl Pts',(97.3862684459935,0.418588808355007,-1.72631623326657));
#24696=CARTESIAN_POINT('Ctrl Pts',(97.3922185767068,0.507231746150265,-1.70387460894952));
#24697=CARTESIAN_POINT('Ctrl Pts',(97.3968032529147,0.577344520500685,-1.68141262582316));
#24698=CARTESIAN_POINT('Ctrl Pts',(97.4098068981207,0.773718353630419,-1.60476158921119));
#24699=CARTESIAN_POINT('Ctrl Pts',(97.4180998167281,0.895342774546599,-1.54021384451901));
#24700=CARTESIAN_POINT('Ctrl Pts',(97.4289225824041,1.0343752584647,-1.44434531561639));
#24701=CARTESIAN_POINT('Ctrl Pts',(97.4309729684634,1.05994234757812,-1.42568846128217));
#24702=CARTESIAN_POINT('Ctrl Pts',(97.4340760512741,1.09738413411021,-1.39680239221828));
#24703=CARTESIAN_POINT('Ctrl Pts',(97.435108919311,1.10964483692882,-1.38708225078516));
#24704=CARTESIAN_POINT('Ctrl Pts',(97.4369850635182,1.1315418230313,-1.36924644871359));
#24705=CARTESIAN_POINT('Ctrl Pts',(97.4378260072926,1.14122330737616,-1.36118774723576));
#24706=CARTESIAN_POINT('Ctrl Pts',(97.4396459632077,1.1618842645315,-1.34361455493872));
#24707=CARTESIAN_POINT('Ctrl Pts',(97.4406263021129,1.17283429100162,-1.33406702244634));
#24708=CARTESIAN_POINT('Ctrl Pts',(97.4433731628355,1.20301071179697,-1.30709695413706));
#24709=CARTESIAN_POINT('Ctrl Pts',(97.4451516788816,1.22197364284283,-1.28938648683015));
#24710=CARTESIAN_POINT('Ctrl Pts',(97.4528727909988,1.30180750181456,-1.21148222811849));
#24711=CARTESIAN_POINT('Ctrl Pts',(97.4589833470828,1.35866333791957,-1.14735442500851));
#24712=CARTESIAN_POINT('Ctrl Pts',(97.4750549189262,1.49317811195947,-0.971554783332337));
#24713=CARTESIAN_POINT('Ctrl Pts',(97.4851443442598,1.56305236894657,-0.854616541608144));
#24714=CARTESIAN_POINT('Ctrl Pts',(97.4958545248844,1.62598022212548,-0.715224813145737));
#24715=CARTESIAN_POINT('Ctrl Pts',(97.4970451875861,1.63281069967429,-0.699490878835642));
#24716=CARTESIAN_POINT('Ctrl Pts',(97.4988178309789,1.64274381488037,-0.675671320992764));
#24717=CARTESIAN_POINT('Ctrl Pts',(97.4994091186317,1.64601677287129,-0.667658420661842));
#24718=CARTESIAN_POINT('Ctrl Pts',(97.5004312664794,1.65160629733246,-0.653683110942573));
#24719=CARTESIAN_POINT('Ctrl Pts',(97.5008636580802,1.65394935300564,-0.647731820814894));
#24720=CARTESIAN_POINT('Ctrl Pts',(97.5018877044466,1.65944693011367,-0.633543791320473));
#24721=CARTESIAN_POINT('Ctrl Pts',(97.5024776359595,1.66257231444965,-0.625296055382906));
#24722=CARTESIAN_POINT('Ctrl Pts',(97.5042608568555,1.67188687115351,-0.600151759963838));
#24723=CARTESIAN_POINT('Ctrl Pts',(97.5054433995845,1.67788106119412,-0.583183547937348));
#24724=CARTESIAN_POINT('Ctrl Pts',(97.5114601514787,1.70735618660297,-0.495526776001437));
#24725=CARTESIAN_POINT('Ctrl Pts',(97.5161003219243,1.72663425252144,-0.42349563145663));
#24726=CARTESIAN_POINT('Ctrl Pts',(97.5269767928662,1.76143472299729,-0.250582050110423));
#24727=CARTESIAN_POINT('Ctrl Pts',(97.5331561149429,1.77289076556361,-0.149236379042087));
#24728=CARTESIAN_POINT('Ctrl Pts',(97.5395352881717,1.77561363837197,-0.0475422940912269));
#24729=CARTESIAN_POINT('Origin',(88.3562164250559,0.,0.));
#24730=CARTESIAN_POINT('',(98.4367443001643,1.7756136383719,-0.0475422940939716));
#24731=CARTESIAN_POINT('',(98.289313862947,1.77561363837197,-0.0475422940912461));
#24732=CARTESIAN_POINT('',(88.3562164250559,1.77561363837197,-0.0475422940912398));
#24733=CARTESIAN_POINT('Ctrl Pts',(98.4367443001643,1.77561363837182,-0.0475422940967033));
#24734=CARTESIAN_POINT('Ctrl Pts',(98.4365226374283,1.77552297576021,-0.0509283690169651));
#24735=CARTESIAN_POINT('Ctrl Pts',(98.4363014139303,1.77542262597964,-0.0543142353769213));
#24736=CARTESIAN_POINT('Ctrl Pts',(98.4286423307297,1.7716056866418,-0.171754060191483));
#24737=CARTESIAN_POINT('Ctrl Pts',(98.4216940556708,1.75691583374141,-0.28520175953313));
#24738=CARTESIAN_POINT('Ctrl Pts',(98.4079341841336,1.70689092790807,-0.503668546124907));
#24739=CARTESIAN_POINT('Ctrl Pts',(98.401151729996,1.67244459277732,-0.608345121057067));
#24740=CARTESIAN_POINT('Ctrl Pts',(98.3924543515143,1.61872191312569,-0.731716303873464));
#24741=CARTESIAN_POINT('Ctrl Pts',(98.3908498136962,1.60843200433929,-0.754066159180973));
#24742=CARTESIAN_POINT('Ctrl Pts',(98.3882849468019,1.59141509328202,-0.789092966644753));
#24743=CARTESIAN_POINT('Ctrl Pts',(98.3873351652438,1.58499274876237,-0.801915004951576));
#24744=CARTESIAN_POINT('Ctrl Pts',(98.3855293391019,1.57255970802052,-0.826004280537739));
#24745=CARTESIAN_POINT('Ctrl Pts',(98.3846744785475,1.5665813571433,-0.837287252671703));
#24746=CARTESIAN_POINT('Ctrl Pts',(98.3827171014043,1.55268629428937,-0.862841618770187));
#24747=CARTESIAN_POINT('Ctrl Pts',(98.3816119228124,1.54469359885245,-0.877070146655087));
#24748=CARTESIAN_POINT('Ctrl Pts',(98.3786807758117,1.52311668573725,-0.914271198507795));
#24749=CARTESIAN_POINT('Ctrl Pts',(98.3768433345683,1.50920926710067,-0.937050434558558));
#24750=CARTESIAN_POINT('Ctrl Pts',(98.3652794628307,1.41936610879395,-1.07701513562128));
#24751=CARTESIAN_POINT('Ctrl Pts',(98.3550641054095,1.33035544637778,-1.18520161856188));
#24752=CARTESIAN_POINT('Ctrl Pts',(98.3394501219947,1.1760901985898,-1.33318366193406));
#24753=CARTESIAN_POINT('Ctrl Pts',(98.3340642890454,1.11938805249025,-1.38113696148111));
#24754=CARTESIAN_POINT('Ctrl Pts',(98.3275965216838,1.04537659153359,-1.43616748804243));
#24755=CARTESIAN_POINT('Ctrl Pts',(98.3263431814397,1.03074126028944,-1.44670722292181));
#24756=CARTESIAN_POINT('Ctrl Pts',(98.3244933039316,1.00866356401447,-1.46210147495414));
#24757=CARTESIAN_POINT('Ctrl Pts',(98.3238863674541,1.00134168787206,-1.46712567323955));
#24758=CARTESIAN_POINT('Ctrl Pts',(98.3228442049251,0.988628256098838,-1.47570998774132));
#24759=CARTESIAN_POINT('Ctrl Pts',(98.3224073046791,0.983254637283262,-1.47929581848026));
#24760=CARTESIAN_POINT('Ctrl Pts',(98.3213810435232,0.970528645119562,-1.48768792460388));
#24761=CARTESIAN_POINT('Ctrl Pts',(98.3207933377285,0.963160043479178,-1.49246907868839));
#24762=CARTESIAN_POINT('Ctrl Pts',(98.3190783443929,0.941430787727218,-1.50634025874099));
#24763=CARTESIAN_POINT('Ctrl Pts',(98.317960326134,0.926974335617681,-1.5152793591475));
#24764=CARTESIAN_POINT('Ctrl Pts',(98.3096365204388,0.817359668665095,-1.58090324273059));
#24765=CARTESIAN_POINT('Ctrl Pts',(98.3028801393751,0.717201749197308,-1.62879100508618));
#24766=CARTESIAN_POINT('Ctrl Pts',(98.2898535083788,0.518035788211802,-1.70205456398339));
#24767=CARTESIAN_POINT('Ctrl Pts',(98.2836121332032,0.420033608408203,-1.72884926171801));
#24768=CARTESIAN_POINT('Ctrl Pts',(98.2750979641418,0.289384626960589,-1.75279992892654));
#24769=CARTESIAN_POINT('Ctrl Pts',(98.2730621396235,0.258339959894389,-1.75764368547648));
#24770=CARTESIAN_POINT('Ctrl Pts',(98.269970593612,0.211616922047383,-1.76366910864739));
#24771=CARTESIAN_POINT('Ctrl Pts',(98.2689342835042,0.196023722010649,-1.76547022645596));
#24772=CARTESIAN_POINT('Ctrl Pts',(98.2670465068762,0.167757246598624,-1.76835610293289));
#24773=CARTESIAN_POINT('Ctrl Pts',(98.2661973355244,0.15509217009072,-1.7695118549669));
#24774=CARTESIAN_POINT('Ctrl Pts',(98.2643531703054,0.127702105482516,-1.77171502668333));
#24775=CARTESIAN_POINT('Ctrl Pts',(98.2633567517855,0.112974377992038,-1.77271507312335));
#24776=CARTESIAN_POINT('Ctrl Pts',(98.2605948383426,0.0723586769443952,
-1.7749647853012));
#24777=CARTESIAN_POINT('Ctrl Pts',(98.2588175748128,0.0464540697977625,
-1.77583154129507));
#24778=CARTESIAN_POINT('Ctrl Pts',(98.2478448323583,-0.112002047341471,
-1.77766408290553));
#24779=CARTESIAN_POINT('Ctrl Pts',(98.238205264741,-0.244277910121359,-1.76435544837809));
#24780=CARTESIAN_POINT('Ctrl Pts',(98.223832924817,-0.436403834762349,-1.72299579622583));
#24781=CARTESIAN_POINT('Ctrl Pts',(98.2191578161576,-0.498220721826873,
-1.70614764806835));
#24782=CARTESIAN_POINT('Ctrl Pts',(98.21209137115,-0.592034120180635,-1.67504363813668));
#24783=CARTESIAN_POINT('Ctrl Pts',(98.2096333631561,-0.624746110059658,
-1.66312003979795));
#24784=CARTESIAN_POINT('Ctrl Pts',(98.206435404249,-0.667657169603206,-1.64603382752091));
#24785=CARTESIAN_POINT('Ctrl Pts',(98.2056529700315,-0.678185084900449,
-1.64172423543386));
#24786=CARTESIAN_POINT('Ctrl Pts',(98.2043650002294,-0.695575021505212,
-1.63440984659287));
#24787=CARTESIAN_POINT('Ctrl Pts',(98.2038561949455,-0.702460609193973,
-1.63146230633669));
#24788=CARTESIAN_POINT('Ctrl Pts',(98.2028256784177,-0.716442723950815,
-1.62537199317396));
#24789=CARTESIAN_POINT('Ctrl Pts',(98.202304159467,-0.723537654254827,-1.62222611296702));
#24790=CARTESIAN_POINT('Ctrl Pts',(98.2009398865599,-0.742139755598212,
-1.61383165132288));
#24791=CARTESIAN_POINT('Ctrl Pts',(98.2001016361212,-0.75361212478544,-1.60850638910493));
#24792=CARTESIAN_POINT('Ctrl Pts',(98.1963668658106,-0.804860294422662,
-1.58404924868774));
#24793=CARTESIAN_POINT('Ctrl Pts',(98.1935428635928,-0.843974861475339,
-1.5635598011405));
#24794=CARTESIAN_POINT('Ctrl Pts',(98.1847558318783,-0.965095747324518,
-1.4942413430828));
#24795=CARTESIAN_POINT('Ctrl Pts',(98.1789641534986,-1.0439542722814,-1.44025294342655));
#24796=CARTESIAN_POINT('Ctrl Pts',(98.1676266807647,-1.18705611781828,-1.32432540184134));
#24797=CARTESIAN_POINT('Ctrl Pts',(98.1621075802911,-1.25172333746431,-1.26337885229478));
#24798=CARTESIAN_POINT('Ctrl Pts',(98.1546796392565,-1.3294126995913,-1.17831514815713));
#24799=CARTESIAN_POINT('Ctrl Pts',(98.1529566238408,-1.34682338263695,-1.15837445215766));
#24800=CARTESIAN_POINT('Ctrl Pts',(98.1502465623942,-1.37321598920205,-1.12674697635486));
#24801=CARTESIAN_POINT('Ctrl Pts',(98.1492722548657,-1.38250946637842,-1.11532437216522));
#24802=CARTESIAN_POINT('Ctrl Pts',(98.147445560409,-1.39956424930796,-1.09382164108728));
#24803=CARTESIAN_POINT('Ctrl Pts',(98.1465946862198,-1.40736140904762,-1.083771064498));
#24804=CARTESIAN_POINT('Ctrl Pts',(98.1446810272647,-1.42456575191729,-1.06109581886622));
#24805=CARTESIAN_POINT('Ctrl Pts',(98.1436160324964,-1.43391428335433,-1.0484282133084));
#24806=CARTESIAN_POINT('Ctrl Pts',(98.1408651139608,-1.45747773056723,-1.01559412229908));
#24807=CARTESIAN_POINT('Ctrl Pts',(98.1391698945206,-1.47144267951145,-0.995253279818638));
#24808=CARTESIAN_POINT('Ctrl Pts',(98.1299299124651,-1.54455691133181,-0.883853881162364));
#24809=CARTESIAN_POINT('Ctrl Pts',(98.1220999265996,-1.59567665629541,-0.787821499273327));
#24810=CARTESIAN_POINT('Ctrl Pts',(98.1083156442436,-1.66874288259566,-0.613830041084897));
#24811=CARTESIAN_POINT('Ctrl Pts',(98.1024276197712,-1.69474280435508,-0.537901312946196));
#24812=CARTESIAN_POINT('Ctrl Pts',(98.0947504353423,-1.72247193898184,-0.434594604369087));
#24813=CARTESIAN_POINT('Ctrl Pts',(98.0928436333156,-1.72883222985613,-0.408560062187443));
#24814=CARTESIAN_POINT('Ctrl Pts',(98.0896073294105,-1.73874857958756,-0.363577448623549));
#24815=CARTESIAN_POINT('Ctrl Pts',(98.0882664394465,-1.74258972100933,-0.344697438010488));
#24816=CARTESIAN_POINT('Ctrl Pts',(98.0863142891777,-1.74779435486674,-0.316799615883821));
#24817=CARTESIAN_POINT('Ctrl Pts',(98.0856909587469,-1.74939667284509,-0.307828513503592));
#24818=CARTESIAN_POINT('Ctrl Pts',(98.0845837905023,-1.75213691597315,-0.291773468410792));
#24819=CARTESIAN_POINT('Ctrl Pts',(98.0840985555096,-1.75330104728428,-0.284694523845136));
#24820=CARTESIAN_POINT('Ctrl Pts',(98.0830153387652,-1.7558166922319,-0.268796210864844));
#24821=CARTESIAN_POINT('Ctrl Pts',(98.0824186616965,-1.75714468546585,-0.25997350361966));
#24822=CARTESIAN_POINT('Ctrl Pts',(98.0806117904877,-1.76098691092547,-0.233071504715948));
#24823=CARTESIAN_POINT('Ctrl Pts',(98.0794126603786,-1.76328908890409,-0.21496250692346));
#24824=CARTESIAN_POINT('Ctrl Pts',(98.0728680335193,-1.77444059774624,-0.114942937855293));
#24825=CARTESIAN_POINT('Ctrl Pts',(98.0677612371266,-1.77786302348111,-0.0325196174557306));
#24826=CARTESIAN_POINT('Ctrl Pts',(98.0542092851574,-1.77168138552039,0.187649300816255));
#24827=CARTESIAN_POINT('Ctrl Pts',(98.0458418052931,-1.7517860784445,0.324513006834991));
#24828=CARTESIAN_POINT('Ctrl Pts',(98.0353107137848,-1.70974651376196,0.482153117889082));
#24829=CARTESIAN_POINT('Ctrl Pts',(98.03366182822,-1.7027024226322,0.506467300088243));
#24830=CARTESIAN_POINT('Ctrl Pts',(98.0310334389136,-1.69077085320271,0.544584281928687));
#24831=CARTESIAN_POINT('Ctrl Pts',(98.0300651751099,-1.6862279912027,0.558491950076518));
#24832=CARTESIAN_POINT('Ctrl Pts',(98.0282438568472,-1.67741244524881,0.584391630116195));
#24833=CARTESIAN_POINT('Ctrl Pts',(98.0273922357488,-1.67318161729964,0.596396973323348));
#24834=CARTESIAN_POINT('Ctrl Pts',(98.0254689627225,-1.66338615754936,0.62326757727564));
#24835=CARTESIAN_POINT('Ctrl Pts',(98.0243949998835,-1.65775062836051,0.638105639848719));
#24836=CARTESIAN_POINT('Ctrl Pts',(98.0211111458412,-1.6400238472746,0.682958923629991));
#24837=CARTESIAN_POINT('Ctrl Pts',(98.0188806765523,-1.6273111628562,0.712719616732592));
#24838=CARTESIAN_POINT('Ctrl Pts',(98.0106019595959,-1.57771725409396,0.820565890651796));
#24839=CARTESIAN_POINT('Ctrl Pts',(98.0043977721695,-1.53597321104229,0.896271650262331));
#24840=CARTESIAN_POINT('Ctrl Pts',(97.9903054138692,-1.43047117226747,1.05843984856373));
#24841=CARTESIAN_POINT('Ctrl Pts',(97.9823954532755,-1.36403934787121,1.14277769929264));
#24842=CARTESIAN_POINT('Ctrl Pts',(97.9727294385042,-1.27064827168052,1.24150877886826));
#24843=CARTESIAN_POINT('Ctrl Pts',(97.970707315795,-1.25038037092677,1.26191926518674));
#24844=CARTESIAN_POINT('Ctrl Pts',(97.9679625986899,-1.22174048663087,1.28939272494242));
#24845=CARTESIAN_POINT('Ctrl Pts',(97.9672118533408,-1.21378668231616,1.29688292490814));
#24846=CARTESIAN_POINT('Ctrl Pts',(97.9659665193693,-1.20038287707994,1.30927411740428));
#24847=CARTESIAN_POINT('Ctrl Pts',(97.9654689886107,-1.19497082297416,1.31421554776976));
#24848=CARTESIAN_POINT('Ctrl Pts',(97.964442223177,-1.18368010785411,1.32439702272067));
#24849=CARTESIAN_POINT('Ctrl Pts',(97.9639133722064,-1.17779694215291,1.32963169360216));
#24850=CARTESIAN_POINT('Ctrl Pts',(97.9625073710163,-1.16198092568197,1.3435169799523));
#24851=CARTESIAN_POINT('Ctrl Pts',(97.9616352344026,-1.15198612211205,1.35209672251745));
#24852=CARTESIAN_POINT('Ctrl Pts',(97.9570487077875,-1.09850509111268,1.39698234556685));
#24853=CARTESIAN_POINT('Ctrl Pts',(97.9534564902755,-1.05339165488499,1.43130726617521));
#24854=CARTESIAN_POINT('Ctrl Pts',(97.945185801493,-0.944185678737328,1.50643180065365));
#24855=CARTESIAN_POINT('Ctrl Pts',(97.9405591773055,-0.878966951924941,
1.54539356479032));
#24856=CARTESIAN_POINT('Ctrl Pts',(97.929629373244,-0.720839677627748,1.62660098704003));
#24857=CARTESIAN_POINT('Ctrl Pts',(97.9233069362445,-0.62640163384933,1.66525010040541));
#24858=CARTESIAN_POINT('Ctrl Pts',(97.9152413107957,-0.507617572906279,
1.70232154741751));
#24859=CARTESIAN_POINT('Ctrl Pts',(97.9137649937122,-0.485930335010842,
1.70863860579432));
#24860=CARTESIAN_POINT('Ctrl Pts',(97.9113573006744,-0.450694205457453,
1.71817709357557));
#24861=CARTESIAN_POINT('Ctrl Pts',(97.9104343016002,-0.437217148970669,
1.72165587087046));
#24862=CARTESIAN_POINT('Ctrl Pts',(97.9086474557629,-0.411195807127017,
1.72804741926426));
#24863=CARTESIAN_POINT('Ctrl Pts',(97.9077844044879,-0.398657958101282,
1.73098286887631));
#24864=CARTESIAN_POINT('Ctrl Pts',(97.9057602392808,-0.369330770826302,
1.73751363433028));
#24865=CARTESIAN_POINT('Ctrl Pts',(97.9045957904995,-0.352519266985833,
1.74100229120531));
#24866=CARTESIAN_POINT('Ctrl Pts',(97.9006964974025,-0.296439978558571,
1.7517941097598));
#24867=CARTESIAN_POINT('Ctrl Pts',(97.8979281115964,-0.256979177285258,
1.75801607637832));
#24868=CARTESIAN_POINT('Ctrl Pts',(97.8909912461611,-0.159013821258514,
1.77009403424395));
#24869=CARTESIAN_POINT('Ctrl Pts',(97.8867815991976,-0.100367001062135,
1.77438542427143));
#24870=CARTESIAN_POINT('Ctrl Pts',(97.8742659603391,0.0722684173030461,
1.7784316221213));
#24871=CARTESIAN_POINT('Ctrl Pts',(97.8658356941724,0.186146864378722,1.77013868261274));
#24872=CARTESIAN_POINT('Ctrl Pts',(97.8550772581095,0.334221250188591,1.74490035263605));
#24873=CARTESIAN_POINT('Ctrl Pts',(97.8525099053,0.369803807893793,1.73770729657601));
#24874=CARTESIAN_POINT('Ctrl Pts',(97.8491695754232,0.416718218583295,1.7267169172412));
#24875=CARTESIAN_POINT('Ctrl Pts',(97.8483510348131,0.428265698665458,1.72388917762427));
#24876=CARTESIAN_POINT('Ctrl Pts',(97.8470711401953,0.446415923645576,1.71925092291531));
#24877=CARTESIAN_POINT('Ctrl Pts',(97.846605593857,0.453037831890558,1.71751787173543));
#24878=CARTESIAN_POINT('Ctrl Pts',(97.8456375832112,0.466852080647597,1.71381702485344));
#24879=CARTESIAN_POINT('Ctrl Pts',(97.8451355773905,0.474042319213878,1.71184214878116));
#24880=CARTESIAN_POINT('Ctrl Pts',(97.8438853100209,0.492009119869962,1.70678549142416));
#24881=CARTESIAN_POINT('Ctrl Pts',(97.843140245577,0.502769587967576,1.70364680770171));
#24882=CARTESIAN_POINT('Ctrl Pts',(97.8401984756198,0.545431741698417,1.6907634082199));
#24883=CARTESIAN_POINT('Ctrl Pts',(97.838042826499,0.577087995457027,1.680222148401));
#24884=CARTESIAN_POINT('Ctrl Pts',(97.8321180859629,0.66449869191991,1.64835282213077));
#24885=CARTESIAN_POINT('Ctrl Pts',(97.8284209059208,0.719504709059385,1.62509676327981));
#24886=CARTESIAN_POINT('Ctrl Pts',(97.8161060884032,0.899612536774803,1.5380070647654));
#24887=CARTESIAN_POINT('Ctrl Pts',(97.807595170684,1.01828400274892,1.46214299419755));
#24888=CARTESIAN_POINT('Ctrl Pts',(97.7969174290843,1.14610632363562,1.35725053249853));
#24889=CARTESIAN_POINT('Ctrl Pts',(97.7952887999147,1.16508921265166,1.34099058125209));
#24890=CARTESIAN_POINT('Ctrl Pts',(97.7926854511532,1.1945785945918,1.31463229641913));
#24891=CARTESIAN_POINT('Ctrl Pts',(97.791721606471,1.20531517550429,1.3047955394964));
#24892=CARTESIAN_POINT('Ctrl Pts',(97.7899122073739,1.22512541035748,1.28619241744018));
#24893=CARTESIAN_POINT('Ctrl Pts',(97.789068107955,1.23422900830743,1.27745917612038));
#24894=CARTESIAN_POINT('Ctrl Pts',(97.7871498418919,1.25460151602236,1.25749441867292));
#24895=CARTESIAN_POINT('Ctrl Pts',(97.7860732558245,1.26581396448494,1.24620710780207));
#24896=CARTESIAN_POINT('Ctrl Pts',(97.7827726543576,1.29950883591614,1.2113633433446));
#24897=CARTESIAN_POINT('Ctrl Pts',(97.7805277507915,1.32149536371475,1.18733909448381));
#24898=CARTESIAN_POINT('Ctrl Pts',(97.7720276424793,1.40125802460095,1.09522281927296));
#24899=CARTESIAN_POINT('Ctrl Pts',(97.7656040654292,1.45452714375907,1.02341780103985));
#24900=CARTESIAN_POINT('Ctrl Pts',(97.7508671869894,1.56241181947067,0.852453555950466));
#24901=CARTESIAN_POINT('Ctrl Pts',(97.7425304549368,1.61342038204608,0.751455225819273));
#24902=CARTESIAN_POINT('Ctrl Pts',(97.7330012546246,1.6625408141901,0.62570806089402));
#24903=CARTESIAN_POINT('Ctrl Pts',(97.731456761187,1.6701980292724,0.604972056208978));
#24904=CARTESIAN_POINT('Ctrl Pts',(97.7293152066599,1.68040887706859,0.57564757016288));
#24905=CARTESIAN_POINT('Ctrl Pts',(97.7287014301601,1.68328732009332,0.567175392340083));
#24906=CARTESIAN_POINT('Ctrl Pts',(97.7275950720059,1.68839041301477,0.551774252266665));
#24907=CARTESIAN_POINT('Ctrl Pts',(97.7271012790119,1.69063673414047,0.544852689532012));
#24908=CARTESIAN_POINT('Ctrl Pts',(97.7260715087293,1.69525640007447,0.530314471369937));
#24909=CARTESIAN_POINT('Ctrl Pts',(97.7255360236156,1.69762106372693,0.522695351808296));
#24910=CARTESIAN_POINT('Ctrl Pts',(97.7240922344492,1.7038913599639,0.50200051160188));
#24911=CARTESIAN_POINT('Ctrl Pts',(97.7231894240966,1.70769786490648,0.488894989321775));
#24912=CARTESIAN_POINT('Ctrl Pts',(97.7179510521506,1.72907912288824,0.411982412822237));
#24913=CARTESIAN_POINT('Ctrl Pts',(97.7137830337753,1.74322969857604,0.347269867565681));
#24914=CARTESIAN_POINT('Ctrl Pts',(97.7028272905171,1.77125343325277,0.172937823174047));
#24915=CARTESIAN_POINT('Ctrl Pts',(97.6961636456077,1.77856389059651,0.0626439766106631));
#24916=CARTESIAN_POINT('Ctrl Pts',(97.6892780533294,1.77561363837197,-0.0475422940912402));
#24917=CARTESIAN_POINT('Ctrl Pts',(97.5395352881717,1.77561363837197,-0.0475422940912293));
#24918=CARTESIAN_POINT('Ctrl Pts',(97.5419371591145,1.77663884788498,-0.00925268210916231));
#24919=CARTESIAN_POINT('Ctrl Pts',(97.5443657489703,1.77642598817633,0.0290864244276453));
#24920=CARTESIAN_POINT('Ctrl Pts',(97.5485161025327,1.77397510500667,0.0936151268840668));
#24921=CARTESIAN_POINT('Ctrl Pts',(97.5502168588313,1.77240010659219,0.11978820531831));
#24922=CARTESIAN_POINT('Ctrl Pts',(97.5529909444832,1.76892359461123,0.161965152295464));
#24923=CARTESIAN_POINT('Ctrl Pts',(97.5540530881059,1.76738253788206,0.17799531035738));
#24924=CARTESIAN_POINT('Ctrl Pts',(97.5559608844456,1.76424373587094,0.20656175374763));
#24925=CARTESIAN_POINT('Ctrl Pts',(97.5568038472848,1.76272974329664,0.219106265535949));
#24926=CARTESIAN_POINT('Ctrl Pts',(97.5586047728816,1.75922729330079,0.245735003006639));
#24927=CARTESIAN_POINT('Ctrl Pts',(97.5595638059636,1.75720324726604,0.259813564836092));
#24928=CARTESIAN_POINT('Ctrl Pts',(97.5621876949148,1.75123713904399,0.298046071965117));
#24929=CARTESIAN_POINT('Ctrl Pts',(97.563862850041,1.74696473512794,0.322144514392271));
#24930=CARTESIAN_POINT('Ctrl Pts',(97.5676359893372,1.73632160857712,0.375712700358774));
#24931=CARTESIAN_POINT('Ctrl Pts',(97.5697413781647,1.72969579651495,0.405123473296547));
#24932=CARTESIAN_POINT('Ctrl Pts',(97.5767108102229,1.70553644330522,0.500922401396418));
#24933=CARTESIAN_POINT('Ctrl Pts',(97.5816592184252,1.6849036034178,0.566459204399034));
#24934=CARTESIAN_POINT('Ctrl Pts',(97.5943815227014,1.62288313963923,0.729766755464741));
#24935=CARTESIAN_POINT('Ctrl Pts',(97.6022100834227,1.57643155989748,0.825332716883103));
#24936=CARTESIAN_POINT('Ctrl Pts',(97.6119127418899,1.50616454494463,0.94204207464389));
#24937=CARTESIAN_POINT('Ctrl Pts',(97.6140373124276,1.48994008014055,0.967498693342539));
#24938=CARTESIAN_POINT('Ctrl Pts',(97.6168904853991,1.46689745526781,1.00169760258894));
#24939=CARTESIAN_POINT('Ctrl Pts',(97.6176503194918,1.4606356450365,1.01080648965644));
#24940=CARTESIAN_POINT('Ctrl Pts',(97.6188580289242,1.45047475921969,1.02529564855163));
#24941=CARTESIAN_POINT('Ctrl Pts',(97.6193093973346,1.44662994089237,1.03071335098042));
#24942=CARTESIAN_POINT('Ctrl Pts',(97.6202677494203,1.43836332744599,1.0422243892309));
#24943=CARTESIAN_POINT('Ctrl Pts',(97.6207741207522,1.43393298470018,1.04831147081946));
#24944=CARTESIAN_POINT('Ctrl Pts',(97.6220676914719,1.42245863229558,1.06386783915769));
#24945=CARTESIAN_POINT('Ctrl Pts',(97.6228511360397,1.41535857672785,1.0732956059689));
#24946=CARTESIAN_POINT('Ctrl Pts',(97.6262364311107,1.38404880857153,1.11401903865881));
#24947=CARTESIAN_POINT('Ctrl Pts',(97.6287796051157,1.35888937072073,1.14457403951826));
#24948=CARTESIAN_POINT('Ctrl Pts',(97.6363732945961,1.27954562341276,1.23462492415807));
#24949=CARTESIAN_POINT('Ctrl Pts',(97.6412942118059,1.22232038627018,1.29130565102304));
#24950=CARTESIAN_POINT('Ctrl Pts',(97.6528943333001,1.07933979279307,1.41487324220862));
#24951=CARTESIAN_POINT('Ctrl Pts',(97.6595738775348,0.990912780022458,1.47815053604306));
#24952=CARTESIAN_POINT('Ctrl Pts',(97.6681462996586,0.876053427730697,1.54537983734966));
#24953=CARTESIAN_POINT('Ctrl Pts',(97.669743790925,0.854581734495018,1.55735622601384));
#24954=CARTESIAN_POINT('Ctrl Pts',(97.6723829283067,0.819058799598392,1.57621420620339));
#24955=CARTESIAN_POINT('Ctrl Pts',(97.6734151429244,0.805152563404083,1.58336283415792));
#24956=CARTESIAN_POINT('Ctrl Pts',(97.6752905940369,0.779876724830942,1.59593703245233));
#24957=CARTESIAN_POINT('Ctrl Pts',(97.6761315061215,0.768540221872781,1.60142706071519));
#24958=CARTESIAN_POINT('Ctrl Pts',(97.6779519523262,0.743997947403623,1.61299175144776));
#24959=CARTESIAN_POINT('Ctrl Pts',(97.6789328194399,0.730774156273614,1.61902577082223));
#24960=CARTESIAN_POINT('Ctrl Pts',(97.6816827530199,0.69370992947995,1.63539159451465));
#24961=CARTESIAN_POINT('Ctrl Pts',(97.6834638575235,0.66971547610311,1.6453632395989));
#24962=CARTESIAN_POINT('Ctrl Pts',(97.6912067650428,0.565507598330987,1.68601301631867));
#24963=CARTESIAN_POINT('Ctrl Pts',(97.6973376590116,0.483356649309191,1.7113741070999));
#24964=CARTESIAN_POINT('Ctrl Pts',(97.7133949114326,0.267890982706294,1.76113600589286));
#24965=CARTESIAN_POINT('Ctrl Pts',(97.7234461675429,0.133029388472,1.7764209467011));
#24966=CARTESIAN_POINT('Ctrl Pts',(97.734130235588,-0.0195114170905297,
1.77622658066348));
#24967=CARTESIAN_POINT('Ctrl Pts',(97.7353277997537,-0.0367591355060871,
1.77595337285126));
#24968=CARTESIAN_POINT('Ctrl Pts',(97.7371085722954,-0.0626713220210358,
1.77516523550523));
#24969=CARTESIAN_POINT('Ctrl Pts',(97.7377012095291,-0.0713399088181698,
1.7748380019945));
#24970=CARTESIAN_POINT('Ctrl Pts',(97.7387246484473,-0.0863944557493178,
1.77415922513816));
#24971=CARTESIAN_POINT('Ctrl Pts',(97.7391569976615,-0.0927812395864988,
1.7738366900193));
#24972=CARTESIAN_POINT('Ctrl Pts',(97.7401796429339,-0.107951766937579,
1.77298840974542));
#24973=CARTESIAN_POINT('Ctrl Pts',(97.7407682320153,-0.116733514956201,
1.77243188297211));
#24974=CARTESIAN_POINT('Ctrl Pts',(97.7425430882662,-0.143353011900473,
1.77054621837499));
#24975=CARTESIAN_POINT('Ctrl Pts',(97.7437187554771,-0.161175761214322,
1.76901284098851));
#24976=CARTESIAN_POINT('Ctrl Pts',(97.7496638677273,-0.252072048401022,
1.75980737631326));
#24977=CARTESIAN_POINT('Ctrl Pts',(97.7542443637918,-0.324649670041035,
1.74787507905684));
#24978=CARTESIAN_POINT('Ctrl Pts',(97.7672302606924,-0.529853785421857,
1.70090969337469));
#24979=CARTESIAN_POINT('Ctrl Pts',(97.7755096034912,-0.659424547624919,
1.65499112923024));
#24980=CARTESIAN_POINT('Ctrl Pts',(97.7863282871474,-0.811013741753595,
1.58061211328096));
#24981=CARTESIAN_POINT('Ctrl Pts',(97.7883909653162,-0.83921574793287,1.56582076550653));
#24982=CARTESIAN_POINT('Ctrl Pts',(97.7915089503022,-0.880690907666014,
1.54262552864903));
#24983=CARTESIAN_POINT('Ctrl Pts',(97.7925441365659,-0.894275778080294,
1.53479014947032));
#24984=CARTESIAN_POINT('Ctrl Pts',(97.7944227449241,-0.918584233923626,
1.52033739752042));
#24985=CARTESIAN_POINT('Ctrl Pts',(97.7952638062974,-0.92934464196915,1.51378377567218));
#24986=CARTESIAN_POINT('Ctrl Pts',(97.7970820480227,-0.952338182849639,
1.49944200697914));
#24987=CARTESIAN_POINT('Ctrl Pts',(97.7980605332358,-0.964547406860139,
1.4916174526218));
#24988=CARTESIAN_POINT('Ctrl Pts',(97.8007966202541,-0.998222518607995,
1.46944967161701));
#24989=CARTESIAN_POINT('Ctrl Pts',(97.8025660632571,-1.01947281200129,1.45478713133355));
#24990=CARTESIAN_POINT('Ctrl Pts',(97.8102111703715,-1.10900676781338,1.39008420687031));
#24991=CARTESIAN_POINT('Ctrl Pts',(97.8162508842426,-1.17397655159482,1.33566671001694));
#24992=CARTESIAN_POINT('Ctrl Pts',(97.831824961299,-1.32823187249575,1.18648789955951));
#24993=CARTESIAN_POINT('Ctrl Pts',(97.8414719049959,-1.41145456906662,1.08616346200528));
#24994=CARTESIAN_POINT('Ctrl Pts',(97.8521686221026,-1.49496269204481,0.959491499160685));
#24995=CARTESIAN_POINT('Ctrl Pts',(97.8536871265767,-1.50660326010684,0.941107916194747));
#24996=CARTESIAN_POINT('Ctrl Pts',(97.8558335719247,-1.52278578444251,0.914481207540025));
#24997=CARTESIAN_POINT('Ctrl Pts',(97.8564774304237,-1.5276041168009,0.906409453027667));
#24998=CARTESIAN_POINT('Ctrl Pts',(97.8576029567433,-1.53596740339845,0.892142997385941));
#24999=CARTESIAN_POINT('Ctrl Pts',(97.8580862998257,-1.53953943476725,0.885964631158831));
#25000=CARTESIAN_POINT('Ctrl Pts',(97.8591330234127,-1.54723311129706,0.872470208562674));
#25001=CARTESIAN_POINT('Ctrl Pts',(97.8596954999529,-1.55134022588294,0.865146274506095));
#25002=CARTESIAN_POINT('Ctrl Pts',(97.8613119503521,-1.56305815395625,0.843898718956846));
#25003=CARTESIAN_POINT('Ctrl Pts',(97.8623579165958,-1.57053475409258,0.829901481934332));
#25004=CARTESIAN_POINT('Ctrl Pts',(97.8647496378755,-1.58735257787546,0.797374665358724));
#25005=CARTESIAN_POINT('Ctrl Pts',(97.8660884833351,-1.59655883494904,0.77877758581373));
#25006=CARTESIAN_POINT('Ctrl Pts',(97.870710858708,-1.62750783232141,0.713402320511595));
#25007=CARTESIAN_POINT('Ctrl Pts',(97.873926323244,-1.64753850443317,0.665839480513909));
#25008=CARTESIAN_POINT('Ctrl Pts',(97.8848783852872,-1.70916172747797,0.499625976748066));
#25009=CARTESIAN_POINT('Ctrl Pts',(97.8924695072112,-1.74021948563971,0.377485083302912));
#25010=CARTESIAN_POINT('Ctrl Pts',(97.9030875904693,-1.76408419524224,0.211705443753069));
#25011=CARTESIAN_POINT('Ctrl Pts',(97.9057733424607,-1.76857821492427,0.170126171294622));
#25012=CARTESIAN_POINT('Ctrl Pts',(97.9096677871547,-1.77288887361713,0.110663428358246));
#25013=CARTESIAN_POINT('Ctrl Pts',(97.9108392467692,-1.773909438039,0.0928796004373038));
#25014=CARTESIAN_POINT('Ctrl Pts',(97.9128636357025,-1.77520132920039,0.0623448377334911));
#25015=CARTESIAN_POINT('Ctrl Pts',(97.9137124275394,-1.77560311037306,0.0496005839481933));
#25016=CARTESIAN_POINT('Ctrl Pts',(97.9154655531839,-1.77614671961305,0.0234054869731207));
#25017=CARTESIAN_POINT('Ctrl Pts',(97.9163703176002,-1.77627302615033,0.00995518283025552));
#25018=CARTESIAN_POINT('Ctrl Pts',(97.9186849738396,-1.77620568077855,-0.0242719771989726));
#25019=CARTESIAN_POINT('Ctrl Pts',(97.9201013790229,-1.77580025721604,-0.0450458849444988));
#25020=CARTESIAN_POINT('Ctrl Pts',(97.9265405207018,-1.77232872463862,-0.13868428019974));
#25021=CARTESIAN_POINT('Ctrl Pts',(97.9316887876581,-1.76514175187097,-0.211316225055452));
#25022=CARTESIAN_POINT('Ctrl Pts',(97.9449346441887,-1.73578302168071,-0.39303942032962));
#25023=CARTESIAN_POINT('Ctrl Pts',(97.9531457576869,-1.70778877041243,-0.500877128334812));
#25024=CARTESIAN_POINT('Ctrl Pts',(97.9650795568703,-1.65163205468216,-0.655781760095029));
#25025=CARTESIAN_POINT('Ctrl Pts',(97.968915515068,-1.63108616642553,-0.70533482489542));
#25026=CARTESIAN_POINT('Ctrl Pts',(97.9735688370383,-1.60268587940883,-0.765923460623624));
#25027=CARTESIAN_POINT('Ctrl Pts',(97.9744865151198,-1.59690867674238,-0.777896831412046));
#25028=CARTESIAN_POINT('Ctrl Pts',(97.9759338604355,-1.58750611361056,-0.796837531781246));
#25029=CARTESIAN_POINT('Ctrl Pts',(97.9764685573685,-1.58396816544437,-0.803847354723185));
#25030=CARTESIAN_POINT('Ctrl Pts',(97.9774951070953,-1.57704873424559,-0.81733391469048));
#25031=CARTESIAN_POINT('Ctrl Pts',(97.9779872989915,-1.57367361708345,-0.823813563396116));
#25032=CARTESIAN_POINT('Ctrl Pts',(97.9791940953441,-1.56525860227976,-0.839728521770535));
#25033=CARTESIAN_POINT('Ctrl Pts',(97.9799059040413,-1.56017316418026,-0.849139678885146));
#25034=CARTESIAN_POINT('Ctrl Pts',(97.9825799341316,-1.54061989690655,-0.884556362929399));
#25035=CARTESIAN_POINT('Ctrl Pts',(97.9845097940014,-1.52558350462171,-0.910244385996139));
#25036=CARTESIAN_POINT('Ctrl Pts',(97.9896095991787,-1.48358368731526,-0.978029371890028));
#25037=CARTESIAN_POINT('Ctrl Pts',(97.9927293480249,-1.45547641781806,-1.01938760093204));
#25038=CARTESIAN_POINT('Ctrl Pts',(98.0032291458754,-1.35419747768202,-1.15566727830361));
#25039=CARTESIAN_POINT('Ctrl Pts',(98.0104663588623,-1.27319245677475,-1.24434645446463));
#25040=CARTESIAN_POINT('Ctrl Pts',(98.0210429073214,-1.14817566122535,-1.35611586141513));
#25041=CARTESIAN_POINT('Ctrl Pts',(98.0241064242361,-1.1111995582421,-1.38657581964405));
#25042=CARTESIAN_POINT('Ctrl Pts',(98.0284505427962,-1.05811459247464,-1.42681756799562));
#25043=CARTESIAN_POINT('Ctrl Pts',(98.0296806365348,-1.04301128094236,-1.43789508901444));
#25044=CARTESIAN_POINT('Ctrl Pts',(98.0316968356135,-1.01816063391409,-1.45552424176401));
#25045=CARTESIAN_POINT('Ctrl Pts',(98.0324772860455,-1.00851827193534,-1.46222186370983));
#25046=CARTESIAN_POINT('Ctrl Pts',(98.0341296745711,-0.988060451087879,
-1.47613332941266));
#25047=CARTESIAN_POINT('Ctrl Pts',(98.0350023896007,-0.977230812993598,
-1.48332497577064));
#25048=CARTESIAN_POINT('Ctrl Pts',(98.0371277876091,-0.950803549775022,
-1.50045952808173));
#25049=CARTESIAN_POINT('Ctrl Pts',(98.038384960799,-0.93512794974577,-1.51027873521665));
#25050=CARTESIAN_POINT('Ctrl Pts',(98.0430764886706,-0.876489502391415,
-1.54574698986765));
#25051=CARTESIAN_POINT('Ctrl Pts',(98.0465664188311,-0.832605587350575,
-1.56981995490838));
#25052=CARTESIAN_POINT('Ctrl Pts',(98.0560740693701,-0.712387083414921,
-1.62930729761519));
#25053=CARTESIAN_POINT('Ctrl Pts',(98.0621874026624,-0.634459393613275,
-1.66120328586798));
#25054=CARTESIAN_POINT('Ctrl Pts',(98.0757177780561,-0.458646834427033,
-1.71898311839709));
#25055=CARTESIAN_POINT('Ctrl Pts',(98.0831285851693,-0.360198599004165,
-1.74227445631536));
#25056=CARTESIAN_POINT('Ctrl Pts',(98.0914517314965,-0.242741857388283,
-1.75967480493606));
#25057=CARTESIAN_POINT('Ctrl Pts',(98.0926847333336,-0.225147330882121,
-1.76201241987327));
#25058=CARTESIAN_POINT('Ctrl Pts',(98.0945071691658,-0.198807964918679,
-1.7651108757947));
#25059=CARTESIAN_POINT('Ctrl Pts',(98.0951066685777,-0.190088314238388,
-1.76607119102596));
#25060=CARTESIAN_POINT('Ctrl Pts',(98.0961850670182,-0.174296457946805,
-1.76769206889822));
#25061=CARTESIAN_POINT('Ctrl Pts',(98.0966651275992,-0.167227086390418,
-1.76837485033131));
#25062=CARTESIAN_POINT('Ctrl Pts',(98.097752993627,-0.151118188660109,-1.76983322932378));
#25063=CARTESIAN_POINT('Ctrl Pts',(98.0983593191796,-0.142076601695277,
-1.77058199888018));
#25064=CARTESIAN_POINT('Ctrl Pts',(98.1002466688599,-0.113749657320795,
-1.772709475433));
#25065=CARTESIAN_POINT('Ctrl Pts',(98.1015150361185,-0.0944465585079882,
-1.77384266246222));
#25066=CARTESIAN_POINT('Ctrl Pts',(98.1045222522783,-0.0481594669893906,
-1.77580216400853));
#25067=CARTESIAN_POINT('Ctrl Pts',(98.106248123938,-0.0211671023189207,
-1.77632901463453));
#25068=CARTESIAN_POINT('Ctrl Pts',(98.1131176827226,0.0874387578623564,
-1.7759726596306));
#25069=CARTESIAN_POINT('Ctrl Pts',(98.1181067590892,0.168939285567786,-1.77008070089214));
#25070=CARTESIAN_POINT('Ctrl Pts',(98.1296836064541,0.35565029070981,-1.7435647268776));
#25071=CARTESIAN_POINT('Ctrl Pts',(98.1362722839938,0.459963614353038,-1.71899246435281));
#25072=CARTESIAN_POINT('Ctrl Pts',(98.144745109016,0.58476420014083,-1.67741466052494));
#25073=CARTESIAN_POINT('Ctrl Pts',(98.1463434532876,0.607935970934208,-1.66915633597266));
#25074=CARTESIAN_POINT('Ctrl Pts',(98.1489837074697,0.645547762443126,-1.65486457139248));
#25075=CARTESIAN_POINT('Ctrl Pts',(98.1500161719442,0.660093192022824,-1.64911661655065));
#25076=CARTESIAN_POINT('Ctrl Pts',(98.1518918880881,0.686212867529391,-1.63839391614542));
#25077=CARTESIAN_POINT('Ctrl Pts',(98.1527328122948,0.697813810165198,-1.63348663793392));
#25078=CARTESIAN_POINT('Ctrl Pts',(98.1545530709162,0.722684517020114,-1.62265287132497));
#25079=CARTESIAN_POINT('Ctrl Pts',(98.1555337359409,0.73593562315748,-1.61668611320359));
#25080=CARTESIAN_POINT('Ctrl Pts',(98.1582824934228,0.772657363213013,-1.59960588896563));
#25081=CARTESIAN_POINT('Ctrl Pts',(98.1600626071388,0.795958889960783,-1.58813970484989));
#25082=CARTESIAN_POINT('Ctrl Pts',(98.1677971655269,0.895109510548429,-1.53661958927264));
#25083=CARTESIAN_POINT('Ctrl Pts',(98.1739202673956,0.968244157993132,-1.4916166768251));
#25084=CARTESIAN_POINT('Ctrl Pts',(98.1899829822579,1.14777658438383,-1.36236033822119));
#25085=CARTESIAN_POINT('Ctrl Pts',(98.2000488329196,1.24830444035904,-1.27088763640709));
#25086=CARTESIAN_POINT('Ctrl Pts',(98.2107428969953,1.34878504245925,-1.15591487250569));
#25087=CARTESIAN_POINT('Ctrl Pts',(98.2119378289671,1.35992248902994,-1.14279095291831));
#25088=CARTESIAN_POINT('Ctrl Pts',(98.2137155016879,1.37637927370779,-1.12281756133547));
#25089=CARTESIAN_POINT('Ctrl Pts',(98.2143076247235,1.38184174525249,-1.11608807007254));
#25090=CARTESIAN_POINT('Ctrl Pts',(98.2153305709726,1.39124895350104,-1.1043239163556));
#25091=CARTESIAN_POINT('Ctrl Pts',(98.2157629355758,1.39521596198389,-1.09930768459222));
#25092=CARTESIAN_POINT('Ctrl Pts',(98.2167861113364,1.4045815147121,-1.08733269592127));
#25093=CARTESIAN_POINT('Ctrl Pts',(98.2173752093448,1.40995550491436,-1.0803550830565));
#25094=CARTESIAN_POINT('Ctrl Pts',(98.2191532341675,1.42611049970892,-1.05905348993811));
#25095=CARTESIAN_POINT('Ctrl Pts',(98.2203315055686,1.43672712406474,-1.04460551570994));
#25096=CARTESIAN_POINT('Ctrl Pts',(98.2263036644115,1.48994984101678,-0.969828857736916));
#25097=CARTESIAN_POINT('Ctrl Pts',(98.2309066892802,1.5289865771356,-0.90703968983351));
#25098=CARTESIAN_POINT('Ctrl Pts',(98.2439885611737,1.6295265351328,-0.720287164590067));
#25099=CARTESIAN_POINT('Ctrl Pts',(98.2523414160577,1.68061428677739,-0.591357193237791));
#25100=CARTESIAN_POINT('Ctrl Pts',(98.2631585769089,1.72407792782382,-0.42842104542671));
#25101=CARTESIAN_POINT('Ctrl Pts',(98.2651305105155,1.73116113799823,-0.398836096408877));
#25102=CARTESIAN_POINT('Ctrl Pts',(98.2681508041026,1.74072437027604,-0.353816861656476));
#25103=CARTESIAN_POINT('Ctrl Pts',(98.2691813075371,1.74376626902148,-0.338506835867741));
#25104=CARTESIAN_POINT('Ctrl Pts',(98.2710549465546,1.74889721030061,-0.310775194624514));
#25105=CARTESIAN_POINT('Ctrl Pts',(98.2718957786435,1.75105667158789,-0.298367546198805));
#25106=CARTESIAN_POINT('Ctrl Pts',(98.2737175236098,1.75542703886347,-0.271572877420098));
#25107=CARTESIAN_POINT('Ctrl Pts',(98.2746997859108,1.7575933920722,-0.25717963111573));
#25108=CARTESIAN_POINT('Ctrl Pts',(98.2774578426196,1.76314687979346,-0.216926914012553));
#25109=CARTESIAN_POINT('Ctrl Pts',(98.2792457912219,1.7661416168894,-0.191017980664657));
#25110=CARTESIAN_POINT('Ctrl Pts',(98.2837696300757,1.77221356599926,-0.12595650345143));
#25111=CARTESIAN_POINT('Ctrl Pts',(98.2865256431726,1.77456345838068,-0.0867645056172716));
#25112=CARTESIAN_POINT('Ctrl Pts',(98.289313862947,1.77561363837197,-0.0475422940912524));
#25113=CARTESIAN_POINT('Origin',(88.3562164250559,0.,0.));
#25114=CARTESIAN_POINT('',(99.1886897733872,1.77561363837197,-0.04754229409124));
#25115=CARTESIAN_POINT('',(99.0420054636133,1.77561363839331,-0.0475422932941635));
#25116=CARTESIAN_POINT('',(88.3562164250559,1.77561363837197,-0.0475422940912398));
#25117=CARTESIAN_POINT('Ctrl Pts',(99.1886897733872,1.77561363837197,-0.0475422940912343));
#25118=CARTESIAN_POINT('Ctrl Pts',(99.1853655918391,1.7743934007775,-0.0931158314270797));
#25119=CARTESIAN_POINT('Ctrl Pts',(99.1820232071228,1.77141824310023,-0.138656366478061));
#25120=CARTESIAN_POINT('Ctrl Pts',(99.1747180039858,1.76105271532418,-0.238147712229466));
#25121=CARTESIAN_POINT('Ctrl Pts',(99.1707654191669,1.75293685978064,-0.291948735364658));
#25122=CARTESIAN_POINT('Ctrl Pts',(99.1646454542468,1.73624645399278,-0.376168724526229));
#25123=CARTESIAN_POINT('Ctrl Pts',(99.1624287111429,1.7293081351142,-0.406876298464051));
#25124=CARTESIAN_POINT('Ctrl Pts',(99.1594918742787,1.71885314255375,-0.448027341126179));
#25125=CARTESIAN_POINT('Ctrl Pts',(99.158737245475,1.71605069849231,-0.458644349977841));
#25126=CARTESIAN_POINT('Ctrl Pts',(99.1574823386392,1.71119192270817,-0.476383458904964));
#25127=CARTESIAN_POINT('Ctrl Pts',(99.1569791217336,1.70918916654739,-0.483519800167071));
#25128=CARTESIAN_POINT('Ctrl Pts',(99.1559464361303,1.7049653206176,-0.498216216129109));
#25129=CARTESIAN_POINT('Ctrl Pts',(99.1554172951155,1.70273850954039,-0.50577437332868));
#25130=CARTESIAN_POINT('Ctrl Pts',(99.1540095123898,1.69664847473252,-0.525948761124122));
#25131=CARTESIAN_POINT('Ctrl Pts',(99.1531359076543,1.69269476578993,-0.538537465406394));
#25132=CARTESIAN_POINT('Ctrl Pts',(99.1489103294804,1.67273655458295,-0.599692596467958));
#25133=CARTESIAN_POINT('Ctrl Pts',(99.145656479497,1.65477875901909,-0.647601022024729));
#25134=CARTESIAN_POINT('Ctrl Pts',(99.1322318050646,1.57092282876405,-0.844939786562546));
#25135=CARTESIAN_POINT('Ctrl Pts',(99.1225267294456,1.48665883891865,-0.985682789500896));
#25136=CARTESIAN_POINT('Ctrl Pts',(99.1098879580792,1.36269877248474,-1.13987296787201));
#25137=CARTESIAN_POINT('Ctrl Pts',(99.1076543331006,1.34026564081712,-1.16616726365281));
#25138=CARTESIAN_POINT('Ctrl Pts',(99.1043235309985,1.30616558520151,-1.20385222887757));
#25139=CARTESIAN_POINT('Ctrl Pts',(99.1032506721229,1.29508524292166,-1.21576433128528));
#25140=CARTESIAN_POINT('Ctrl Pts',(99.1013236362932,1.27502321056714,-1.2367468454062));
#25141=CARTESIAN_POINT('Ctrl Pts',(99.1004722067142,1.26610431724749,-1.24587591290242));
#25142=CARTESIAN_POINT('Ctrl Pts',(99.0986529540769,1.24693680553999,-1.265076724189));
#25143=CARTESIAN_POINT('Ctrl Pts',(99.097684037869,1.23666284915556,-1.27512175554073));
#25144=CARTESIAN_POINT('Ctrl Pts',(99.0950316486968,1.20836861635364,-1.30212192890378));
#25145=CARTESIAN_POINT('Ctrl Pts',(99.0933376417343,1.19011471043686,-1.31882640973637));
#25146=CARTESIAN_POINT('Ctrl Pts',(99.0816487282209,1.06298059048463,-1.43037995726261));
#25147=CARTESIAN_POINT('Ctrl Pts',(99.0711107372911,0.943252698267116,-1.51200966178706));
#25148=CARTESIAN_POINT('Ctrl Pts',(99.0549142438954,0.746329323859891,-1.61370069789504));
#25149=CARTESIAN_POINT('Ctrl Pts',(99.0492939992146,0.675409699749159,-1.64464627735572));
#25150=CARTESIAN_POINT('Ctrl Pts',(99.0425823107762,0.585426168804902,-1.67710382076618));
#25151=CARTESIAN_POINT('Ctrl Pts',(99.0413060112466,0.568062250892884,-1.68306457681726));
#25152=CARTESIAN_POINT('Ctrl Pts',(99.0394292726399,0.542107551231169,-1.69152694583775));
#25153=CARTESIAN_POINT('Ctrl Pts',(99.0388180051892,0.533585843355805,-1.69423438816787));
#25154=CARTESIAN_POINT('Ctrl Pts',(99.0377712990078,0.518869680928439,-1.69878782853164));
#25155=CARTESIAN_POINT('Ctrl Pts',(99.0373341366804,0.51268520247532,-1.70066449341263));
#25156=CARTESIAN_POINT('Ctrl Pts',(99.0363114049782,0.49812675834041,-1.70499558196026));
#25157=CARTESIAN_POINT('Ctrl Pts',(99.0357274421577,0.489744787357734,-1.70742210749768));
#25158=CARTESIAN_POINT('Ctrl Pts',(99.0340342100576,0.465250652675802,-1.7143177803379));
#25159=CARTESIAN_POINT('Ctrl Pts',(99.0329338610926,0.449092359875985,-1.71862146028356));
#25160=CARTESIAN_POINT('Ctrl Pts',(99.0243800590873,0.321829100888745,-1.75059986292592));
#25161=CARTESIAN_POINT('Ctrl Pts',(99.0174098392056,0.208329635111639,-1.76770467022071));
#25162=CARTESIAN_POINT('Ctrl Pts',(99.0043488632174,-0.00410467531662812,
-1.77895784161103));
#25163=CARTESIAN_POINT('Ctrl Pts',(98.9982963472337,-0.102422050787166,
-1.77601094703713));
#25164=CARTESIAN_POINT('Ctrl Pts',(98.9899907356909,-0.231164989801637,
-1.76142310901206));
#25165=CARTESIAN_POINT('Ctrl Pts',(98.9879573511447,-0.26224242541558,-1.75706497866967));
#25166=CARTESIAN_POINT('Ctrl Pts',(98.9848687432149,-0.308661201271373,
-1.74929657074224));
#25167=CARTESIAN_POINT('Ctrl Pts',(98.983832873189,-0.324100285114179,-1.74650199209836));
#25168=CARTESIAN_POINT('Ctrl Pts',(98.9819455264714,-0.351983166697774,
-1.74107255821595));
#25169=CARTESIAN_POINT('Ctrl Pts',(98.981096339101,-0.364439659402339,-1.73850784375318));
#25170=CARTESIAN_POINT('Ctrl Pts',(98.9792517110055,-0.391298986780564,
-1.73267632803631));
#25171=CARTESIAN_POINT('Ctrl Pts',(98.9782548407113,-0.405690677627047,
-1.7293632371168));
#25172=CARTESIAN_POINT('Ctrl Pts',(98.9754905083115,-0.445248864144231,
-1.71973564615285));
#25173=CARTESIAN_POINT('Ctrl Pts',(98.973711244928,-0.470320023236342,-1.7130488012569));
#25174=CARTESIAN_POINT('Ctrl Pts',(98.9627560009343,-0.62225491264947,-1.66893886346217));
#25175=CARTESIAN_POINT('Ctrl Pts',(98.9531381926924,-0.744737609617128,
-1.61799625190002));
#25176=CARTESIAN_POINT('Ctrl Pts',(98.9387751744068,-0.916557642621267,
-1.52286089100711));
#25177=CARTESIAN_POINT('Ctrl Pts',(98.9340881646006,-0.970982670593367,
-1.48875005448321));
#25178=CARTESIAN_POINT('Ctrl Pts',(98.9270063664742,-1.05193503502289,-1.4316814844162));
#25179=CARTESIAN_POINT('Ctrl Pts',(98.9245446169095,-1.07983066464143,-1.41076054225632));
#25180=CARTESIAN_POINT('Ctrl Pts',(98.9213426083941,-1.11599475049936,-1.38193679851596));
#25181=CARTESIAN_POINT('Ctrl Pts',(98.9205597403517,-1.12482691845868,-1.37475744002252));
#25182=CARTESIAN_POINT('Ctrl Pts',(98.9192712337831,-1.13935703203509,-1.36271263796874));
#25183=CARTESIAN_POINT('Ctrl Pts',(98.9187623207169,-1.14509418747203,-1.35789524235546));
#25184=CARTESIAN_POINT('Ctrl Pts',(98.9177317861651,-1.15671157779988,-1.34801431649525));
#25185=CARTESIAN_POINT('Ctrl Pts',(98.9172103550533,-1.16258940881228,-1.34294830281267));
#25186=CARTESIAN_POINT('Ctrl Pts',(98.9158466032465,-1.17795474137115,-1.32952866687338));
#25187=CARTESIAN_POINT('Ctrl Pts',(98.9150087796622,-1.18738679453287,-1.32111183162366));
#25188=CARTESIAN_POINT('Ctrl Pts',(98.9112792988069,-1.22928902317129,-1.28290842335939));
#25189=CARTESIAN_POINT('Ctrl Pts',(98.908459905395,-1.2607366513882,-1.25201809917143));
#25190=CARTESIAN_POINT('Ctrl Pts',(98.8996736473734,-1.35657216437321,-1.15060380264404));
#25191=CARTESIAN_POINT('Ctrl Pts',(98.8938787514653,-1.41644237731922,-1.07604378091271));
#25192=CARTESIAN_POINT('Ctrl Pts',(98.8825364292769,-1.51986205985886,-0.923560528793251));
#25193=CARTESIAN_POINT('Ctrl Pts',(98.8770157542252,-1.56410841159947,-0.846467393317558));
#25194=CARTESIAN_POINT('Ctrl Pts',(98.8695858986433,-1.61382738017507,-0.742513357050467));
#25195=CARTESIAN_POINT('Ctrl Pts',(98.8678626619265,-1.62471391625138,-0.718379753274194));
#25196=CARTESIAN_POINT('Ctrl Pts',(98.86515232877,-1.64081042075584,-0.680457262471034));
#25197=CARTESIAN_POINT('Ctrl Pts',(98.8641779750259,-1.64639525545746,-0.666830985903728));
#25198=CARTESIAN_POINT('Ctrl Pts',(98.8623512376158,-1.65648721988568,-0.641308006905735));
#25199=CARTESIAN_POINT('Ctrl Pts',(98.8615003672752,-1.66103724594756,-0.62942920365116));
#25200=CARTESIAN_POINT('Ctrl Pts',(98.8595867745885,-1.67093199307132,-0.602742203805938));
#25201=CARTESIAN_POINT('Ctrl Pts',(98.8585218429632,-1.6762081584955,-0.587909917617987));
#25202=CARTESIAN_POINT('Ctrl Pts',(98.8557712079912,-1.68924429291163,-0.549660184306032));
#25203=CARTESIAN_POINT('Ctrl Pts',(98.8540762122415,-1.69671459747118,-0.526148332548572));
#25204=CARTESIAN_POINT('Ctrl Pts',(98.8448155523712,-1.7344946103781,-0.398055064325833));
#25205=CARTESIAN_POINT('Ctrl Pts',(98.8369629025161,-1.75562411564626,-0.291026234724324));
#25206=CARTESIAN_POINT('Ctrl Pts',(98.8231721092441,-1.77504843875658,-0.103236649659238));
#25207=CARTESIAN_POINT('Ctrl Pts',(98.8173006873,-1.77789622299953,-0.0232520401958028));
#25208=CARTESIAN_POINT('Ctrl Pts',(98.8096424742066,-1.77449283939336,0.0833974388469762));
#25209=CARTESIAN_POINT('Ctrl Pts',(98.8077385175066,-1.77303522794508,0.110119037685076));
#25210=CARTESIAN_POINT('Ctrl Pts',(98.804506493651,-1.7694922730804,0.155985521807472));
#25211=CARTESIAN_POINT('Ctrl Pts',(98.8031670754739,-1.76769841838572,0.17514783552763));
#25212=CARTESIAN_POINT('Ctrl Pts',(98.8012166407239,-1.7645971226372,0.203332308239764));
#25213=CARTESIAN_POINT('Ctrl Pts',(98.8005935828458,-1.76353118416357,0.212378917090293));
#25214=CARTESIAN_POINT('Ctrl Pts',(98.7994866983602,-1.76150141464823,0.228535103057142));
#25215=CARTESIAN_POINT('Ctrl Pts',(98.7990014777767,-1.76056405615017,0.235647483427507));
#25216=CARTESIAN_POINT('Ctrl Pts',(98.7979180495305,-1.75836380205932,0.251595827902148));
#25217=CARTESIAN_POINT('Ctrl Pts',(98.7973211495345,-1.75707737481331,0.260428163777265));
#25218=CARTESIAN_POINT('Ctrl Pts',(98.7955128630197,-1.75295480552192,0.287310531903416));
#25219=CARTESIAN_POINT('Ctrl Pts',(98.7943125660607,-1.74990659700875,0.305327459531161));
#25220=CARTESIAN_POINT('Ctrl Pts',(98.7874779139404,-1.73077690356379,0.408674420337282));
#25221=CARTESIAN_POINT('Ctrl Pts',(98.7821099263512,-1.70873179509717,0.492790724815104));
#25222=CARTESIAN_POINT('Ctrl Pts',(98.7716504320384,-1.65365588455882,0.653777184477575));
#25223=CARTESIAN_POINT('Ctrl Pts',(98.7665682559406,-1.62118309839323,0.730593686956729));
#25224=CARTESIAN_POINT('Ctrl Pts',(98.7587953743425,-1.56484439991561,0.841433679805118));
#25225=CARTESIAN_POINT('Ctrl Pts',(98.7562027206278,-1.54498544507029,0.877364388479768));
#25226=CARTESIAN_POINT('Ctrl Pts',(98.7515861669163,-1.50800319683622,0.939120824538004));
#25227=CARTESIAN_POINT('Ctrl Pts',(98.7495801744132,-1.4914153587427,0.96524691523214));
#25228=CARTESIAN_POINT('Ctrl Pts',(98.7465248642275,-1.46544750786853,1.00387810556305));
#25229=CARTESIAN_POINT('Ctrl Pts',(98.7454942651578,-1.4565705097325,1.0167152862802));
#25230=CARTESIAN_POINT('Ctrl Pts',(98.7436124682416,-1.4401579709312,1.0397935837147));
#25231=CARTESIAN_POINT('Ctrl Pts',(98.7427634949703,-1.43267936766312,1.05007404166609));
#25232=CARTESIAN_POINT('Ctrl Pts',(98.7409146461137,-1.4162376790882,1.07217297615569));
#25233=CARTESIAN_POINT('Ctrl Pts',(98.7399132876168,-1.40723567697853,1.0839611527235));
#25234=CARTESIAN_POINT('Ctrl Pts',(98.7371236904087,-1.38189798586762,1.11629336927533));
#25235=CARTESIAN_POINT('Ctrl Pts',(98.7353232936643,-1.36525354271101,1.13658944457184));
#25236=CARTESIAN_POINT('Ctrl Pts',(98.7245622101405,-1.26410964732252,1.25449502180644));
#25237=CARTESIAN_POINT('Ctrl Pts',(98.7151838822325,-1.16963485109714,1.34300929100709));
#25238=CARTESIAN_POINT('Ctrl Pts',(98.7009129047559,-1.01358937622943,1.46015954330516));
#25239=CARTESIAN_POINT('Ctrl Pts',(98.696084047736,-0.95857742238463,1.49684986835111));
#25240=CARTESIAN_POINT('Ctrl Pts',(98.6888200224892,-0.871091029044569,
1.54839342678187));
#25241=CARTESIAN_POINT('Ctrl Pts',(98.6863143274156,-0.840000626976328,
1.56547792405233));
#25242=CARTESIAN_POINT('Ctrl Pts',(98.6830651927527,-0.798223280701308,
1.58683166103935));
#25243=CARTESIAN_POINT('Ctrl Pts',(98.6822776109989,-0.787978915687187,
1.59194358323487));
#25244=CARTESIAN_POINT('Ctrl Pts',(98.680983494902,-0.770938531780708,1.60024190665419));
#25245=CARTESIAN_POINT('Ctrl Pts',(98.6804736289704,-0.764170595658663,
1.60348485725573));
#25246=CARTESIAN_POINT('Ctrl Pts',(98.6795072361373,-0.751235177516634,
1.60958253944513));
#25247=CARTESIAN_POINT('Ctrl Pts',(98.6790502187828,-0.745071556700032,
1.61244492078025));
#25248=CARTESIAN_POINT('Ctrl Pts',(98.6778166922189,-0.728314711739129,
1.62011018794636));
#25249=CARTESIAN_POINT('Ctrl Pts',(98.6770442375694,-0.717690275736269,
1.62484461611598));
#25250=CARTESIAN_POINT('Ctrl Pts',(98.674027012129,-0.675712106864466,1.64305870571012));
#25251=CARTESIAN_POINT('Ctrl Pts',(98.6718247187761,-0.644017051319341,
1.65573885405461));
#25252=CARTESIAN_POINT('Ctrl Pts',(98.6631162420858,-0.515445484201801,
1.70292476970301));
#25253=CARTESIAN_POINT('Ctrl Pts',(98.6568762560695,-0.416015601717569,
1.72990498191401));
#25254=CARTESIAN_POINT('Ctrl Pts',(98.6448591896422,-0.223712728737859,
1.76453484334769));
#25255=CARTESIAN_POINT('Ctrl Pts',(98.6391163310975,-0.131489548701381,
1.77379208137029));
#25256=CARTESIAN_POINT('Ctrl Pts',(98.6314158825446,-0.0120159714731658,
1.77641397412405));
#25257=CARTESIAN_POINT('Ctrl Pts',(98.6296616920669,0.0149478827089522,
1.77639168728451));
#25258=CARTESIAN_POINT('Ctrl Pts',(98.6269134675092,0.056721081769153,1.77540603183595));
#25259=CARTESIAN_POINT('Ctrl Pts',(98.625932778585,0.0715371409881411,1.77487077672411));
#25260=CARTESIAN_POINT('Ctrl Pts',(98.6241002612597,0.0990427900830045,
1.7735321309148));
#25261=CARTESIAN_POINT('Ctrl Pts',(98.6232500284524,0.111733889720835,1.77277782506423));
#25262=CARTESIAN_POINT('Ctrl Pts',(98.6213458058649,0.139993132443401,1.77079356329233));
#25263=CARTESIAN_POINT('Ctrl Pts',(98.620289706387,0.155555192378052,1.76949441249334));
#25264=CARTESIAN_POINT('Ctrl Pts',(98.6171858477343,0.200956353272661,1.76510070444062));
#25265=CARTESIAN_POINT('Ctrl Pts',(98.6151211068252,0.230735346222123,1.76145535350444));
#25266=CARTESIAN_POINT('Ctrl Pts',(98.6033794876242,0.397640475646846,1.73671903822601));
#25267=CARTESIAN_POINT('Ctrl Pts',(98.593227490331,0.531999176174459,1.70037494881006));
#25268=CARTESIAN_POINT('Ctrl Pts',(98.5790893099674,0.711680908388488,1.62836936601019));
#25269=CARTESIAN_POINT('Ctrl Pts',(98.5750987581099,0.761657481554427,1.60560116400373));
#25270=CARTESIAN_POINT('Ctrl Pts',(98.568928291336,0.8386733296598,1.56610773033495));
#25271=CARTESIAN_POINT('Ctrl Pts',(98.5666981463312,0.866455525316215,1.5509098923693));
#25272=CARTESIAN_POINT('Ctrl Pts',(98.5637466923177,0.903327222458187,1.52943946103634));
#25273=CARTESIAN_POINT('Ctrl Pts',(98.5629904284223,0.912784591470168,1.52381410971773));
#25274=CARTESIAN_POINT('Ctrl Pts',(98.5617335720251,0.928527920055514,1.51425062890651));
#25275=CARTESIAN_POINT('Ctrl Pts',(98.5612300216202,0.934842494583412,1.51036041516676));
#25276=CARTESIAN_POINT('Ctrl Pts',(98.560197442476,0.947809300271062,1.50225948730427));
#25277=CARTESIAN_POINT('Ctrl Pts',(98.5596687334252,0.954458194486666,1.49804392389004));
#25278=CARTESIAN_POINT('Ctrl Pts',(98.5582635418187,0.972147243862521,1.48666304702944));
#25279=CARTESIAN_POINT('Ctrl Pts',(98.5573920627569,0.983136403498689,1.47941884425101));
#25280=CARTESIAN_POINT('Ctrl Pts',(98.5532051093773,1.03595757479437,1.44374988768768));
#25281=CARTESIAN_POINT('Ctrl Pts',(98.5499855428606,1.07664705352534,1.41366684949636));
#25282=CARTESIAN_POINT('Ctrl Pts',(98.5365686148749,1.24329277849515,1.2790849515194));
#25283=CARTESIAN_POINT('Ctrl Pts',(98.5268456739964,1.35576864060012,1.15919373416175));
#25284=CARTESIAN_POINT('Ctrl Pts',(98.5141753303012,1.47030673723865,0.997230721897223));
#25285=CARTESIAN_POINT('Ctrl Pts',(98.5119301891267,1.48952844472357,0.968284963338501));
#25286=CARTESIAN_POINT('Ctrl Pts',(98.5085854473844,1.51650398303549,0.924957011884526));
#25287=CARTESIAN_POINT('Ctrl Pts',(98.5075104643707,1.52492864688005,0.911000766669012));
#25288=CARTESIAN_POINT('Ctrl Pts',(98.5055810222647,1.53960661139219,0.885911136446451));
#25289=CARTESIAN_POINT('Ctrl Pts',(98.5047293358463,1.54593427384532,0.874822419612228));
#25290=CARTESIAN_POINT('Ctrl Pts',(98.5029110386238,1.55911957693626,0.851126404757805));
#25291=CARTESIAN_POINT('Ctrl Pts',(98.5019433509962,1.56594502415916,0.838502338871315));
#25292=CARTESIAN_POINT('Ctrl Pts',(98.499298271279,1.58407846727482,0.803969706712192));
#25293=CARTESIAN_POINT('Ctrl Pts',(98.49761044578,1.59508413231313,0.781906889647084));
#25294=CARTESIAN_POINT('Ctrl Pts',(98.4858863631611,1.66764272314306,0.628538722057488));
#25295=CARTESIAN_POINT('Ctrl Pts',(98.4753015316341,1.7133620134927,0.490375265286924));
#25296=CARTESIAN_POINT('Ctrl Pts',(98.4590902808865,1.75685440464913,0.272833814031389));
#25297=CARTESIAN_POINT('Ctrl Pts',(98.4535002958183,1.76701811105037,0.196532193408574));
#25298=CARTESIAN_POINT('Ctrl Pts',(98.4468199706563,1.77344041694632,0.101531418005063));
#25299=CARTESIAN_POINT('Ctrl Pts',(98.4455465498248,1.77439314168554,0.0832381253092255));
#25300=CARTESIAN_POINT('Ctrl Pts',(98.4436731452741,1.77538935398147,0.0560046241025156));
#25301=CARTESIAN_POINT('Ctrl Pts',(98.4430623886061,1.77564858790227,0.0470741658988919));
#25302=CARTESIAN_POINT('Ctrl Pts',(98.4420162058808,1.77597921489377,0.0316805725871297));
#25303=CARTESIAN_POINT('Ctrl Pts',(98.4415790622106,1.77608272802193,0.0252185935006792));
#25304=CARTESIAN_POINT('Ctrl Pts',(98.440555870741,1.77624318808995,0.0100232632241994));
#25305=CARTESIAN_POINT('Ctrl Pts',(98.4399714354593,1.77627100220953,0.00128988648284571));
#25306=CARTESIAN_POINT('Ctrl Pts',(98.4385008173595,1.7761783837321,-0.0208113540785626));
#25307=CARTESIAN_POINT('Ctrl Pts',(98.4376191380422,1.77597145713807,-0.0341784484187622));
#25308=CARTESIAN_POINT('Ctrl Pts',(98.4367443001643,1.77561363837182,-0.0475422940967033));
#25309=CARTESIAN_POINT('',(98.4811171438985,0.00162347919700848,1.77624925807593));
#25310=CARTESIAN_POINT('Ctrl Pts',(98.289313862947,1.77561363837197,-0.0475422940912524));
#25311=CARTESIAN_POINT('Ctrl Pts',(98.2926748518192,1.77687955123043,-0.000262873115973129));
#25312=CARTESIAN_POINT('Ctrl Pts',(98.2960828732913,1.77625693264144,0.0470604327664538));
#25313=CARTESIAN_POINT('Ctrl Pts',(98.3092516879989,1.76662997259377,0.228110696891337));
#25314=CARTESIAN_POINT('Ctrl Pts',(98.3192027038273,1.74440043006838,0.360673984676432));
#25315=CARTESIAN_POINT('Ctrl Pts',(98.3298177239441,1.70265328893669,0.506302355255301));
#25316=CARTESIAN_POINT('Ctrl Pts',(98.3310331350711,1.69758237990944,0.52305297849011));
#25317=CARTESIAN_POINT('Ctrl Pts',(98.332834906219,1.68961372689328,0.548037973578791));
#25318=CARTESIAN_POINT('Ctrl Pts',(98.3334310134548,1.68690168186181,0.556329839586212));
#25319=CARTESIAN_POINT('Ctrl Pts',(98.3344578002709,1.68209655016203,0.570662883572255));
#25320=CARTESIAN_POINT('Ctrl Pts',(98.3348900687355,1.68003183489243,0.576713072352935));
#25321=CARTESIAN_POINT('Ctrl Pts',(98.335909235951,1.67506457256116,0.591015444484796));
#25322=CARTESIAN_POINT('Ctrl Pts',(98.3364944684919,1.67213367977719,0.599257492989124));
#25323=CARTESIAN_POINT('Ctrl Pts',(98.33824851222,1.66311583413547,0.62403546039924));
#25324=CARTESIAN_POINT('Ctrl Pts',(98.3394070841259,1.65684340338447,0.640503339522243));
#25325=CARTESIAN_POINT('Ctrl Pts',(98.3451772684421,1.62406675285224,0.722850979244298));
#25326=CARTESIAN_POINT('Ctrl Pts',(98.3496120734622,1.59387121686358,0.787199528455292));
#25327=CARTESIAN_POINT('Ctrl Pts',(98.3619943555025,1.49795900545056,0.963303832718304));
#25328=CARTESIAN_POINT('Ctrl Pts',(98.3698167081504,1.42377010853301,1.06991244510049));
#25329=CARTESIAN_POINT('Ctrl Pts',(98.3804699594886,1.31370190167222,1.19611550347375));
#25330=CARTESIAN_POINT('Ctrl Pts',(98.3829148951586,1.28784252760183,1.22391432785782));
#25331=CARTESIAN_POINT('Ctrl Pts',(98.3864111018609,1.25019429420161,1.26187112190757));
#25332=CARTESIAN_POINT('Ctrl Pts',(98.3874311661815,1.23913127248095,1.2727364872564));
#25333=CARTESIAN_POINT('Ctrl Pts',(98.3893084125561,1.21863990764363,1.29234130997582));
#25334=CARTESIAN_POINT('Ctrl Pts',(98.3901635611303,1.20925614744861,1.30112598967335));
#25335=CARTESIAN_POINT('Ctrl Pts',(98.3919116788421,1.18997983046023,1.3187830089058));
#25336=CARTESIAN_POINT('Ctrl Pts',(98.3928048933193,1.18008142031832,1.32764771163769));
#25337=CARTESIAN_POINT('Ctrl Pts',(98.3937500890546,1.16955835449965,1.33686117729683));
#25338=CARTESIAN_POINT('Ctrl Pts',(98.3937973804396,1.16903172191039,1.33732172086906));
#25339=CARTESIAN_POINT('Ctrl Pts',(98.3938910820493,1.16798801740504,1.33823335952641));
#25340=CARTESIAN_POINT('Ctrl Pts',(98.3939374917743,1.1674709558828,1.33868446637692));
#25341=CARTESIAN_POINT('Ctrl Pts',(98.3940299924789,1.16644014107159,1.33958274238679));
#25342=CARTESIAN_POINT('Ctrl Pts',(98.3940760832672,1.16592639171338,1.34002991590023));
#25343=CARTESIAN_POINT('Ctrl Pts',(98.3955449320196,1.14955010418151,1.35426748302609));
#25344=CARTESIAN_POINT('Ctrl Pts',(98.396979267043,1.13344491347429,1.36777498861236));
#25345=CARTESIAN_POINT('Ctrl Pts',(98.4035806832206,1.058837064672,1.42812631167305));
#25346=CARTESIAN_POINT('Ctrl Pts',(98.4088804281883,0.99765300898167,1.47151843145206));
#25347=CARTESIAN_POINT('Ctrl Pts',(98.4214706820547,0.849054705011137,1.56336936999886));
#25348=CARTESIAN_POINT('Ctrl Pts',(98.4288226220731,0.759923363159647,1.60858088611291));
#25349=CARTESIAN_POINT('Ctrl Pts',(98.440494697446,0.611053310709455,1.66894721811466));
#25350=CARTESIAN_POINT('Ctrl Pts',(98.4448690506855,0.553485999450752,1.68891259510949));
#25351=CARTESIAN_POINT('Ctrl Pts',(98.4500574456642,0.48188554245696,1.70968912342778));
#25352=CARTESIAN_POINT('Ctrl Pts',(98.4510007887297,0.468725649094946,1.7133437685902));
#25353=CARTESIAN_POINT('Ctrl Pts',(98.4524789907407,0.447859275483054,1.71888016523592));
#25354=CARTESIAN_POINT('Ctrl Pts',(98.4530192363543,0.440180410349877,1.72086262253008));
#25355=CARTESIAN_POINT('Ctrl Pts',(98.4540488943388,0.425438818715921,1.72456333650106));
#25356=CARTESIAN_POINT('Ctrl Pts',(98.4545387242794,0.418378496097635,1.72628975722882));
#25357=CARTESIAN_POINT('Ctrl Pts',(98.4557293251382,0.40110642187058,1.73040101197066));
#25358=CARTESIAN_POINT('Ctrl Pts',(98.4564274755549,0.390883568340982,1.73273889357978));
#25359=CARTESIAN_POINT('Ctrl Pts',(98.457923829001,0.368784289121395,1.73758727588388));
#25360=CARTESIAN_POINT('Ctrl Pts',(98.4587204364205,0.356901554587099,1.7400668642479));
#25361=CARTESIAN_POINT('Ctrl Pts',(98.4670245891664,0.231918324213672,1.76481310706288));
#25362=CARTESIAN_POINT('Ctrl Pts',(98.4740375076626,0.116925795384379,1.77614387257846));
#25363=CARTESIAN_POINT('Ctrl Pts',(98.4811171438985,0.00162347919702141,
1.77624925807593));
#25364=CARTESIAN_POINT('Ctrl Pts',(98.4811171438985,0.00162347919766435,
1.77624925807593));
#25365=CARTESIAN_POINT('Ctrl Pts',(98.4875839157544,-0.103697436792226,
1.77634552064461));
#25366=CARTESIAN_POINT('Ctrl Pts',(98.494081006342,-0.208796193401722,1.76707590037909));
#25367=CARTESIAN_POINT('Ctrl Pts',(98.5020981984134,-0.331206729051687,
1.74520167397757));
#25368=CARTESIAN_POINT('Ctrl Pts',(98.5033345465983,-0.349899210184728,
1.74155025172625));
#25369=CARTESIAN_POINT('Ctrl Pts',(98.5054576915823,-0.381654194789689,
1.73481531090901));
#25370=CARTESIAN_POINT('Ctrl Pts',(98.5063397633945,-0.394747301001014,
1.73188297511));
#25371=CARTESIAN_POINT('Ctrl Pts',(98.5081044220591,-0.420732992364379,
1.72575323467924));
#25372=CARTESIAN_POINT('Ctrl Pts',(98.508986857412,-0.43362542444743,1.72255898384962));
#25373=CARTESIAN_POINT('Ctrl Pts',(98.5107328039029,-0.458925592904638,
1.71598854539845));
#25374=CARTESIAN_POINT('Ctrl Pts',(98.5115959674733,-0.471334902767029,
1.71262161089462));
#25375=CARTESIAN_POINT('Ctrl Pts',(98.513706922513,-0.501436778407503,1.7041023356231));
#25376=CARTESIAN_POINT('Ctrl Pts',(98.5149592350811,-0.519087499813065,
1.69880891680824));
#25377=CARTESIAN_POINT('Ctrl Pts',(98.5193533491707,-0.580281886891746,
1.67941411298376));
#25378=CARTESIAN_POINT('Ctrl Pts',(98.5225402361988,-0.623357159398503,
1.66390625594159));
#25379=CARTESIAN_POINT('Ctrl Pts',(98.5331483485892,-0.762482084685145,
1.60765805585683));
#25380=CARTESIAN_POINT('Ctrl Pts',(98.5407652104414,-0.855540222574703,
1.56012487059466));
#25381=CARTESIAN_POINT('Ctrl Pts',(98.5529661464366,-0.996886164596863,
1.47146092481033));
#25382=CARTESIAN_POINT('Ctrl Pts',(98.5575322656208,-1.04810136681483,1.43543152092562));
#25383=CARTESIAN_POINT('Ctrl Pts',(98.5644393845948,-1.12410865233419,1.37571986674328));
#25384=CARTESIAN_POINT('Ctrl Pts',(98.5668449705458,-1.15029743806007,1.3538986580067));
#25385=CARTESIAN_POINT('Ctrl Pts',(98.5699898124653,-1.18434131904986,1.32383089194837));
#25386=CARTESIAN_POINT('Ctrl Pts',(98.570769630895,-1.19276688433482,1.31624456962711));
#25387=CARTESIAN_POINT('Ctrl Pts',(98.5720510214666,-1.20659376044404,1.30355313468374));
#25388=CARTESIAN_POINT('Ctrl Pts',(98.5725558631913,-1.2120365933746,1.29849396643398));
#25389=CARTESIAN_POINT('Ctrl Pts',(98.5735753785123,-1.22302183098433,1.28815381981295));
#25390=CARTESIAN_POINT('Ctrl Pts',(98.5740898933287,-1.22856212945266,1.28287090629999));
#25391=CARTESIAN_POINT('Ctrl Pts',(98.5754300682774,-1.24297766284799,1.26894603370402));
#25392=CARTESIAN_POINT('Ctrl Pts',(98.576251438368,-1.25179713435195,1.2602465880456));
#25393=CARTESIAN_POINT('Ctrl Pts',(98.5798302854721,-1.29011325097555,1.22165277626801));
#25394=CARTESIAN_POINT('Ctrl Pts',(98.5825222048819,-1.31863773503365,1.1908076446268));
#25395=CARTESIAN_POINT('Ctrl Pts',(98.591290013983,-1.40931625978545,1.08549301844199));
#25396=CARTESIAN_POINT('Ctrl Pts',(98.5971759493595,-1.46646821425704,1.00694623045769));
#25397=CARTESIAN_POINT('Ctrl Pts',(98.6086676286214,-1.56360968666951,0.847490809877018));
#25398=CARTESIAN_POINT('Ctrl Pts',(98.614245295967,-1.60441542964787,0.7674401857532));
#25399=CARTESIAN_POINT('Ctrl Pts',(98.6217380132887,-1.64920890843683,0.660209009121993));
#25400=CARTESIAN_POINT('Ctrl Pts',(98.6234625044879,-1.65887208667197,0.635538543580224));
#25401=CARTESIAN_POINT('Ctrl Pts',(98.6261684087063,-1.67301255676996,0.596914874832605));
#25402=CARTESIAN_POINT('Ctrl Pts',(98.6271369871057,-1.67787529767851,0.58310620540181));
#25403=CARTESIAN_POINT('Ctrl Pts',(98.6289489764837,-1.68660068306509,0.557315573032014));
#25404=CARTESIAN_POINT('Ctrl Pts',(98.6297908543013,-1.69050773137571,0.545349528412544));
#25405=CARTESIAN_POINT('Ctrl Pts',(98.6316788155087,-1.69894108765747,0.518559036508505));
#25406=CARTESIAN_POINT('Ctrl Pts',(98.6327269984785,-1.70340115010637,0.503714987754341));
#25407=CARTESIAN_POINT('Ctrl Pts',(98.6358142009334,-1.71588728261929,0.460094900941571));
#25408=CARTESIAN_POINT('Ctrl Pts',(98.6378701064034,-1.72338199963596,0.431173723486116));
#25409=CARTESIAN_POINT('Ctrl Pts',(98.6496118578181,-1.76158244788667,0.266797333653768));
#25410=CARTESIAN_POINT('Ctrl Pts',(98.6597745737697,-1.77704130590816,0.128315204723318));
#25411=CARTESIAN_POINT('Ctrl Pts',(98.6753244703899,-1.77578011922774,-0.0845794326828024));
#25412=CARTESIAN_POINT('Ctrl Pts',(98.6807007819412,-1.77071019573902,-0.158544002731478));
#25413=CARTESIAN_POINT('Ctrl Pts',(98.6871531795143,-1.75869201340312,-0.249777149980269));
#25414=CARTESIAN_POINT('Ctrl Pts',(98.6884004977045,-1.75607815253738,-0.26753655208544));
#25415=CARTESIAN_POINT('Ctrl Pts',(98.6902397272791,-1.75178042620321,-0.293950734562597));
#25416=CARTESIAN_POINT('Ctrl Pts',(98.6908419663048,-1.75030071227005,-0.302636945739618));
#25417=CARTESIAN_POINT('Ctrl Pts',(98.6918751046767,-1.74763548509284,-0.317608526650054));
#25418=CARTESIAN_POINT('Ctrl Pts',(98.6923076625196,-1.74648059900108,-0.323898882195918));
#25419=CARTESIAN_POINT('Ctrl Pts',(98.6933215921682,-1.74368131157944,-0.338695435045995));
#25420=CARTESIAN_POINT('Ctrl Pts',(98.6939013673405,-1.74200862743133,-0.347196002126398));
#25421=CARTESIAN_POINT('Ctrl Pts',(98.6956218738606,-1.7368312694828,-0.372527517922934));
#25422=CARTESIAN_POINT('Ctrl Pts',(98.6967529342113,-1.73314426243373,-0.389320728585039));
#25423=CARTESIAN_POINT('Ctrl Pts',(98.7067051547055,-1.69822512922198,-0.5380250326482));
#25424=CARTESIAN_POINT('Ctrl Pts',(98.714852794876,-1.65222733382778,-0.666029239217347));
#25425=CARTESIAN_POINT('Ctrl Pts',(98.7284898044332,-1.55410184525391,-0.864394764854116));
#25426=CARTESIAN_POINT('Ctrl Pts',(98.7338305891552,-1.51059069657303,-0.938362507798115));
#25427=CARTESIAN_POINT('Ctrl Pts',(98.7410347656329,-1.44716871950847,-1.03026244745366));
#25428=CARTESIAN_POINT('Ctrl Pts',(98.7427254591458,-1.43195733628363,-1.05130209171884));
#25429=CARTESIAN_POINT('Ctrl Pts',(98.7453899781658,-1.40752132847668,-1.08358613757846));
#25430=CARTESIAN_POINT('Ctrl Pts',(98.7463516137895,-1.39861008326424,-1.09506393491514));
#25431=CARTESIAN_POINT('Ctrl Pts',(98.7481573354621,-1.38171301983853,-1.11628484631996));
#25432=CARTESIAN_POINT('Ctrl Pts',(98.7489999779953,-1.373762382497,-1.12605489636957));
#25433=CARTESIAN_POINT('Ctrl Pts',(98.7508985234889,-1.35570729167018,-1.14776585877698));
#25434=CARTESIAN_POINT('Ctrl Pts',(98.7519566367536,-1.34554777082187,-1.15965938807568));
#25435=CARTESIAN_POINT('Ctrl Pts',(98.7546959680289,-1.31900612804613,-1.1899127268983));
#25436=CARTESIAN_POINT('Ctrl Pts',(98.7563864816377,-1.30239766536331,-1.20806857392049));
#25437=CARTESIAN_POINT('Ctrl Pts',(98.7654135191758,-1.21254712717535,-1.3022834953871));
#25438=CARTESIAN_POINT('Ctrl Pts',(98.7730184037613,-1.1330195401061,-1.37203244763905));
#25439=CARTESIAN_POINT('Ctrl Pts',(98.7867598095984,-0.981038595867624,
-1.48305753577234));
#25440=CARTESIAN_POINT('Ctrl Pts',(98.7928353713481,-0.910969693365428,
-1.52709902369894));
#25441=CARTESIAN_POINT('Ctrl Pts',(98.8007216822298,-0.814129666660991,
-1.57892217976014));
#25442=CARTESIAN_POINT('Ctrl Pts',(98.8026559734616,-0.789880305491776,
-1.59119188820044));
#25443=CARTESIAN_POINT('Ctrl Pts',(98.8059310273371,-0.747825033144203,
-1.61127255952482));
#25444=CARTESIAN_POINT('Ctrl Pts',(98.8072835985089,-0.730155243086849,
-1.61935633492277));
#25445=CARTESIAN_POINT('Ctrl Pts',(98.8092456467165,-0.704028887914428,
-1.63079428755314));
#25446=CARTESIAN_POINT('Ctrl Pts',(98.8098674678683,-0.695674192761286,
-1.6343757554316));
#25447=CARTESIAN_POINT('Ctrl Pts',(98.8109683782373,-0.680742530658057,
-1.64064137468307));
#25448=CARTESIAN_POINT('Ctrl Pts',(98.8114488954001,-0.674176531846912,
-1.64335039554523));
#25449=CARTESIAN_POINT('Ctrl Pts',(98.812516464792,-0.659479487156446,-1.64931123397924));
#25450=CARTESIAN_POINT('Ctrl Pts',(98.8131023006504,-0.651340458944043,
-1.65254239133418));
#25451=CARTESIAN_POINT('Ctrl Pts',(98.8148600603908,-0.626708875417907,
-1.66211076528193));
#25452=CARTESIAN_POINT('Ctrl Pts',(98.8160216812129,-0.610144793441377,
-1.66826244930331));
#25453=CARTESIAN_POINT('Ctrl Pts',(98.8238253475529,-0.497158532421888,
-1.70831601058425));
#25454=CARTESIAN_POINT('Ctrl Pts',(98.8300896204472,-0.398045422492196,
-1.73409210342019));
#25455=CARTESIAN_POINT('Ctrl Pts',(98.8414800174878,-0.215095904723764,
-1.76514654681028));
#25456=CARTESIAN_POINT('Ctrl Pts',(98.8465879756094,-0.13206097766988,-1.7732927947059));
#25457=CARTESIAN_POINT('Ctrl Pts',(98.8549759869495,0.000984312464261099,
-1.77694682007739));
#25458=CARTESIAN_POINT('Ctrl Pts',(98.8581585024249,0.0507655887931716,
-1.77622158975453));
#25459=CARTESIAN_POINT('Ctrl Pts',(98.86260976139,0.118880795877582,-1.77236347644932));
#25460=CARTESIAN_POINT('Ctrl Pts',(98.863822793402,0.137296022137774,-1.77103209920204));
#25461=CARTESIAN_POINT('Ctrl Pts',(98.8659048649879,0.168630359430165,-1.76827506414069));
#25462=CARTESIAN_POINT('Ctrl Pts',(98.8667693107381,0.181560933057691,-1.76699420283598));
#25463=CARTESIAN_POINT('Ctrl Pts',(98.8684237835398,0.206151542872894,-1.76428557099717));
#25464=CARTESIAN_POINT('Ctrl Pts',(98.8692129476589,0.217813788089008,-1.76288376725664));
#25465=CARTESIAN_POINT('Ctrl Pts',(98.871070182808,0.245097660709174,-1.75932937590262));
#25466=CARTESIAN_POINT('Ctrl Pts',(98.8721411209248,0.260706010851268,-1.75708425070233));
#25467=CARTESIAN_POINT('Ctrl Pts',(98.8759247362313,0.315401275171302,-1.74847200709364));
#25468=CARTESIAN_POINT('Ctrl Pts',(98.8786714290312,0.354300724598346,-1.74100628688364));
#25469=CARTESIAN_POINT('Ctrl Pts',(98.8904415437691,0.517555674101067,-1.70397611009358));
#25470=CARTESIAN_POINT('Ctrl Pts',(98.8998194007648,0.638766261996261,-1.66233793867587));
#25471=CARTESIAN_POINT('Ctrl Pts',(98.9142854474111,0.818207159846212,-1.57815155134061));
#25472=CARTESIAN_POINT('Ctrl Pts',(98.9193890960477,0.880144384773158,-1.54446529280055));
#25473=CARTESIAN_POINT('Ctrl Pts',(98.925556167253,0.954819678083148,-1.49789575488501));
#25474=CARTESIAN_POINT('Ctrl Pts',(98.9267756550597,0.96957930582316,-1.48838447251716));
#25475=CARTESIAN_POINT('Ctrl Pts',(98.9285822191231,0.991467682733885,-1.4738155233181));
#25476=CARTESIAN_POINT('Ctrl Pts',(98.929179115918,0.998703604855317,-1.46892187690465));
#25477=CARTESIAN_POINT('Ctrl Pts',(98.9302066664914,1.01117187945313,-1.46035487301818));
#25478=CARTESIAN_POINT('Ctrl Pts',(98.9306389185864,1.01642079469667,-1.45670645512857));
#25479=CARTESIAN_POINT('Ctrl Pts',(98.9316573092023,1.02879629237097,-1.44800502914916));
#25480=CARTESIAN_POINT('Ctrl Pts',(98.9322417906084,1.03590543215427,-1.44292769026064));
#25481=CARTESIAN_POINT('Ctrl Pts',(98.9339912151489,1.05719199545506,-1.42748644154262));
#25482=CARTESIAN_POINT('Ctrl Pts',(98.935145997999,1.07125394101419,-1.41696418693468));
#25483=CARTESIAN_POINT('Ctrl Pts',(98.9431672054606,1.1687850805004,-1.34170170256927));
#25484=CARTESIAN_POINT('Ctrl Pts',(98.9496286742871,1.24650015604602,-1.26982881640559));
#25485=CARTESIAN_POINT('Ctrl Pts',(98.9626802312856,1.38913449633555,-1.11212164058899));
#25486=CARTESIAN_POINT('Ctrl Pts',(98.9692496444194,1.45357344753965,-1.02646497876475));
#25487=CARTESIAN_POINT('Ctrl Pts',(98.9780866352389,1.52613272069163,-0.909357692274584));
#25488=CARTESIAN_POINT('Ctrl Pts',(98.9800833948425,1.54166862908891,-0.882762793228912));
#25489=CARTESIAN_POINT('Ctrl Pts',(98.9831213869077,1.56396580518879,-0.842208315683904));
#25490=CARTESIAN_POINT('Ctrl Pts',(98.9841440394403,1.57124893003603,-0.828541285207962));
#25491=CARTESIAN_POINT('Ctrl Pts',(98.9860094158675,1.58412594206036,-0.803596597524649));
#25492=CARTESIAN_POINT('Ctrl Pts',(98.9868499322321,1.58978046990137,-0.792351270174113));
#25493=CARTESIAN_POINT('Ctrl Pts',(98.9886778991063,1.6017566690981,-0.76788948001522));
#25494=CARTESIAN_POINT('Ctrl Pts',(98.9896667765806,1.60803525477435,-0.754653084190841));
#25495=CARTESIAN_POINT('Ctrl Pts',(98.992413899012,1.62492265813026,-0.717883508951439));
#25496=CARTESIAN_POINT('Ctrl Pts',(98.9941838603736,1.63518294028412,-0.694195222592844));
#25497=CARTESIAN_POINT('Ctrl Pts',(99.0051623376704,1.69502118552491,-0.547349992656807));
#25498=CARTESIAN_POINT('Ctrl Pts',(99.0148168437555,1.7311698234477,-0.41919876280801));
#25499=CARTESIAN_POINT('Ctrl Pts',(99.0292100396768,1.76310811693019,-0.224994899731161));
#25500=CARTESIAN_POINT('Ctrl Pts',(99.0338908562335,1.77007927957483,-0.161223912246889));
#25501=CARTESIAN_POINT('Ctrl Pts',(99.0396587094954,1.77449477108834,-0.0806659106480894));
#25502=CARTESIAN_POINT('Ctrl Pts',(99.0408364707886,1.77517010346589,-0.0641074739969688));
#25503=CARTESIAN_POINT('Ctrl Pts',(99.0420054636133,1.77561363841465,-0.0475422924970873));
#25504=CARTESIAN_POINT('Origin',(88.3562164250559,0.,0.));
#25505=CARTESIAN_POINT('',(99.938371422543,1.77561385491717,-0.0475342058543041));
#25506=CARTESIAN_POINT('',(99.7906385404719,1.77561363837197,-0.0475422940912401));
#25507=CARTESIAN_POINT('',(88.3562164250559,1.77561363837197,-0.0475422940912398));
#25508=CARTESIAN_POINT('Ctrl Pts',(99.9400048992461,1.77561095934877,-0.0476422453347091));
#25509=CARTESIAN_POINT('Ctrl Pts',(99.9392792521777,1.77531380150608,-0.0587172213027325));
#25510=CARTESIAN_POINT('Ctrl Pts',(99.9385505341127,1.77491303798314,-0.0697890155623971));
#25511=CARTESIAN_POINT('Ctrl Pts',(99.9369984403196,1.77384358538345,-0.0932584136990634));
#25512=CARTESIAN_POINT('Ctrl Pts',(99.9361742979604,1.77314844128254,-0.105654101208776));
#25513=CARTESIAN_POINT('Ctrl Pts',(99.9344996615558,1.7714802627955,-0.130700875105751));
#25514=CARTESIAN_POINT('Ctrl Pts',(99.9336490360991,1.77050150043317,-0.143350838123707));
#25515=CARTESIAN_POINT('Ctrl Pts',(99.9316524489825,1.76789937283275,-0.172866848806497));
#25516=CARTESIAN_POINT('Ctrl Pts',(99.9305032412245,1.76617004982319,-0.189722060810516));
#25517=CARTESIAN_POINT('Ctrl Pts',(99.9268197043723,1.75989646429347,-0.243306607235349));
#25518=CARTESIAN_POINT('Ctrl Pts',(99.9242575803557,1.75444560647524,-0.2799177247912));
#25519=CARTESIAN_POINT('Ctrl Pts',(99.9188907561589,1.74081754955114,-0.355218525302948));
#25520=CARTESIAN_POINT('Ctrl Pts',(99.9160828625299,1.73248391536634,-0.393859182768566));
#25521=CARTESIAN_POINT('Ctrl Pts',(99.9068863343339,1.70131242095907,-0.518120979208936));
#25522=CARTESIAN_POINT('Ctrl Pts',(99.9003871154567,1.6733577245273,-0.602316659261444));
#25523=CARTESIAN_POINT('Ctrl Pts',(99.8885033207208,1.61070886918589,-0.752442737875994));
#25524=CARTESIAN_POINT('Ctrl Pts',(99.8831240293653,1.57792324616843,-0.818970971649752));
#25525=CARTESIAN_POINT('Ctrl Pts',(99.8766607461606,1.53209825313043,-0.898924294433005));
#25526=CARTESIAN_POINT('Ctrl Pts',(99.875405976219,1.52288289342607,-0.914449397219466));
#25527=CARTESIAN_POINT('Ctrl Pts',(99.8735533210496,1.50877398085504,-0.937413630721445));
#25528=CARTESIAN_POINT('Ctrl Pts',(99.8729450395149,1.50405891905455,-0.944960325588245));
#25529=CARTESIAN_POINT('Ctrl Pts',(99.8719017297436,1.49582496966288,-0.957921401550772));
#25530=CARTESIAN_POINT('Ctrl Pts',(99.871465004197,1.49233303364727,-0.963352413437259));
#25531=CARTESIAN_POINT('Ctrl Pts',(99.8704414561022,1.48404183626071,-0.976094445538943));
#25532=CARTESIAN_POINT('Ctrl Pts',(99.8698562650296,1.47921810449177,-0.983389213818415));
#25533=CARTESIAN_POINT('Ctrl Pts',(99.8681121966172,1.46459806209791,-1.00514761448588));
#25534=CARTESIAN_POINT('Ctrl Pts',(99.8669633910738,1.45464174386018,-1.01950314568186));
#25535=CARTESIAN_POINT('Ctrl Pts',(99.8570888886245,1.36638987041332,-1.14282360682151));
#25536=CARTESIAN_POINT('Ctrl Pts',(99.8490232228396,1.2761820275638,-1.24275373112078));
#25537=CARTESIAN_POINT('Ctrl Pts',(99.8354415165225,1.11083491621752,-1.38872823491735));
#25538=CARTESIAN_POINT('Ctrl Pts',(99.8300658307838,1.04202826893568,-1.44107423976197));
#25539=CARTESIAN_POINT('Ctrl Pts',(99.822815779425,0.947837441630749,-1.50244757922321));
#25540=CARTESIAN_POINT('Ctrl Pts',(99.8211175361908,0.925671531266362,-1.51620468467212));
#25541=CARTESIAN_POINT('Ctrl Pts',(99.8184414050231,0.890646570793234,-1.53688831335412));
#25542=CARTESIAN_POINT('Ctrl Pts',(99.8174758928225,0.877990887495211,-1.54415316007862));
#25543=CARTESIAN_POINT('Ctrl Pts',(99.8156630005511,0.854202879532878,-1.55742140577891));
#25544=CARTESIAN_POINT('Ctrl Pts',(99.8148170862501,0.843093095928934,-1.56346346673544));
#25545=CARTESIAN_POINT('Ctrl Pts',(99.8129112722668,0.818047393114282,-1.57674000765449));
#25546=CARTESIAN_POINT('Ctrl Pts',(99.8118491340533,0.80407831081921,-1.58390928760646));
#25547=CARTESIAN_POINT('Ctrl Pts',(99.8090994969535,0.767899129692909,-1.60187539864835));
#25548=CARTESIAN_POINT('Ctrl Pts',(99.8074025790595,0.745556248085736,-1.61239562138282));
#25549=CARTESIAN_POINT('Ctrl Pts',(99.7983819927947,0.626753416003302,-1.66533710957251));
#25550=CARTESIAN_POINT('Ctrl Pts',(99.790789515764,0.526894156329278,-1.69957157426181));
#25551=CARTESIAN_POINT('Ctrl Pts',(99.7770031165378,0.343660052257937,-1.74468083967509));
#25552=CARTESIAN_POINT('Ctrl Pts',(99.770869800802,0.261409366537865,-1.75888585157346));
#25553=CARTESIAN_POINT('Ctrl Pts',(99.7629159480555,0.151270746352097,-1.77000796365344));
#25554=CARTESIAN_POINT('Ctrl Pts',(99.7609691631254,0.124017058489385,-1.77212611326942));
#25555=CARTESIAN_POINT('Ctrl Pts',(99.7576745026277,0.0772252176373467,
-1.77467790295851));
#25556=CARTESIAN_POINT('Ctrl Pts',(99.7563145813094,0.057709255188337,-1.7754197008849));
#25557=CARTESIAN_POINT('Ctrl Pts',(99.7543430091102,0.0290627801484523,
-1.77603565654665));
#25558=CARTESIAN_POINT('Ctrl Pts',(99.7537187894799,0.0199398800334438,
-1.77616150981563));
#25559=CARTESIAN_POINT('Ctrl Pts',(99.7526123540901,0.00366713514776551,
-1.77626060169673));
#25560=CARTESIAN_POINT('Ctrl Pts',(99.7521287122019,-0.00348198047841314,
-1.7762609755629));
#25561=CARTESIAN_POINT('Ctrl Pts',(99.7510521069026,-0.0194762158373868,
-1.77616524410506));
#25562=CARTESIAN_POINT('Ctrl Pts',(99.7504604057516,-0.0283208211096542,
-1.77604623723244));
#25563=CARTESIAN_POINT('Ctrl Pts',(99.7486847258366,-0.0550129008027708,
-1.7754876377026));
#25564=CARTESIAN_POINT('Ctrl Pts',(99.7475112590055,-0.0728555946040405,
-1.77484503353384));
#25565=CARTESIAN_POINT('Ctrl Pts',(99.7398221239447,-0.190856629995937,
-1.76881262694266));
#25566=CARTESIAN_POINT('Ctrl Pts',(99.7336685694406,-0.290426464850753,
-1.75521564326854));
#25567=CARTESIAN_POINT('Ctrl Pts',(99.7248323280064,-0.430893613010248,
-1.72374525363767));
#25568=CARTESIAN_POINT('Ctrl Pts',(99.7221578903596,-0.473094878815755,
-1.71264361633276));
#25569=CARTESIAN_POINT('Ctrl Pts',(99.7153225145289,-0.578965032774141,
-1.68058089631236));
#25570=CARTESIAN_POINT('Ctrl Pts',(99.7111369461174,-0.641930697904599,
-1.6575513342473));
#25571=CARTESIAN_POINT('Ctrl Pts',(99.7048149888961,-0.732513790773486,
-1.61848386212147));
#25572=CARTESIAN_POINT('Ctrl Pts',(99.7027636764108,-0.761243948389654,
-1.60517099380572));
#25573=CARTESIAN_POINT('Ctrl Pts',(99.6996521933884,-0.803719061091138,
-1.58409220598707));
#25574=CARTESIAN_POINT('Ctrl Pts',(99.6986117595525,-0.817742190328487,
-1.57689889647653));
#25575=CARTESIAN_POINT('Ctrl Pts',(99.6967181221554,-0.842928011231842,
-1.56355327239801));
#25576=CARTESIAN_POINT('Ctrl Pts',(99.6958672457838,-0.854123844266056,
-1.55746554114823));
#25577=CARTESIAN_POINT('Ctrl Pts',(99.69402118773,-0.878147613338086,-1.54406568295718));
#25578=CARTESIAN_POINT('Ctrl Pts',(99.6930245993296,-0.890951739418545,
-1.5367130633913));
#25579=CARTESIAN_POINT('Ctrl Pts',(99.6902667353676,-0.925923183817079,
-1.51604713323828));
#25580=CARTESIAN_POINT('Ctrl Pts',(99.6884938009734,-0.947893001584265,
-1.50240852890187));
#25581=CARTESIAN_POINT('Ctrl Pts',(99.6767724349312,-1.08975192908441,-1.40999395846063));
#25582=CARTESIAN_POINT('Ctrl Pts',(99.6662955626293,-1.19999981145682,-1.31743224038946));
#25583=CARTESIAN_POINT('Ctrl Pts',(99.6503314610838,-1.34924967021319,-1.15769038922376));
#25584=CARTESIAN_POINT('Ctrl Pts',(99.6448692042926,-1.39706286175475,-1.09951770787243));
#25585=CARTESIAN_POINT('Ctrl Pts',(99.6383198288909,-1.45166331899783,-1.02375163381629));
#25586=CARTESIAN_POINT('Ctrl Pts',(99.6370577693318,-1.46205375954034,-1.00885710946254));
#25587=CARTESIAN_POINT('Ctrl Pts',(99.6351965077656,-1.4772052608326,-0.986411805413159));
#25588=CARTESIAN_POINT('Ctrl Pts',(99.6345867946377,-1.48214045131977,-0.978980757547719));
#25589=CARTESIAN_POINT('Ctrl Pts',(99.6335408124788,-1.49056155263733,-0.966091226365382));
#25590=CARTESIAN_POINT('Ctrl Pts',(99.6331028493312,-1.49407382481972,-0.960650513844036));
#25591=CARTESIAN_POINT('Ctrl Pts',(99.6320752740193,-1.50228194358447,-0.947781748736228));
#25592=CARTESIAN_POINT('Ctrl Pts',(99.6314873073003,-1.5069525203552,-0.940337913113716));
#25593=CARTESIAN_POINT('Ctrl Pts',(99.6297726079399,-1.52048907246235,-0.918403832452889));
#25594=CARTESIAN_POINT('Ctrl Pts',(99.6286551172428,-1.52920293552013,-0.903820254677063));
#25595=CARTESIAN_POINT('Ctrl Pts',(99.6187106805063,-1.60560059805604,-0.771691766231914));
#25596=CARTESIAN_POINT('Ctrl Pts',(99.6105574799591,-1.65983126352376,-0.646863368455838));
#25597=CARTESIAN_POINT('Ctrl Pts',(99.5983844292871,-1.71732902175815,-0.457897146413347));
#25598=CARTESIAN_POINT('Ctrl Pts',(99.5945429649507,-1.7322284499121,-0.397834817794887));
#25599=CARTESIAN_POINT('Ctrl Pts',(99.58799479525,-1.75180934750379,-0.296540702316916));
#25600=CARTESIAN_POINT('Ctrl Pts',(99.5853367672581,-1.75823454459147,-0.255701484365897));
#25601=CARTESIAN_POINT('Ctrl Pts',(99.5814973861227,-1.7653311808215,-0.197414115403766));
#25602=CARTESIAN_POINT('Ctrl Pts',(99.5803526893854,-1.76717934810694,-0.180121145564705));
#25603=CARTESIAN_POINT('Ctrl Pts',(99.5783439666791,-1.76995701254263,-0.149943454102504));
#25604=CARTESIAN_POINT('Ctrl Pts',(99.577483578208,-1.77100044245696,-0.137070359363327));
#25605=CARTESIAN_POINT('Ctrl Pts',(99.5756919457403,-1.7728710226764,-0.110380939572005));
#25606=CARTESIAN_POINT('Ctrl Pts',(99.5747601053092,-1.77367724657241,-0.0965640770739489));
#25607=CARTESIAN_POINT('Ctrl Pts',(99.5723208687671,-1.77535556627284,-0.0605730682739813));
#25608=CARTESIAN_POINT('Ctrl Pts',(99.5708056613789,-1.77597370635523,-0.0383900994893181));
#25609=CARTESIAN_POINT('Ctrl Pts',(99.5633995410787,-1.77695471708159,0.0691536612728943));
#25610=CARTESIAN_POINT('Ctrl Pts',(99.5573340018839,-1.77157955834121,0.154441982225163));
#25611=CARTESIAN_POINT('Ctrl Pts',(99.5434710263297,-1.74582305589433,0.344121463576641));
#25612=CARTESIAN_POINT('Ctrl Pts',(99.5356332822249,-1.72216148013362,0.447746490714757));
#25613=CARTESIAN_POINT('Ctrl Pts',(99.5257745371451,-1.6799104182754,0.577847852038138));
#25614=CARTESIAN_POINT('Ctrl Pts',(99.5235801883268,-1.66966848831537,0.606806810991485));
#25615=CARTESIAN_POINT('Ctrl Pts',(99.5199159153223,-1.65106312672038,0.655368524575739));
#25616=CARTESIAN_POINT('Ctrl Pts',(99.5184305741234,-1.64308874987426,0.675112443245771));
#25617=CARTESIAN_POINT('Ctrl Pts',(99.5163113338566,-1.63105426898313,0.703431482326731));
#25618=CARTESIAN_POINT('Ctrl Pts',(99.5156623728187,-1.62727781093949,0.71212415697693));
#25619=CARTESIAN_POINT('Ctrl Pts',(99.5145282781634,-1.62051380663837,0.727358766740251));
#25620=CARTESIAN_POINT('Ctrl Pts',(99.5140414411001,-1.61755586197693,0.733913355206157));
#25621=CARTESIAN_POINT('Ctrl Pts',(99.5129767898867,-1.61096676102347,0.748280946912124));
#25622=CARTESIAN_POINT('Ctrl Pts',(99.5124000171557,-1.60731848528246,0.756085693070234));
#25623=CARTESIAN_POINT('Ctrl Pts',(99.5107471456957,-1.5966410717615,0.778501265610848));
#25624=CARTESIAN_POINT('Ctrl Pts',(99.5096793495866,-1.58946828092328,0.793043228406025));
#25625=CARTESIAN_POINT('Ctrl Pts',(99.5008415912529,-1.52789425438043,0.913684502815119));
#25626=CARTESIAN_POINT('Ctrl Pts',(99.493601590606,-1.46312834122856,1.01417143867414));
#25627=CARTESIAN_POINT('Ctrl Pts',(99.4804804603201,-1.32992641536686,1.18121472859065));
#25628=CARTESIAN_POINT('Ctrl Pts',(99.4746531293541,-1.26529930309067,1.25019504500519));
#25629=CARTESIAN_POINT('Ctrl Pts',(99.4665952006454,-1.17233060216966,1.33479834431371));
#25630=CARTESIAN_POINT('Ctrl Pts',(99.464564864965,-1.1486060131395,1.35526738894227));
#25631=CARTESIAN_POINT('Ctrl Pts',(99.4614804359575,-1.11221992440914,1.38501861360285));
#25632=CARTESIAN_POINT('Ctrl Pts',(99.4604456449017,-1.09995573949492,1.39477850038196));
#25633=CARTESIAN_POINT('Ctrl Pts',(99.4585600797156,-1.07751736270954,1.41215504566552));
#25634=CARTESIAN_POINT('Ctrl Pts',(99.4577115898142,-1.06738742833346,1.41982731461435));
#25635=CARTESIAN_POINT('Ctrl Pts',(99.4558682938061,-1.04531622381875,1.43617404014555));
#25636=CARTESIAN_POINT('Ctrl Pts',(99.4548720571789,-1.03334748611272,1.44480961768282));
#25637=CARTESIAN_POINT('Ctrl Pts',(99.452109095913,-1.00005320888311,1.46820648139115));
#25638=CARTESIAN_POINT('Ctrl Pts',(99.4503305675742,-0.978510575681864,
1.48265087663836));
#25639=CARTESIAN_POINT('Ctrl Pts',(99.4393650406622,-0.845083703505877,
1.56793931940031));
#25640=CARTESIAN_POINT('Ctrl Pts',(99.4297346032892,-0.725899861980511,
1.62654768766169));
#25641=CARTESIAN_POINT('Ctrl Pts',(99.4132261851446,-0.513513059204109,
1.70296219279321));
#25642=CARTESIAN_POINT('Ctrl Pts',(99.406412628982,-0.423323860294552,1.72759267593499));
#25643=CARTESIAN_POINT('Ctrl Pts',(99.3989092240858,-0.317537418872479,
1.7476953949356));
#25644=CARTESIAN_POINT('Ctrl Pts',(99.3979188592608,-0.303434005996591,
1.75019914373216));
#25645=CARTESIAN_POINT('Ctrl Pts',(99.3963811588102,-0.281291185585047,
1.75385439581656));
#25646=CARTESIAN_POINT('Ctrl Pts',(99.395827783108,-0.273271899624891,1.75512177592375));
#25647=CARTESIAN_POINT('Ctrl Pts',(99.3947828513343,-0.258027197697644,
1.75742405182669));
#25648=CARTESIAN_POINT('Ctrl Pts',(99.3942907632141,-0.250803755068399,
1.75846945123871));
#25649=CARTESIAN_POINT('Ctrl Pts',(99.3931074145119,-0.233330856136563,
1.76088832852753));
#25650=CARTESIAN_POINT('Ctrl Pts',(99.3924186187754,-0.223075277598957,
1.76221690702849));
#25651=CARTESIAN_POINT('Ctrl Pts',(99.3900901545508,-0.188141699620423,
1.76643258260177));
#25652=CARTESIAN_POINT('Ctrl Pts',(99.3884720624082,-0.163413785774393,
1.76889158833672));
#25653=CARTESIAN_POINT('Ctrl Pts',(99.3787860734461,-0.0132833053826002,
1.78064552423622));
#25654=CARTESIAN_POINT('Ctrl Pts',(99.3712145071567,0.112775518964679,1.77712229812572));
#25655=CARTESIAN_POINT('Ctrl Pts',(99.3582908978089,0.320502485080232,1.74910580232864));
#25656=CARTESIAN_POINT('Ctrl Pts',(99.3530614820441,0.402682228437745,1.73203281494645));
#25657=CARTESIAN_POINT('Ctrl Pts',(99.3459862975025,0.50818242865288,1.70219886459313));
#25658=CARTESIAN_POINT('Ctrl Pts',(99.3443049547342,0.532863873231661,1.69463457343424));
#25659=CARTESIAN_POINT('Ctrl Pts',(99.3416457711371,0.57122700964473,1.68195622162478));
#25660=CARTESIAN_POINT('Ctrl Pts',(99.3406798730468,0.585025949542344,1.67720650040071));
#25661=CARTESIAN_POINT('Ctrl Pts',(99.3388603405357,0.610755940497993,1.66799384708985));
#25662=CARTESIAN_POINT('Ctrl Pts',(99.338008104977,0.622700613752867,1.66357152651223));
#25663=CARTESIAN_POINT('Ctrl Pts',(99.3360798469588,0.649480136139083,1.65332802326466));
#25664=CARTESIAN_POINT('Ctrl Pts',(99.3350014667269,0.664286113416507,1.64743495482028));
#25665=CARTESIAN_POINT('Ctrl Pts',(99.3321915025723,0.70241576887303,1.63166102944136));
#25666=CARTESIAN_POINT('Ctrl Pts',(99.3304499398288,0.725610252672839,1.62147934731486));
#25667=CARTESIAN_POINT('Ctrl Pts',(99.3188781813886,0.876810879562657,1.55121296927954));
#25668=CARTESIAN_POINT('Ctrl Pts',(99.3085394090597,0.997448841115302,1.47652997338205));
#25669=CARTESIAN_POINT('Ctrl Pts',(99.292757123101,1.16632940484223,1.34176053312714));
#25670=CARTESIAN_POINT('Ctrl Pts',(99.2873316344231,1.22173194500975,1.29151801145696));
#25671=CARTESIAN_POINT('Ctrl Pts',(99.2808222364033,1.28641841376054,1.22495674981306));
#25672=CARTESIAN_POINT('Ctrl Pts',(99.279564782693,1.29882885688778,1.21179001394723));
#25673=CARTESIAN_POINT('Ctrl Pts',(99.2777099214663,1.31703667078401,1.19187145132884));
#25674=CARTESIAN_POINT('Ctrl Pts',(99.2771020453949,1.32298758720841,1.18526241875934));
#25675=CARTESIAN_POINT('Ctrl Pts',(99.2760587791879,1.33317695828544,1.17377383924956));
#25676=CARTESIAN_POINT('Ctrl Pts',(99.2756217056807,1.33743868534919,1.16891556343645));
#25677=CARTESIAN_POINT('Ctrl Pts',(99.2745957466579,1.34742539695441,1.1574048059943));
#25678=CARTESIAN_POINT('Ctrl Pts',(99.2740085084895,1.35312770827142,1.1507330266272));
#25679=CARTESIAN_POINT('Ctrl Pts',(99.2722603634668,1.37005164552685,1.13063203699189));
#25680=CARTESIAN_POINT('Ctrl Pts',(99.2711094941957,1.38112487471722,1.11707853417323));
#25681=CARTESIAN_POINT('Ctrl Pts',(99.2612388272418,1.47528352954298,0.998288507725664));
#25682=CARTESIAN_POINT('Ctrl Pts',(99.2531741563852,1.54641737843456,0.884106868278432));
#25683=CARTESIAN_POINT('Ctrl Pts',(99.2395914388576,1.64112501813017,0.685004458460632));
#25684=CARTESIAN_POINT('Ctrl Pts',(99.2342128648273,1.67248107709777,0.604422902659847));
#25685=CARTESIAN_POINT('Ctrl Pts',(99.2269561200872,1.70553528107832,0.496887753225648));
#25686=CARTESIAN_POINT('Ctrl Pts',(99.2252531992854,1.71266596037846,0.47172367728203));
#25687=CARTESIAN_POINT('Ctrl Pts',(99.2225677244021,1.72292285971994,0.432221963871046));
#25688=CARTESIAN_POINT('Ctrl Pts',(99.2215975234154,1.72643157187855,0.417986856902056));
#25689=CARTESIAN_POINT('Ctrl Pts',(99.2197744587135,1.73265609629284,0.391316851957801));
#25690=CARTESIAN_POINT('Ctrl Pts',(99.2189230534486,1.73541526266783,0.378892964028254));
#25691=CARTESIAN_POINT('Ctrl Pts',(99.2170027972605,1.74130663515942,0.350949990746207));
#25692=CARTESIAN_POINT('Ctrl Pts',(99.2159316676685,1.74436530237799,0.335416691834679));
#25693=CARTESIAN_POINT('Ctrl Pts',(99.2126659819314,1.75300257111312,0.288233924499014));
#25694=CARTESIAN_POINT('Ctrl Pts',(99.2104511826106,1.75793000450438,0.256473537490275));
#25695=CARTESIAN_POINT('Ctrl Pts',(99.2018629622776,1.77350429536551,0.13429209840756));
#25696=CARTESIAN_POINT('Ctrl Pts',(99.1953165639767,1.77804619474441,0.0433090279489397));
#25697=CARTESIAN_POINT('Ctrl Pts',(99.1886897733872,1.77561363837197,-0.0475422940912343));
#25698=CARTESIAN_POINT('Ctrl Pts',(99.0420054636133,1.77561363841465,-0.0475422924970873));
#25699=CARTESIAN_POINT('Ctrl Pts',(99.0432892873456,1.77610074208309,-0.029349902698944));
#25700=CARTESIAN_POINT('Ctrl Pts',(99.0445625357543,1.77630827248011,-0.0111493778985186));
#25701=CARTESIAN_POINT('Ctrl Pts',(99.0466052615637,1.77619111743689,0.0183558676580814));
#25702=CARTESIAN_POINT('Ctrl Pts',(99.0473826964922,1.77603834619032,0.0296586110785028));
#25703=CARTESIAN_POINT('Ctrl Pts',(99.0486612332802,1.77560649672732,0.0483812222678931));
#25704=CARTESIAN_POINT('Ctrl Pts',(99.0491655764023,1.77538877824435,0.0558020332029134));
#25705=CARTESIAN_POINT('Ctrl Pts',(99.0501851804467,1.77485174892134,0.0708806680593242));
#25706=CARTESIAN_POINT('Ctrl Pts',(99.0507002718848,1.77452939136981,0.0785381724348064));
#25707=CARTESIAN_POINT('Ctrl Pts',(99.0520437423076,1.77355436430919,0.0986075615288776));
#25708=CARTESIAN_POINT('Ctrl Pts',(99.0528677924276,1.77282095743971,0.111015354235097));
#25709=CARTESIAN_POINT('Ctrl Pts',(99.0564801458365,1.76900657735169,0.165781198002898));
#25710=CARTESIAN_POINT('Ctrl Pts',(99.0592013510977,1.76453706022991,0.208031907885738));
#25711=CARTESIAN_POINT('Ctrl Pts',(99.0679776109073,1.74494311017726,0.345813207589858));
#25712=CARTESIAN_POINT('Ctrl Pts',(99.0738465368231,1.72353509891961,0.440275213959686));
#25713=CARTESIAN_POINT('Ctrl Pts',(99.0853080267608,1.66770723420564,0.617922978705789));
#25714=CARTESIAN_POINT('Ctrl Pts',(99.0908726661741,1.63445813853118,0.701156341888515));
#25715=CARTESIAN_POINT('Ctrl Pts',(99.0983495247431,1.5834370898929,0.805289649538533));
#25716=CARTESIAN_POINT('Ctrl Pts',(99.1000721935234,1.57126390996472,0.82879071172082));
#25717=CARTESIAN_POINT('Ctrl Pts',(99.1027758685017,1.55155137827189,0.864850584095201));
#25718=CARTESIAN_POINT('Ctrl Pts',(99.1037440752267,1.54437375702883,0.877603492064699));
#25719=CARTESIAN_POINT('Ctrl Pts',(99.1055557270017,1.53073033691304,0.901158786466298));
#25720=CARTESIAN_POINT('Ctrl Pts',(99.1063976436872,1.52430564233796,0.911984000642247));
#25721=CARTESIAN_POINT('Ctrl Pts',(99.108286158266,1.5097109560891,0.935990039442954));
#25722=CARTESIAN_POINT('Ctrl Pts',(99.109334861521,1.50148240390291,0.949133862529524));
#25723=CARTESIAN_POINT('Ctrl Pts',(99.1120325435817,1.48000646096914,0.982460027120919));
#25724=CARTESIAN_POINT('Ctrl Pts',(99.1136903450453,1.46651815381288,1.00248253565721));
#25725=CARTESIAN_POINT('Ctrl Pts',(99.1240115026733,1.3807985323342,1.12429410084689));
#25726=CARTESIAN_POINT('Ctrl Pts',(99.133064532903,1.29842427558394,1.21849329315012));
#25727=CARTESIAN_POINT('Ctrl Pts',(99.1472344620872,1.15626794806983,1.35013572344426));
#25728=CARTESIAN_POINT('Ctrl Pts',(99.1522814701665,1.10296789944966,1.39401749244203));
#25729=CARTESIAN_POINT('Ctrl Pts',(99.1598186615983,1.01792406157426,1.45609504200487));
#25730=CARTESIAN_POINT('Ctrl Pts',(99.1623852570002,0.987947857069246,1.47659798969468));
#25731=CARTESIAN_POINT('Ctrl Pts',(99.1656946796753,0.947699840814268,1.50235170792423));
#25732=CARTESIAN_POINT('Ctrl Pts',(99.1664839158295,0.937977749651262,1.50844071851244));
#25733=CARTESIAN_POINT('Ctrl Pts',(99.1677765901112,0.921837954093644,1.5183327952488));
#25734=CARTESIAN_POINT('Ctrl Pts',(99.168283410278,0.915454204860696,1.52219029561664));
#25735=CARTESIAN_POINT('Ctrl Pts',(99.1693026778979,0.902498735611143,1.52990789784766));
#25736=CARTESIAN_POINT('Ctrl Pts',(99.1698150078892,0.895926124456394,1.53376612582198));
#25737=CARTESIAN_POINT('Ctrl Pts',(99.1711426271564,0.878742626091827,1.54370496389767));
#25738=CARTESIAN_POINT('Ctrl Pts',(99.1719537735807,0.868093205618535,1.54971862785812));
#25739=CARTESIAN_POINT('Ctrl Pts',(99.1754080840351,0.822139438171575,1.57504607861606));
#25740=CARTESIAN_POINT('Ctrl Pts',(99.1779912546023,0.78624375102347,1.59326856488484));
#25741=CARTESIAN_POINT('Ctrl Pts',(99.1867456263915,0.660655153695733,1.65174427654853));
#25742=CARTESIAN_POINT('Ctrl Pts',(99.192710994448,0.568257969306344,1.68576682996564));
#25743=CARTESIAN_POINT('Ctrl Pts',(99.2043192225569,0.386446847465715,1.73605408299114));
#25744=CARTESIAN_POINT('Ctrl Pts',(99.2099325103568,0.297677575490778,1.75345668900032));
#25745=CARTESIAN_POINT('Ctrl Pts',(99.2174686074734,0.181586577711848,1.7671435858428));
#25746=CARTESIAN_POINT('Ctrl Pts',(99.2191980960664,0.155131972944316,1.76966213981009));
#25747=CARTESIAN_POINT('Ctrl Pts',(99.2219101409578,0.114014316283613,1.77264762395241));
#25748=CARTESIAN_POINT('Ctrl Pts',(99.2228797670406,0.0993845283088616,
1.77352799721832));
#25749=CARTESIAN_POINT('Ctrl Pts',(99.2246927561435,0.072173050022952,1.77482775223062));
#25750=CARTESIAN_POINT('Ctrl Pts',(99.2255345730323,0.0595944783970281,
1.77529461873417));
#25751=CARTESIAN_POINT('Ctrl Pts',(99.2274211510333,0.0315374759813947,
1.77603746795361));
#25752=CARTESIAN_POINT('Ctrl Pts',(99.2284679963782,0.0160584200929307,
1.77624485941758));
#25753=CARTESIAN_POINT('Ctrl Pts',(99.2311574066812,-0.0234691334653549,
1.77625774520556));
#25754=CARTESIAN_POINT('Ctrl Pts',(99.2328087009123,-0.0475139116236059,
1.77577721218532));
#25755=CARTESIAN_POINT('Ctrl Pts',(99.2450917824138,-0.224655602862794,
1.76863683066527));
#25756=CARTESIAN_POINT('Ctrl Pts',(99.2563388094861,-0.376304968175417,
1.74267701529871));
#25757=CARTESIAN_POINT('Ctrl Pts',(99.2711077324227,-0.569878370148193,
1.68307431336017));
#25758=CARTESIAN_POINT('Ctrl Pts',(99.2746851855186,-0.616430079077429,
1.66658784751913));
#25759=CARTESIAN_POINT('Ctrl Pts',(99.2802968719213,-0.689626156049868,
1.63717778371984));
#25760=CARTESIAN_POINT('Ctrl Pts',(99.2823722837504,-0.716738624041437,
1.62549110103071));
#25761=CARTESIAN_POINT('Ctrl Pts',(99.2851499516887,-0.753234740449387,
1.6086687768326));
#25762=CARTESIAN_POINT('Ctrl Pts',(99.285882505262,-0.762880381969297,1.60411699849026));
#25763=CARTESIAN_POINT('Ctrl Pts',(99.2871077919186,-0.779058113458006,
1.59630379509152));
#25764=CARTESIAN_POINT('Ctrl Pts',(99.2876032382343,-0.785612063855842,
1.59308852338859));
#25765=CARTESIAN_POINT('Ctrl Pts',(99.2886269539362,-0.799183429840687,
1.58632648709598));
#25766=CARTESIAN_POINT('Ctrl Pts',(99.2891548325884,-0.806197392030392,
1.58277340427916));
#25767=CARTESIAN_POINT('Ctrl Pts',(99.2905711823503,-0.825051300539528,
1.57306467766297));
#25768=CARTESIAN_POINT('Ctrl Pts',(99.2914544336315,-0.836846123196716,
1.56682185368301));
#25769=CARTESIAN_POINT('Ctrl Pts',(99.295917550194,-0.896560469117792,1.53434922623438));
#25770=CARTESIAN_POINT('Ctrl Pts',(99.2993848921658,-0.943326691737096,
1.50604920374993));
#25771=CARTESIAN_POINT('Ctrl Pts',(99.3096805000545,-1.0802687265442,1.41429409752211));
#25772=CARTESIAN_POINT('Ctrl Pts',(99.3163307999408,-1.16591373935445,1.34456500967248));
#25773=CARTESIAN_POINT('Ctrl Pts',(99.3276975514788,-1.29649112588474,1.21633672839006));
#25774=CARTESIAN_POINT('Ctrl Pts',(99.3322896698326,-1.34524478937329,1.16218712138409));
#25775=CARTESIAN_POINT('Ctrl Pts',(99.3383701899041,-1.4034568537298,1.08894636090368));
#25776=CARTESIAN_POINT('Ctrl Pts',(99.3397303704078,-1.41609155920959,1.07246443014137));
#25777=CARTESIAN_POINT('Ctrl Pts',(99.3419900545939,-1.43642708980782,1.04495077513096));
#25778=CARTESIAN_POINT('Ctrl Pts',(99.3428829094727,-1.44429693340484,1.03404606185917));
#25779=CARTESIAN_POINT('Ctrl Pts',(99.3446317015374,-1.45938570938459,1.01263023048757));
#25780=CARTESIAN_POINT('Ctrl Pts',(99.3454871010975,-1.46661678643711,1.00212864418156));
#25781=CARTESIAN_POINT('Ctrl Pts',(99.3475482328559,-1.48367972825955,0.976768118861398));
#25782=CARTESIAN_POINT('Ctrl Pts',(99.348757980751,-1.49340213502523,0.961837572949676));
#25783=CARTESIAN_POINT('Ctrl Pts',(99.3528383497562,-1.52521093968469,0.911344101748684));
#25784=CARTESIAN_POINT('Ctrl Pts',(99.3557458916567,-1.546263014484,0.875149511328884));
#25785=CARTESIAN_POINT('Ctrl Pts',(99.3693812403015,-1.63760254700222,0.704508843364687));
#25786=CARTESIAN_POINT('Ctrl Pts',(99.3806267310964,-1.69175624209207,0.562159362751232));
#25787=CARTESIAN_POINT('Ctrl Pts',(99.3953467076809,-1.73926485341889,0.364292562724473));
#25788=CARTESIAN_POINT('Ctrl Pts',(99.3990499103184,-1.74915637591595,0.313375705525583));
#25789=CARTESIAN_POINT('Ctrl Pts',(99.4035403303765,-1.75869429079464,0.249443505924488));
#25790=CARTESIAN_POINT('Ctrl Pts',(99.404422573216,-1.76044502314089,0.236772074930093));
#25791=CARTESIAN_POINT('Ctrl Pts',(99.4058272285281,-1.76303551462548,0.216401895961216));
#25792=CARTESIAN_POINT('Ctrl Pts',(99.4063541936045,-1.76396204485191,0.208714916883869));
#25793=CARTESIAN_POINT('Ctrl Pts',(99.4073711786707,-1.76566233481554,0.193787507265233));
#25794=CARTESIAN_POINT('Ctrl Pts',(99.4078614863327,-1.76644188193674,0.186548006820078));
#25795=CARTESIAN_POINT('Ctrl Pts',(99.4090833226112,-1.76828260252271,0.168406290473624));
#25796=CARTESIAN_POINT('Ctrl Pts',(99.4098117893353,-1.76928751227249,0.157498429045854));
#25797=CARTESIAN_POINT('Ctrl Pts',(99.4124814728353,-1.77262301164909,0.117217305697917));
#25798=CARTESIAN_POINT('Ctrl Pts',(99.4143914517961,-1.77432367816289,0.087794992966839));
#25799=CARTESIAN_POINT('Ctrl Pts',(99.4195064829357,-1.7769513627159,0.007837107781896));
#25800=CARTESIAN_POINT('Ctrl Pts',(99.4226592852629,-1.77645526996791,-0.0427192022554856));
#25801=CARTESIAN_POINT('Ctrl Pts',(99.4333140768053,-1.76741283978097,-0.214837798277852));
#25802=CARTESIAN_POINT('Ctrl Pts',(99.4406721279363,-1.74852552867487,-0.335501403474995));
#25803=CARTESIAN_POINT('Ctrl Pts',(99.4512606222229,-1.70575649953419,-0.497548848671729));
#25804=CARTESIAN_POINT('Ctrl Pts',(99.4541933857084,-1.69236706164545,-0.541343952642791));
#25805=CARTESIAN_POINT('Ctrl Pts',(99.4583827222333,-1.67123666944194,-0.60197317309261));
#25806=CARTESIAN_POINT('Ctrl Pts',(99.4595936261781,-1.66490119705217,-0.619279959715436));
#25807=CARTESIAN_POINT('Ctrl Pts',(99.4616646285539,-1.6536901188701,-0.648489320709872));
#25808=CARTESIAN_POINT('Ctrl Pts',(99.4625200751906,-1.64895234383836,-0.660443458012944));
#25809=CARTESIAN_POINT('Ctrl Pts',(99.4642681155468,-1.63905775038948,-0.68463871422407));
#25810=CARTESIAN_POINT('Ctrl Pts',(99.4651609475684,-1.63389258630172,-0.696875511043717));
#25811=CARTESIAN_POINT('Ctrl Pts',(99.4674065458348,-1.62062764647262,-0.727343135443157));
#25812=CARTESIAN_POINT('Ctrl Pts',(99.4687650640643,-1.61235724381205,-0.745497194371389));
#25813=CARTESIAN_POINT('Ctrl Pts',(99.4744715500483,-1.5766155052103,-0.820574385555406));
#25814=CARTESIAN_POINT('Ctrl Pts',(99.4789118357835,-1.54642456437316,-0.876143927188428));
#25815=CARTESIAN_POINT('Ctrl Pts',(99.4932409811137,-1.44156772339623,-1.04677536934854));
#25816=CARTESIAN_POINT('Ctrl Pts',(99.5034209365941,-1.35652492448684,-1.15485551100838));
#25817=CARTESIAN_POINT('Ctrl Pts',(99.5162287698012,-1.23093010844199,-1.2812357384225));
#25818=CARTESIAN_POINT('Ctrl Pts',(99.5191467371018,-1.20094684118452,-1.30938199797962));
#25819=CARTESIAN_POINT('Ctrl Pts',(99.5228541013217,-1.16074990438188,-1.34457251024279));
#25820=CARTESIAN_POINT('Ctrl Pts',(99.523702366848,-1.151404098962,-1.35258426654439));
#25821=CARTESIAN_POINT('Ctrl Pts',(99.5250661439311,-1.13612464304131,-1.36540953859781));
#25822=CARTESIAN_POINT('Ctrl Pts',(99.525585765161,-1.1302420886398,-1.37028290483263));
#25823=CARTESIAN_POINT('Ctrl Pts',(99.526606500248,-1.11856221181205,-1.37983263907232));
#25824=CARTESIAN_POINT('Ctrl Pts',(99.5271077231788,-1.11276659650673,-1.38451075799837));
#25825=CARTESIAN_POINT('Ctrl Pts',(99.5283704100267,-1.09801839484495,-1.39626281538049));
#25826=CARTESIAN_POINT('Ctrl Pts',(99.5291284701099,-1.08902656769191,-1.40328735364925));
#25827=CARTESIAN_POINT('Ctrl Pts',(99.5322371657803,-1.05161410817432,-1.43193826852985));
#25828=CARTESIAN_POINT('Ctrl Pts',(99.5345403861176,-1.02261016355933,-1.45279327288942));
#25829=CARTESIAN_POINT('Ctrl Pts',(99.5410686892214,-0.937396972408941,
-1.51024744135645));
#25830=CARTESIAN_POINT('Ctrl Pts',(99.5452028114585,-0.879716984612754,
-1.5445580849568));
#25831=CARTESIAN_POINT('Ctrl Pts',(99.5571705698544,-0.706942612411793,
-1.63450576244057));
#25832=CARTESIAN_POINT('Ctrl Pts',(99.5649597770886,-0.587635972053866,
-1.68108800140466));
#25833=CARTESIAN_POINT('Ctrl Pts',(99.5747368687377,-0.441255290506512,
-1.72073570980605));
#25834=CARTESIAN_POINT('Ctrl Pts',(99.5762941741049,-0.418015931223066,
-1.72652836876657));
#25835=CARTESIAN_POINT('Ctrl Pts',(99.57888080784,-0.379600569687917,-1.73528276347286));
#25836=CARTESIAN_POINT('Ctrl Pts',(99.5799013564955,-0.364489968487033,
-1.73851945614003));
#25837=CARTESIAN_POINT('Ctrl Pts',(99.5817647772732,-0.336996623264775,
-1.74403434989305));
#25838=CARTESIAN_POINT('Ctrl Pts',(99.5826054707985,-0.324628107014912,
-1.74637885803619));
#25839=CARTESIAN_POINT('Ctrl Pts',(99.5844360142161,-0.297780001545141,
-1.75117297027572));
#25840=CARTESIAN_POINT('Ctrl Pts',(99.5854273162199,-0.283292957181344,
-1.75357485695897));
#25841=CARTESIAN_POINT('Ctrl Pts',(99.5882374014438,-0.242383623576375,
-1.75983727631489));
#25842=CARTESIAN_POINT('Ctrl Pts',(99.5900690870497,-0.215902653926874,
-1.76328187455139));
#25843=CARTESIAN_POINT('Ctrl Pts',(99.5982463802858,-0.0985510470303378,
-1.77586371933742));
#25844=CARTESIAN_POINT('Ctrl Pts',(99.6047844694313,-0.00714448441541827,
-1.77858055815757));
#25845=CARTESIAN_POINT('Ctrl Pts',(99.6187152633795,0.18410631529159,-1.76952024871536));
#25846=CARTESIAN_POINT('Ctrl Pts',(99.6261058465728,0.283578968985655,-1.7563258846063));
#25847=CARTESIAN_POINT('Ctrl Pts',(99.6359917403932,0.41823895901789,-1.72672005651326));
#25848=CARTESIAN_POINT('Ctrl Pts',(99.638661994828,0.454803647013667,-1.71745162617049));
#25849=CARTESIAN_POINT('Ctrl Pts',(99.6421078547935,0.502559990141931,-1.70371388540186));
#25850=CARTESIAN_POINT('Ctrl Pts',(99.642932833974,0.514038270888048,-1.70028592385774));
#25851=CARTESIAN_POINT('Ctrl Pts',(99.6442685228136,0.532709532106138,-1.6945034299695));
#25852=CARTESIAN_POINT('Ctrl Pts',(99.6447830490297,0.539923475066438,-1.69221865203481));
#25853=CARTESIAN_POINT('Ctrl Pts',(99.6458020449293,0.554257689050783,-1.68757776708112));
#25854=CARTESIAN_POINT('Ctrl Pts',(99.6463065436914,0.561378053054144,-1.6852225348353));
#25855=CARTESIAN_POINT('Ctrl Pts',(99.647590608685,0.579554388520755,-1.67908228699703));
#25856=CARTESIAN_POINT('Ctrl Pts',(99.6483665187982,0.590588539889225,-1.67523306155811));
#25857=CARTESIAN_POINT('Ctrl Pts',(99.65167105263,0.637755546053814,-1.65825504946743));
#25858=CARTESIAN_POINT('Ctrl Pts',(99.6541443323714,0.67349767890683,-1.64406305052046));
#25859=CARTESIAN_POINT('Ctrl Pts',(99.6614132597729,0.778731644759576,-1.59826946346361));
#25860=CARTESIAN_POINT('Ctrl Pts',(99.6660916153545,0.846679010947396,-1.5633376052402));
#25861=CARTESIAN_POINT('Ctrl Pts',(99.6777899807179,1.01024025450393,-1.46544899385541));
#25862=CARTESIAN_POINT('Ctrl Pts',(99.6848042723125,1.1024038474716,-1.39743626646984));
#25863=CARTESIAN_POINT('Ctrl Pts',(99.6937429759855,1.20560634216282,-1.30467513652625));
#25864=CARTESIAN_POINT('Ctrl Pts',(99.695334491446,1.22347957194752,-1.28792915481132));
#25865=CARTESIAN_POINT('Ctrl Pts',(99.6979654092271,1.2521631673138,-1.2599186120261));
#25866=CARTESIAN_POINT('Ctrl Pts',(99.6989954639974,1.26318170084049,-1.24887127888373));
#25867=CARTESIAN_POINT('Ctrl Pts',(99.7008680235581,1.28282208906133,-1.22865370659812));
#25868=CARTESIAN_POINT('Ctrl Pts',(99.7017082223326,1.29149481100285,-1.21953416599933));
#25869=CARTESIAN_POINT('Ctrl Pts',(99.7035282682852,1.30997696920059,-1.19968154373612));
#25870=CARTESIAN_POINT('Ctrl Pts',(99.7045094603304,1.31975292581889,-1.18891869320682));
#25871=CARTESIAN_POINT('Ctrl Pts',(99.7072634834585,1.34666338271397,-1.15855069276903));
#25872=CARTESIAN_POINT('Ctrl Pts',(99.7090484322009,1.3634999659923,-1.13868770583191));
#25873=CARTESIAN_POINT('Ctrl Pts',(99.7168278763477,1.43425942801717,-1.05138886750474));
#25874=CARTESIAN_POINT('Ctrl Pts',(99.7229935416995,1.48365521374533,-0.98044992566828));
#25875=CARTESIAN_POINT('Ctrl Pts',(99.7390288130308,1.59629557601057,-0.79056043226644));
#25876=CARTESIAN_POINT('Ctrl Pts',(99.7490176642994,1.65154522841434,-0.667492573692244));
#25877=CARTESIAN_POINT('Ctrl Pts',(99.7596586726682,1.69766493002482,-0.522781801265699));
#25878=CARTESIAN_POINT('Ctrl Pts',(99.7608674685648,1.70270649283093,-0.506120225278715));
#25879=CARTESIAN_POINT('Ctrl Pts',(99.7626612353024,1.70990012536191,-0.481021154106113));
#25880=CARTESIAN_POINT('Ctrl Pts',(99.7632558419026,1.71223626194066,-0.472638107588769));
#25881=CARTESIAN_POINT('Ctrl Pts',(99.7642810533036,1.71618127765296,-0.458068486587766));
#25882=CARTESIAN_POINT('Ctrl Pts',(99.7647132303375,1.71781846469908,-0.451890077013478));
#25883=CARTESIAN_POINT('Ctrl Pts',(99.7657333970947,1.72162137440022,-0.437219291168476));
#25884=CARTESIAN_POINT('Ctrl Pts',(99.7663197064307,1.72375764248461,-0.428719562719988));
#25885=CARTESIAN_POINT('Ctrl Pts',(99.7680802292582,1.73001878357742,-0.403004273451283));
#25886=CARTESIAN_POINT('Ctrl Pts',(99.7692440941399,1.7339494347153,-0.385741950330786));
#25887=CARTESIAN_POINT('Ctrl Pts',(99.7750666825079,1.75250225611509,-0.298239851186436));
#25888=CARTESIAN_POINT('Ctrl Pts',(99.7795450193971,1.763118914875,-0.227211598628625));
#25889=CARTESIAN_POINT('Ctrl Pts',(99.7862063381242,1.77257983483769,-0.119715507923802));
#25890=CARTESIAN_POINT('Ctrl Pts',(99.7884223183664,1.77464721044379,-0.0836365264494882));
#25891=CARTESIAN_POINT('Ctrl Pts',(99.7906385404719,1.77561363837197,-0.0475422940912529));
#25892=CARTESIAN_POINT('Origin',(88.3562164250559,0.,0.));
#25893=CARTESIAN_POINT('',(100.349869898682,-0.11727379276914,-1.77237437355361));
#25894=CARTESIAN_POINT('Ctrl Pts',(99.7906385404719,1.77561363837197,-0.0475422940912529));
#25895=CARTESIAN_POINT('Ctrl Pts',(99.7964931379277,1.7781666525646,0.0478078968502291));
#25896=CARTESIAN_POINT('Ctrl Pts',(99.8023587123669,1.77303685265072,0.143263940921935));
#25897=CARTESIAN_POINT('Ctrl Pts',(99.8107947900208,1.75531046788573,0.274421537102804));
#25898=CARTESIAN_POINT('Ctrl Pts',(99.8131725253114,1.74923995707394,0.310775302863875));
#25899=CARTESIAN_POINT('Ctrl Pts',(99.8166590559928,1.73884174739516,0.362990650705894));
#25900=CARTESIAN_POINT('Ctrl Pts',(99.8177394055839,1.73541749313107,0.379023653154207));
#25901=CARTESIAN_POINT('Ctrl Pts',(99.8196698378899,1.7289457704255,0.407396722334368));
#25902=CARTESIAN_POINT('Ctrl Pts',(99.8205170332232,1.72598681844863,0.419755946467089));
#25903=CARTESIAN_POINT('Ctrl Pts',(99.8223018592488,1.71950719328883,0.445592975642046));
#25904=CARTESIAN_POINT('Ctrl Pts',(99.8232402929298,1.71596009639686,0.459063193945807));
#25905=CARTESIAN_POINT('Ctrl Pts',(99.8257451941639,1.70612447016286,0.494706490924222));
#25906=CARTESIAN_POINT('Ctrl Pts',(99.8273204131688,1.69956236915572,0.51680062505471));
#25907=CARTESIAN_POINT('Ctrl Pts',(99.8371210260799,1.65644934391702,0.652244844617913));
#25908=CARTESIAN_POINT('Ctrl Pts',(99.8457053012009,1.6090108339211,0.761788915842328));
#25909=CARTESIAN_POINT('Ctrl Pts',(99.8622288396868,1.49878525081889,0.95925809194317));
#25910=CARTESIAN_POINT('Ctrl Pts',(99.8701051645889,1.43823314635055,1.04786563122638));
#25911=CARTESIAN_POINT('Ctrl Pts',(99.8788255728269,1.35900400659355,1.14388552079713));
#25912=CARTESIAN_POINT('Ctrl Pts',(99.880032118174,1.34774881689578,1.15712538543225));
#25913=CARTESIAN_POINT('Ctrl Pts',(99.88182385533,1.33056559766765,1.17674765100802));
#25914=CARTESIAN_POINT('Ctrl Pts',(99.8824186231808,1.32478233477899,1.18325467138048));
#25915=CARTESIAN_POINT('Ctrl Pts',(99.8834451532781,1.31465846148942,1.19447824188463));
#25916=CARTESIAN_POINT('Ctrl Pts',(99.8838784755474,1.3103399516301,1.19921405715651));
#25917=CARTESIAN_POINT('Ctrl Pts',(99.8849028899476,1.30002390826394,1.21040469578874));
#25918=CARTESIAN_POINT('Ctrl Pts',(99.8854922784282,1.29400386830803,1.21683839792716));
#25919=CARTESIAN_POINT('Ctrl Pts',(99.887266350407,1.27563525445852,1.23617871322627));
#25920=CARTESIAN_POINT('Ctrl Pts',(99.8884405157298,1.26313922334615,1.24894454465055));
#25921=CARTESIAN_POINT('Ctrl Pts',(99.8943601328358,1.19854138109877,1.31297562898711));
#25922=CARTESIAN_POINT('Ctrl Pts',(99.8989193420682,1.14349806820828,1.36118365845796));
#25923=CARTESIAN_POINT('Ctrl Pts',(99.9118385786317,0.977832497260549,1.48911351408132));
#25924=CARTESIAN_POINT('Ctrl Pts',(99.9200734028822,0.860822258658605,1.5596788529844));
#25925=CARTESIAN_POINT('Ctrl Pts',(99.9308564995049,0.707663326519199,1.62951195839032));
#25926=CARTESIAN_POINT('Ctrl Pts',(99.9329377705117,0.678071051601471,1.64204629957554));
#25927=CARTESIAN_POINT('Ctrl Pts',(99.936079338257,0.633489645552694,1.65951893390905));
#25928=CARTESIAN_POINT('Ctrl Pts',(99.937119141254,0.618747359725876,1.66507174057476));
#25929=CARTESIAN_POINT('Ctrl Pts',(99.9390041654468,0.592059809403849,1.67472047197822));
#25930=CARTESIAN_POINT('Ctrl Pts',(99.9398469900029,0.580140901425605,1.67888653504072));
#25931=CARTESIAN_POINT('Ctrl Pts',(99.9416669293301,0.554440053742645,1.68756349768375));
#25932=CARTESIAN_POINT('Ctrl Pts',(99.9426453277446,0.540645338890821,1.69203337074829));
#25933=CARTESIAN_POINT('Ctrl Pts',(99.9453754435427,0.502224343950848,1.70396504131501));
#25934=CARTESIAN_POINT('Ctrl Pts',(99.9471388696398,0.477489164643469,1.71106111244297));
#25935=CARTESIAN_POINT('Ctrl Pts',(99.9547220431117,0.371519166192495,1.73898529049829));
#25936=CARTESIAN_POINT('Ctrl Pts',(99.9607023952819,0.289028596435848,1.75458122753618));
#25937=CARTESIAN_POINT('Ctrl Pts',(99.9758780197278,0.081262821903158,1.778811285086));
#25938=CARTESIAN_POINT('Ctrl Pts',(99.985173949752,-0.0444159527475959,
1.78011275838108));
#25939=CARTESIAN_POINT('Ctrl Pts',(99.9958587893048,-0.19451352868987,1.76575080219603));
#25940=CARTESIAN_POINT('Ctrl Pts',(99.9976423189186,-0.219787471432643,
1.7627833211611));
#25941=CARTESIAN_POINT('Ctrl Pts',(100.000114885196,-0.255247737791905,
1.75784524555791));
#25942=CARTESIAN_POINT('Ctrl Pts',(100.000825719795,-0.265492664041288,
1.75632712597737));
#25943=CARTESIAN_POINT('Ctrl Pts',(100.00202503367,-0.282873654983778,1.75359600164842));
#25944=CARTESIAN_POINT('Ctrl Pts',(100.002515985675,-0.290016567911134,
1.75242884010167));
#25945=CARTESIAN_POINT('Ctrl Pts',(100.003538950127,-0.304961934473112,
1.74989286107541));
#25946=CARTESIAN_POINT('Ctrl Pts',(100.004070480329,-0.312762670649016,
1.74851546311266));
#25947=CARTESIAN_POINT('Ctrl Pts',(100.005518719217,-0.334104275838643,
1.74459972001398));
#25948=CARTESIAN_POINT('Ctrl Pts',(100.006429700227,-0.347625568253119,
1.74195589601152));
#25949=CARTESIAN_POINT('Ctrl Pts',(100.012153421272,-0.43308167373984,1.72421193189544));
#25950=CARTESIAN_POINT('Ctrl Pts',(100.016756745132,-0.504060492846061,
1.70481441871399));
#25951=CARTESIAN_POINT('Ctrl Pts',(100.02867172964,-0.686569426825445,1.64253596242109));
#25952=CARTESIAN_POINT('Ctrl Pts',(100.035870955795,-0.795323744137146,
1.59272145887288));
#25953=CARTESIAN_POINT('Ctrl Pts',(100.046476249517,-0.94060713377943,1.50755812215496));
#25954=CARTESIAN_POINT('Ctrl Pts',(100.049612366414,-0.981901512499782,
1.48099359455273));
#25955=CARTESIAN_POINT('Ctrl Pts',(100.054038846053,-1.03744670155824,1.44191651361706));
#25956=CARTESIAN_POINT('Ctrl Pts',(100.055275417571,-1.05267907079813,1.43083388963728));
#25957=CARTESIAN_POINT('Ctrl Pts',(100.057295797944,-1.07708780796221,1.41247406189004));
#25958=CARTESIAN_POINT('Ctrl Pts',(100.058073789185,-1.08637377432647,1.4053444890062));
#25959=CARTESIAN_POINT('Ctrl Pts',(100.059715485944,-1.10572718867635,1.39017889607518));
#25960=CARTESIAN_POINT('Ctrl Pts',(100.060579913049,-1.11577901766145,1.38212414325002));
#25961=CARTESIAN_POINT('Ctrl Pts',(100.062673981084,-1.13979101463918,1.36245013697342));
#25962=CARTESIAN_POINT('Ctrl Pts',(100.063907900593,-1.15366204688499,1.3507249058492));
#25963=CARTESIAN_POINT('Ctrl Pts',(100.068431585451,-1.20349248880167,1.30727551335372));
#25964=CARTESIAN_POINT('Ctrl Pts',(100.071772331565,-1.23834035196693,1.2743138762924));
#25965=CARTESIAN_POINT('Ctrl Pts',(100.080716097545,-1.32655504491058,1.18383517070582));
#25966=CARTESIAN_POINT('Ctrl Pts',(100.08640116284,-1.37751662942011,1.12412620287644));
#25967=CARTESIAN_POINT('Ctrl Pts',(100.100193513115,-1.49029171226726,0.972764769369427));
#25968=CARTESIAN_POINT('Ctrl Pts',(100.108322645641,-1.54783656701778,0.878320211017495));
#25969=CARTESIAN_POINT('Ctrl Pts',(100.117253056011,-1.6037611972641,0.763745715978466));
#25970=CARTESIAN_POINT('Ctrl Pts',(100.118442500313,-1.61105239074613,0.748243105745587));
#25971=CARTESIAN_POINT('Ctrl Pts',(100.12021206701,-1.62167681018176,0.724777766537858));
#25972=CARTESIAN_POINT('Ctrl Pts',(100.120801525421,-1.62517791596065,0.716892765267462));
#25973=CARTESIAN_POINT('Ctrl Pts',(100.121865493586,-1.63143048744985,0.702529823315676));
#25974=CARTESIAN_POINT('Ctrl Pts',(100.122341090928,-1.63420099995054,0.696060832479135));
#25975=CARTESIAN_POINT('Ctrl Pts',(100.123431519087,-1.64049557533343,0.681118590770222));
#25976=CARTESIAN_POINT('Ctrl Pts',(100.124044738171,-1.64399251618068,0.672634286469225));
#25977=CARTESIAN_POINT('Ctrl Pts',(100.125970939406,-1.65483375951348,0.645741497425132));
#25978=CARTESIAN_POINT('Ctrl Pts',(100.12727059158,-1.66193609061336,0.627236290186909));
#25979=CARTESIAN_POINT('Ctrl Pts',(100.130365537081,-1.67828239749075,0.582417273933465));
#25980=CARTESIAN_POINT('Ctrl Pts',(100.13214689171,-1.68721950536279,0.555996578154497));
#25981=CARTESIAN_POINT('Ctrl Pts',(100.139388530913,-1.72137497511728,0.446600285214749));
#25982=CARTESIAN_POINT('Ctrl Pts',(100.144677507945,-1.7411241685882,0.362038905240627));
#25983=CARTESIAN_POINT('Ctrl Pts',(100.156192531159,-1.77028828940717,0.176880812480538));
#25984=CARTESIAN_POINT('Ctrl Pts',(100.1624167039,-1.77746729641969,0.0762515473305784));
#25985=CARTESIAN_POINT('Ctrl Pts',(100.170503652907,-1.7757399584398,-0.049288293428972));
#25986=CARTESIAN_POINT('Ctrl Pts',(100.172118675183,-1.77487652381352,-0.0741280254872288));
#25987=CARTESIAN_POINT('Ctrl Pts',(100.174783874909,-1.77261439996511,-0.11467621371666));
#25988=CARTESIAN_POINT('Ctrl Pts',(100.175824420483,-1.77152716548375,-0.130399081014327));
#25989=CARTESIAN_POINT('Ctrl Pts',(100.177713247363,-1.76918879768221,-0.158731110894724));
#25990=CARTESIAN_POINT('Ctrl Pts',(100.1785591612,-1.76801167852979,-0.171345434039105));
#25991=CARTESIAN_POINT('Ctrl Pts',(100.180388596644,-1.76518858407098,-0.198459725023159));
#25992=CARTESIAN_POINT('Ctrl Pts',(100.181373437265,-1.76349866436725,-0.212954076099071));
#25993=CARTESIAN_POINT('Ctrl Pts',(100.18412998137,-1.75829911352762,-0.253229608198164));
#25994=CARTESIAN_POINT('Ctrl Pts',(100.18591364563,-1.75440143670731,-0.278956057226832));
#25995=CARTESIAN_POINT('Ctrl Pts',(100.193654462878,-1.73522562382617,-0.389126828354918));
#25996=CARTESIAN_POINT('Ctrl Pts',(100.199778930604,-1.71440618092535,-0.472477938770434));
#25997=CARTESIAN_POINT('Ctrl Pts',(100.215758291561,-1.64573007071061,-0.681690225334595));
#25998=CARTESIAN_POINT('Ctrl Pts',(100.225732072662,-1.58945147911387,-0.804223648557327));
#25999=CARTESIAN_POINT('Ctrl Pts',(100.236360272327,-1.51089579874509,-0.934109162755003));
#26000=CARTESIAN_POINT('Ctrl Pts',(100.237566452318,-1.50168445839896,-0.948846608274311));
#26001=CARTESIAN_POINT('Ctrl Pts',(100.239360746398,-1.48751214229155,-0.970797734955737));
#26002=CARTESIAN_POINT('Ctrl Pts',(100.239958336748,-1.48271201375453,-0.978113341094658));
#26003=CARTESIAN_POINT('Ctrl Pts',(100.241044264017,-1.47383879528095,-0.991421078291027));
#26004=CARTESIAN_POINT('Ctrl Pts',(100.241533627991,-1.46978298334533,-0.997423948534114));
#26005=CARTESIAN_POINT('Ctrl Pts',(100.24265665706,-1.46034494559226,-1.01121028597273));
#26006=CARTESIAN_POINT('Ctrl Pts',(100.243288632095,-1.45493709641348,-1.01897578867778));
#26007=CARTESIAN_POINT('Ctrl Pts',(100.245298897122,-1.43743486561957,-1.04368501502761));
#26008=CARTESIAN_POINT('Ctrl Pts',(100.246662715023,-1.42510411452673,-1.06046016221564));
#26009=CARTESIAN_POINT('Ctrl Pts',(100.249940084928,-1.39444202574328,-1.10067277560797));
#26010=CARTESIAN_POINT('Ctrl Pts',(100.251837960713,-1.37581088016087,-1.12387443024082));
#26011=CARTESIAN_POINT('Ctrl Pts',(100.260015852776,-1.29218072667421,-1.2228219534349));
#26012=CARTESIAN_POINT('Ctrl Pts',(100.266086711509,-1.22144413596312,-1.2934840281648));
#26013=CARTESIAN_POINT('Ctrl Pts',(100.277662150094,-1.07847096798431,-1.41406198557683));
#26014=CARTESIAN_POINT('Ctrl Pts',(100.283125091899,-1.00775549094225,-1.46529764574405));
#26015=CARTESIAN_POINT('Ctrl Pts',(100.290221680105,-0.914734817061573,
-1.52276537288529));
#26016=CARTESIAN_POINT('Ctrl Pts',(100.291670065379,-0.895685677918712,
-1.53404734704009));
#26017=CARTESIAN_POINT('Ctrl Pts',(100.294045044164,-0.864386076516734,
-1.55180300017576));
#26018=CARTESIAN_POINT('Ctrl Pts',(100.294963867128,-0.852261632047777,
-1.5584947651689));
#26019=CARTESIAN_POINT('Ctrl Pts',(100.296752076926,-0.828644702208023,
-1.57117150139329));
#26020=CARTESIAN_POINT('Ctrl Pts',(100.297620782814,-0.817162507140867,
-1.57717384932715));
#26021=CARTESIAN_POINT('Ctrl Pts',(100.299673488765,-0.790016696886263,
-1.59098838352615));
#26022=CARTESIAN_POINT('Ctrl Pts',(100.300861028043,-0.774301481547401,
-1.59869559191857));
#26023=CARTESIAN_POINT('Ctrl Pts',(100.304918676448,-0.720588396485923,
-1.6240603277503));
#26024=CARTESIAN_POINT('Ctrl Pts',(100.30782579467,-0.682083190217163,-1.64060403581061));
#26025=CARTESIAN_POINT('Ctrl Pts',(100.31520079313,-0.58440537653619,-1.67853801187126));
#26026=CARTESIAN_POINT('Ctrl Pts',(100.319716751716,-0.524616485653908,
-1.6981742315184));
#26027=CARTESIAN_POINT('Ctrl Pts',(100.332814292871,-0.350563757656464,
-1.74526754135083));
#26028=CARTESIAN_POINT('Ctrl Pts',(100.341510471993,-0.234449217791222,
-1.76462115464189));
#26029=CARTESIAN_POINT('Ctrl Pts',(100.349869898682,-0.11727379276914,-1.77237437355361));
#26030=CARTESIAN_POINT('',(100.349869898682,-1.70764710160359,-0.4888818250711));
#26031=CARTESIAN_POINT('Origin',(100.349869898682,0.,0.));
#26032=CARTESIAN_POINT('',(100.129086829157,0.00137221428264897,1.77624946995853));
#26033=CARTESIAN_POINT('Ctrl Pts',(100.128149994198,0.00130396094780403,
1.77624952137526));
#26034=CARTESIAN_POINT('Ctrl Pts',(100.135254863005,-0.0957291980175613,
1.77632075430082));
#26035=CARTESIAN_POINT('Ctrl Pts',(100.142452083519,-0.192611897045183,
1.76844057705337));
#26036=CARTESIAN_POINT('Ctrl Pts',(100.153400526873,-0.341559757154774,
1.74393434377953));
#26037=CARTESIAN_POINT('Ctrl Pts',(100.157258709097,-0.394330021920698,
1.73276509497843));
#26038=CARTESIAN_POINT('Ctrl Pts',(100.163670309496,-0.482710034608528,
1.70981096361842));
#26039=CARTESIAN_POINT('Ctrl Pts',(100.166260022626,-0.518601382447507,
1.69926910775185));
#26040=CARTESIAN_POINT('Ctrl Pts',(100.16991347725,-0.569481615602692,1.68256222428895));
#26041=CARTESIAN_POINT('Ctrl Pts',(100.171008143872,-0.584758490520812,
1.67731406971457));
#26042=CARTESIAN_POINT('Ctrl Pts',(100.17290921631,-0.611336589015278,1.66777626711555));
#26043=CARTESIAN_POINT('Ctrl Pts',(100.173718736893,-0.622669344120547,
1.66357837301651));
#26044=CARTESIAN_POINT('Ctrl Pts',(100.175391216247,-0.646108810887612,
1.65462281025941));
#26045=CARTESIAN_POINT('Ctrl Pts',(100.176253489696,-0.658207907909286,
1.64984714612651));
#26046=CARTESIAN_POINT('Ctrl Pts',(100.178490484007,-0.689623498788055,
1.63704641687366));
#26047=CARTESIAN_POINT('Ctrl Pts',(100.179857819311,-0.708852990212084,
1.6288121567253));
#26048=CARTESIAN_POINT('Ctrl Pts',(100.186204135166,-0.798129580645457,
1.58870241649473));
#26049=CARTESIAN_POINT('Ctrl Pts',(100.191033393552,-0.866206930111896,
1.55263449281232));
#26050=CARTESIAN_POINT('Ctrl Pts',(100.202812077758,-1.02848006103079,1.45265444116518));
#26051=CARTESIAN_POINT('Ctrl Pts',(100.209639196324,-1.11927360515802,1.38390744305321));
#26052=CARTESIAN_POINT('Ctrl Pts',(100.218737239276,-1.22586488352479,1.28580545218075));
#26053=CARTESIAN_POINT('Ctrl Pts',(100.220722514642,-1.24829200097628,1.26404399448709));
#26054=CARTESIAN_POINT('Ctrl Pts',(100.223704015737,-1.28051401528967,1.23108426857808));
#26055=CARTESIAN_POINT('Ctrl Pts',(100.224672574085,-1.2907618765233,1.22033534914517));
#26056=CARTESIAN_POINT('Ctrl Pts',(100.226417402782,-1.30880378400833,1.20092979266328));
#26057=CARTESIAN_POINT('Ctrl Pts',(100.227190040689,-1.31664984729168,1.19232247019853));
#26058=CARTESIAN_POINT('Ctrl Pts',(100.228453023708,-1.32923194661045,1.17824396755008));
#26059=CARTESIAN_POINT('Ctrl Pts',(100.22893945945,-1.33402037658051,1.17281969967129));
#26060=CARTESIAN_POINT('Ctrl Pts',(100.229911944483,-1.34347635260876,1.16197526391989));
#26061=CARTESIAN_POINT('Ctrl Pts',(100.2303978796,-1.34814446962376,1.15655596851853));
#26062=CARTESIAN_POINT('Ctrl Pts',(100.231586371648,-1.35942674043813,1.14329707703154));
#26063=CARTESIAN_POINT('Ctrl Pts',(100.232291379014,-1.3660058696929,1.13542820998825));
#26064=CARTESIAN_POINT('Ctrl Pts',(100.23469829316,-1.38809593824661,1.10853783602053));
#26065=CARTESIAN_POINT('Ctrl Pts',(100.236420556478,-1.40327988636873,1.08925289997557));
#26066=CARTESIAN_POINT('Ctrl Pts',(100.240873730137,-1.44107521640734,1.03914730809804));
#26067=CARTESIAN_POINT('Ctrl Pts',(100.243630531566,-1.46309966175944,1.00790074423885));
#26068=CARTESIAN_POINT('Ctrl Pts',(100.257223945286,-1.56571370811657,0.851861914884223));
#26069=CARTESIAN_POINT('Ctrl Pts',(100.268300822581,-1.63145237939817,0.717983898341546));
#26070=CARTESIAN_POINT('Ctrl Pts',(100.283007746724,-1.69847099997986,0.523043288335931));
#26071=CARTESIAN_POINT('Ctrl Pts',(100.287043275869,-1.71453080141143,0.467721480528988));
#26072=CARTESIAN_POINT('Ctrl Pts',(100.292459079198,-1.73280383288821,0.391033029518842));
#26073=CARTESIAN_POINT('Ctrl Pts',(100.293908267301,-1.73735965123781,0.370266741216327));
#26074=CARTESIAN_POINT('Ctrl Pts',(100.296231649236,-1.74411536231491,0.336595930652565));
#26075=CARTESIAN_POINT('Ctrl Pts',(100.29711255254,-1.74654723182124,0.323740635635537));
#26076=CARTESIAN_POINT('Ctrl Pts',(100.29895096592,-1.75134785091464,0.296733246809969));
#26077=CARTESIAN_POINT('Ctrl Pts',(100.29990758161,-1.75368760646362,0.282576913609874));
#26078=CARTESIAN_POINT('Ctrl Pts',(100.302203418469,-1.7589165702476,0.248368533556482));
#26079=CARTESIAN_POINT('Ctrl Pts',(100.303537768131,-1.76163480209468,0.228292142238424));
#26080=CARTESIAN_POINT('Ctrl Pts',(100.308235613119,-1.77004853425795,0.156996165263256));
#26081=CARTESIAN_POINT('Ctrl Pts',(100.311548657578,-1.77385835962502,0.105578141115755));
#26082=CARTESIAN_POINT('Ctrl Pts',(100.319609588662,-1.77771670573629,-0.0211273285827478));
#26083=CARTESIAN_POINT('Ctrl Pts',(100.324307062743,-1.77522748861565,-0.0963891624062148));
#26084=CARTESIAN_POINT('Ctrl Pts',(100.334017882365,-1.76031064369582,-0.250373579713448));
#26085=CARTESIAN_POINT('Ctrl Pts',(100.339023932768,-1.7473475234668,-0.32886927391282));
#26086=CARTESIAN_POINT('Ctrl Pts',(100.345236306438,-1.72559434857467,-0.421465625819561));
#26087=CARTESIAN_POINT('Ctrl Pts',(100.346265671596,-1.72181296112772,-0.436656873573249));
#26088=CARTESIAN_POINT('Ctrl Pts',(100.347762245216,-1.71607028779066,-0.458491843083625));
#26089=CARTESIAN_POINT('Ctrl Pts',(100.348222803322,-1.71427006020475,-0.465177557974144));
#26090=CARTESIAN_POINT('Ctrl Pts',(100.349078977483,-1.71086361427569,-0.477540114841893));
#26091=CARTESIAN_POINT('Ctrl Pts',(100.349473448819,-1.70927082021505,-0.483210232799742));
#26092=CARTESIAN_POINT('Ctrl Pts',(100.349869898682,-1.70764710160359,-0.4888818250711));
#26093=CARTESIAN_POINT('Ctrl Pts',(99.938371422543,1.77561385491717,-0.0475342058543041));
#26094=CARTESIAN_POINT('Ctrl Pts',(99.9429651167472,1.7774525533391,0.0211493523185398));
#26095=CARTESIAN_POINT('Ctrl Pts',(99.9475588109513,1.77529901241746,0.089836337665965));
#26096=CARTESIAN_POINT('Ctrl Pts',(99.9521525051555,1.76920256918782,0.158070654073485));
#26097=CARTESIAN_POINT('Ctrl Pts',(99.9567561361381,1.76309293853142,0.226452570485825));
#26098=CARTESIAN_POINT('Ctrl Pts',(99.9613597671207,1.7530234469905,0.294379482442791));
#26099=CARTESIAN_POINT('Ctrl Pts',(99.9659633981033,1.73909474169064,0.361404955588548));
#26100=CARTESIAN_POINT('Ctrl Pts',(99.9705844437525,1.72511334672927,0.428683973440486));
#26101=CARTESIAN_POINT('Ctrl Pts',(99.9752054894016,1.70724363047171,0.495054354679337));
#26102=CARTESIAN_POINT('Ctrl Pts',(99.9798265350508,1.68563674621482,0.560082870931005));
#26103=CARTESIAN_POINT('Ctrl Pts',(99.9840236069088,1.66601226016998,0.619145121393658));
#26104=CARTESIAN_POINT('Ctrl Pts',(99.9882206787669,1.64330561823309,0.677100483889278));
#26105=CARTESIAN_POINT('Ctrl Pts',(99.9924177506249,1.61766340334978,0.733641040266147));
#26106=CARTESIAN_POINT('Ctrl Pts',(99.996719443715,1.59138199995517,0.791590994162829));
#26107=CARTESIAN_POINT('Ctrl Pts',(100.001021136805,1.56193031631559,0.848242522556317));
#26108=CARTESIAN_POINT('Ctrl Pts',(100.005322829895,1.52945925765464,0.903226683438055));
#26109=CARTESIAN_POINT('Ctrl Pts',(100.009749731426,1.49604307098206,0.959811256280128));
#26110=CARTESIAN_POINT('Ctrl Pts',(100.014176632958,1.45942912853903,1.01462935526712));
#26111=CARTESIAN_POINT('Ctrl Pts',(100.018603534489,1.4198350438754,1.0673015087984));
#26112=CARTESIAN_POINT('Ctrl Pts',(100.022893633379,1.38146451824141,1.11834595734265));
#26113=CARTESIAN_POINT('Ctrl Pts',(100.02718373227,1.34029569218185,1.1673747307569));
#26114=CARTESIAN_POINT('Ctrl Pts',(100.03147383116,1.29657165064649,1.21407002155552));
#26115=CARTESIAN_POINT('Ctrl Pts',(100.035761382289,1.25287357550642,1.26073758142316));
#26116=CARTESIAN_POINT('Ctrl Pts',(100.040048933419,1.20662363749741,1.30507404058467));
#26117=CARTESIAN_POINT('Ctrl Pts',(100.044336484548,1.15810445639107,1.34679550436848));
#26118=CARTESIAN_POINT('Ctrl Pts',(100.048623025896,1.10959670226696,1.38850714213267));
#26119=CARTESIAN_POINT('Ctrl Pts',(100.052909567244,1.05882114733742,1.4276046794328));
#26120=CARTESIAN_POINT('Ctrl Pts',(100.057196108593,1.00609497862374,1.4638432144489));
#26121=CARTESIAN_POINT('Ctrl Pts',(100.061483176441,0.953362333746309,1.50008620051262));
#26122=CARTESIAN_POINT('Ctrl Pts',(100.065770244289,0.898679015852326,1.5334692051429));
#26123=CARTESIAN_POINT('Ctrl Pts',(100.070057312138,0.842391150091806,1.56379065502611));
#26124=CARTESIAN_POINT('Ctrl Pts',(100.074349204795,0.786039936085563,1.59414622968262));
#26125=CARTESIAN_POINT('Ctrl Pts',(100.078641097453,0.728081015997666,1.62143313850311));
#26126=CARTESIAN_POINT('Ctrl Pts',(100.082932990111,0.668883993757652,1.64549635836571));
#26127=CARTESIAN_POINT('Ctrl Pts',(100.087227806043,0.609646651508125,1.66957596806038));
#26128=CARTESIAN_POINT('Ctrl Pts',(100.091522621976,0.549170004807765,1.69042735741353));
#26129=CARTESIAN_POINT('Ctrl Pts',(100.095817437908,0.487839665905936,1.70794511705405));
#26130=CARTESIAN_POINT('Ctrl Pts',(100.100119519895,0.42640556712641,1.72549251358605));
#26131=CARTESIAN_POINT('Ctrl Pts',(100.104421601882,0.364115384978533,1.7396949214122));
#26132=CARTESIAN_POINT('Ctrl Pts',(100.108723683869,0.301364584863964,1.75049805755098));
#26133=CARTESIAN_POINT('Ctrl Pts',(100.109671944794,0.287533111647908,1.75287927480846));
#26134=CARTESIAN_POINT('Ctrl Pts',(100.110620205719,0.273679273198215,1.75509554040592));
#26135=CARTESIAN_POINT('Ctrl Pts',(100.111568466644,0.259807318327067,1.75714661307578));
#26136=CARTESIAN_POINT('Ctrl Pts',(100.117407920815,0.174382892857341,1.76977725569591));
#26137=CARTESIAN_POINT('Ctrl Pts',(100.123247374986,0.0880030702956733,
1.77618254461952));
#26138=CARTESIAN_POINT('Ctrl Pts',(100.129086829157,0.00137221428264898,
1.77624946995853));
#26139=CARTESIAN_POINT('Origin',(70.8,0.,0.));
#26140=CARTESIAN_POINT('',(69.8,0.,1.22464679914735E-16));
#26141=CARTESIAN_POINT('Origin',(70.8,0.,0.));
#26142=CARTESIAN_POINT('',(69.8,0.,1.22464679914735E-16));
#26143=CARTESIAN_POINT('Origin',(70.8,0.,0.));
#26144=CARTESIAN_POINT('Origin',(66.9212607628943,0.,0.));
#26145=CARTESIAN_POINT('',(100.349820515151,0.479516069206331,2.15120439274675));
#26146=CARTESIAN_POINT('Ctrl Pts',(99.6260484068026,-0.00167252030352779,
2.20399936539824));
#26147=CARTESIAN_POINT('Ctrl Pts',(99.6319075205934,-0.109497489706828,
2.20391754166753));
#26148=CARTESIAN_POINT('Ctrl Pts',(99.6377666343843,-0.217027700916224,
2.19592210702929));
#26149=CARTESIAN_POINT('Ctrl Pts',(99.6436257481752,-0.323376599163019,
2.18014760397404));
#26150=CARTESIAN_POINT('Ctrl Pts',(99.6476982151888,-0.397296033995319,
2.16918329339042));
#26151=CARTESIAN_POINT('Ctrl Pts',(99.6517706822024,-0.470800001612205,
2.15443410450263));
#26152=CARTESIAN_POINT('Ctrl Pts',(99.655843149216,-0.543470878609583,2.1359436799933));
#26153=CARTESIAN_POINT('Ctrl Pts',(99.6599096309551,-0.616034951759509,
2.11748043072336));
#26154=CARTESIAN_POINT('Ctrl Pts',(99.6639761126941,-0.687767906160161,
2.09528697922465));
#26155=CARTESIAN_POINT('Ctrl Pts',(99.6680425944332,-0.758259772046648,
2.06945841178212));
#26156=CARTESIAN_POINT('Ctrl Pts',(99.6721043188555,-0.82866917054216,2.0436600607985));
#26157=CARTESIAN_POINT('Ctrl Pts',(99.6761660432778,-0.897839918948113,
2.01423520635791));
#26158=CARTESIAN_POINT('Ctrl Pts',(99.6802277677001,-0.965376331664208,
1.98132898284524));
#26159=CARTESIAN_POINT('Ctrl Pts',(99.6842869148638,-1.03286989095618,1.94844363909648));
#26160=CARTESIAN_POINT('Ctrl Pts',(99.6883460620275,-1.09873074412541,1.91208151843965));
#26161=CARTESIAN_POINT('Ctrl Pts',(99.6924052091912,-1.16258360835439,1.87243567408488));
#26162=CARTESIAN_POINT('Ctrl Pts',(99.6964630934742,-1.22641660669966,1.83280216433315));
#26163=CARTESIAN_POINT('Ctrl Pts',(99.7005209777573,-1.28824245095615,1.78988721103953));
#26164=CARTESIAN_POINT('Ctrl Pts',(99.7045788620403,-1.34771229727502,1.74392877256317));
#26165=CARTESIAN_POINT('Ctrl Pts',(99.7086367961383,-1.40718287365091,1.69796976989702));
#26166=CARTESIAN_POINT('Ctrl Pts',(99.7126947302363,-1.46429701784226,1.64896750133811));
#26167=CARTESIAN_POINT('Ctrl Pts',(99.7167526643343,-1.51873790819427,1.59720104126365));
#26168=CARTESIAN_POINT('Ctrl Pts',(99.7208147569618,-1.57323458901551,1.54538153144885));
#26169=CARTESIAN_POINT('Ctrl Pts',(99.7248768495893,-1.62505219845158,1.49079250321318));
#26170=CARTESIAN_POINT('Ctrl Pts',(99.7289389422167,-1.67391040222215,1.43375031485));
#26171=CARTESIAN_POINT('Ctrl Pts',(99.7330031604474,-1.72279417240918,1.3766782775724));
#26172=CARTESIAN_POINT('Ctrl Pts',(99.737067378678,-1.76871516112033,1.31715090239909));
#26173=CARTESIAN_POINT('Ctrl Pts',(99.7411315969086,-1.81143468416356,1.25551598357379));
#26174=CARTESIAN_POINT('Ctrl Pts',(99.7452030889128,-1.85423066278052,1.19377075609463));
#26175=CARTESIAN_POINT('Ctrl Pts',(99.7492745809169,-1.89381347915068,1.12991085748517));
#26176=CARTESIAN_POINT('Ctrl Pts',(99.7533460729211,-1.92998920718614,1.06431088510126));
#26177=CARTESIAN_POINT('Ctrl Pts',(99.7564895366788,-1.95791928536689,1.01366332507036));
#26178=CARTESIAN_POINT('Ctrl Pts',(99.7596330004366,-1.9838193552616,0.961979094348991));
#26179=CARTESIAN_POINT('Ctrl Pts',(99.7627764641943,-2.00762000554835,0.909438240521063));
#26180=CARTESIAN_POINT('Ctrl Pts',(99.7668503345384,-2.03846520398165,0.841346274854084));
#26181=CARTESIAN_POINT('Ctrl Pts',(99.7709242048826,-2.06590167641681,0.77155217677183));
#26182=CARTESIAN_POINT('Ctrl Pts',(99.7749980752268,-2.08973983899598,0.700430871187907));
#26183=CARTESIAN_POINT('Ctrl Pts',(99.7790659583805,-2.11354296766243,0.629414089499418));
#26184=CARTESIAN_POINT('Ctrl Pts',(99.7831338415343,-2.13375813556486,0.557074421736932));
#26185=CARTESIAN_POINT('Ctrl Pts',(99.7872017246881,-2.15024315109428,0.483808217346638));
#26186=CARTESIAN_POINT('Ctrl Pts',(99.791264841114,-2.16670884955418,0.410627865976101));
#26187=CARTESIAN_POINT('Ctrl Pts',(99.79532795754,-2.17945297566547,0.336523598353343));
#26188=CARTESIAN_POINT('Ctrl Pts',(99.799391073966,-2.18838314651579,0.261906861394773));
#26189=CARTESIAN_POINT('Ctrl Pts',(99.8034516067101,-2.19730763878879,0.187337572230529));
#26190=CARTESIAN_POINT('Ctrl Pts',(99.8075121394541,-2.2024229319316,0.112256933073733));
#26191=CARTESIAN_POINT('Ctrl Pts',(99.8115726721982,-2.2036879743073,0.0370851977666151));
#26192=CARTESIAN_POINT('Ctrl Pts',(99.8156319337375,-2.20495262064433,-0.0380630040093736));
#26193=CARTESIAN_POINT('Ctrl Pts',(99.8196911952767,-2.20236940143706,-0.113301768433216));
#26194=CARTESIAN_POINT('Ctrl Pts',(99.8237504568159,-2.19594933265433,-0.188208736287638));
#26195=CARTESIAN_POINT('Ctrl Pts',(99.8278097579377,-2.1895292012684,-0.263116434572969));
#26196=CARTESIAN_POINT('Ctrl Pts',(99.8318690590596,-2.17927218856319,-0.337691854502154));
#26197=CARTESIAN_POINT('Ctrl Pts',(99.8359283601814,-2.16524121855838,-0.411517272366319));
#26198=CARTESIAN_POINT('Ctrl Pts',(99.8399917946099,-2.1511959617833,-0.485417861568273));
#26199=CARTESIAN_POINT('Ctrl Pts',(99.8440552290384,-2.13336916319436,-0.558566453773009));
#26200=CARTESIAN_POINT('Ctrl Pts',(99.8481186634669,-2.11187485349889,-0.630555789093284));
#26201=CARTESIAN_POINT('Ctrl Pts',(99.8521842116242,-2.09036936283288,-0.702582572028724));
#26202=CARTESIAN_POINT('Ctrl Pts',(99.8562497597815,-2.0651927217192,-0.773448447030229));
#26203=CARTESIAN_POINT('Ctrl Pts',(99.8603153079388,-2.03650795310874,-0.842764117013095));
#26204=CARTESIAN_POINT('Ctrl Pts',(99.8643880953861,-2.00777210716519,-0.912203213460093));
#26205=CARTESIAN_POINT('Ctrl Pts',(99.8684608828333,-1.97551586144112,-0.980086159530162));
#26206=CARTESIAN_POINT('Ctrl Pts',(99.8725336702806,-1.9399490218486,-1.04604674495391));
#26207=CARTESIAN_POINT('Ctrl Pts',(99.8756648402583,-1.91260513961213,-1.09675742098638));
#26208=CARTESIAN_POINT('Ctrl Pts',(99.8787960102359,-1.88330547707187,-1.14633233670067));
#26209=CARTESIAN_POINT('Ctrl Pts',(99.8819271802136,-1.852162309428,-1.19461741973501));
#26210=CARTESIAN_POINT('Ctrl Pts',(99.8860008808318,-1.81164456615917,-1.25743706032109));
#26211=CARTESIAN_POINT('Ctrl Pts',(99.8900745814501,-1.76784935617139,-1.31831374420271));
#26212=CARTESIAN_POINT('Ctrl Pts',(99.8941482820683,-1.72098914358945,-1.3768850233942));
#26213=CARTESIAN_POINT('Ctrl Pts',(99.8982160097284,-1.67419763858216,-1.43537042396254));
#26214=CARTESIAN_POINT('Ctrl Pts',(99.9022837373885,-1.62435034917707,-1.49155676147313));
#26215=CARTESIAN_POINT('Ctrl Pts',(99.9063514650486,-1.57170341901845,-1.54510982219573));
#26216=CARTESIAN_POINT('Ctrl Pts',(99.9104144477303,-1.51911790116863,-1.59860041361399));
#26217=CARTESIAN_POINT('Ctrl Pts',(99.914477430412,-1.46373956386138,-1.64946349240418));
#26218=CARTESIAN_POINT('Ctrl Pts',(99.9185404130937,-1.40586422196226,-1.69739853582075));
#26219=CARTESIAN_POINT('Ctrl Pts',(99.9226008254423,-1.34802549328917,-1.74530325446479));
#26220=CARTESIAN_POINT('Ctrl Pts',(99.926661237791,-1.287693261377,-1.79028330987578));
#26221=CARTESIAN_POINT('Ctrl Pts',(99.9307216501396,-1.22519854720158,-1.83207655951795));
#26222=CARTESIAN_POINT('Ctrl Pts',(99.9347808046823,-1.16272319219846,-1.87385686274167));
#26223=CARTESIAN_POINT('Ctrl Pts',(99.938839959225,-1.0980870814465,-1.912452055093));
#26224=CARTESIAN_POINT('Ctrl Pts',(99.9428991137678,-1.03165120709997,-1.94764262299046));
#26225=CARTESIAN_POINT('Ctrl Pts',(99.9469583213553,-0.965214464572138,
-1.98283365075684));
#26226=CARTESIAN_POINT('Ctrl Pts',(99.9510175289429,-0.89697833435288,-2.01461974390755));
#26227=CARTESIAN_POINT('Ctrl Pts',(99.9550767365305,-0.82732802653297,-2.04282753469623));
#26228=CARTESIAN_POINT('Ctrl Pts',(99.9591400986934,-0.757606432029038,
-2.07106419599434));
#26229=CARTESIAN_POINT('Ctrl Pts',(99.9632034608563,-0.686468212907689,
-2.09571506184319));
#26230=CARTESIAN_POINT('Ctrl Pts',(99.9672668230191,-0.614317465756464,
-2.11665539265761));
#26231=CARTESIAN_POINT('Ctrl Pts',(99.9713323105909,-0.542128978961985,
-2.13760667665888));
#26232=CARTESIAN_POINT('Ctrl Pts',(99.9753977981627,-0.468927374446688,
-2.15484345107275));
#26233=CARTESIAN_POINT('Ctrl Pts',(99.9794632857344,-0.395128183154033,
-2.16829188968584));
#26234=CARTESIAN_POINT('Ctrl Pts',(99.983536032225,-0.32119722357254,-2.1817643404556));
#26235=CARTESIAN_POINT('Ctrl Pts',(99.9876087787156,-0.246667019992794,
-2.19143488320763));
#26236=CARTESIAN_POINT('Ctrl Pts',(99.9916815252062,-0.171959035827759,
-2.19728152269963));
#26237=CARTESIAN_POINT('Ctrl Pts',(99.9948136488818,-0.114505264399459,
-2.20177784920008));
#26238=CARTESIAN_POINT('Ctrl Pts',(99.9979457725574,-0.0569464831372791,
-2.20401367458827));
#26239=CARTESIAN_POINT('Ctrl Pts',(100.001077896233,0.000526810878827148,
-2.20399993703954));
#26240=CARTESIAN_POINT('Ctrl Pts',(100.0051464063,0.0751824437715719,-2.20398209248387));
#26241=CARTESIAN_POINT('Ctrl Pts',(100.009214916367,0.14998309808274,-2.20016671252712));
#26242=CARTESIAN_POINT('Ctrl Pts',(100.013283426434,0.224509972218602,-2.19253535259398));
#26243=CARTESIAN_POINT('Ctrl Pts',(100.017345940743,0.298927016180346,-2.18491523898775));
#26244=CARTESIAN_POINT('Ctrl Pts',(100.021408455051,0.373070608838928,-2.17349035812419));
#26245=CARTESIAN_POINT('Ctrl Pts',(100.025470969359,0.446521919783342,-2.1582942744568));
#26246=CARTESIAN_POINT('Ctrl Pts',(100.029528729261,0.519887269822233,-2.14311597493915));
#26247=CARTESIAN_POINT('Ctrl Pts',(100.033586489162,0.592561481353539,-2.12417533700807));
#26248=CARTESIAN_POINT('Ctrl Pts',(100.037644249064,0.664132470250156,-2.1015575323934));
#26249=CARTESIAN_POINT('Ctrl Pts',(100.04169943528,0.735658064353487,-2.0789540734037));
#26250=CARTESIAN_POINT('Ctrl Pts',(100.045754621497,0.806081369022975,-2.052678219385));
#26251=CARTESIAN_POINT('Ctrl Pts',(100.049809807713,0.875003427246544,-2.0228655423203));
#26252=CARTESIAN_POINT('Ctrl Pts',(100.053863740074,0.943904174901207,-1.99306208327847));
#26253=CARTESIAN_POINT('Ctrl Pts',(100.057917672435,1.01130415862764,-1.95972416217078));
#26254=CARTESIAN_POINT('Ctrl Pts',(100.061971604796,1.07682397552376,-1.92303565378731));
#26255=CARTESIAN_POINT('Ctrl Pts',(100.066025601453,1.14234483158063,-1.8863465635149));
#26256=CARTESIAN_POINT('Ctrl Pts',(100.07007959811,1.20598504484707,-1.84630701587621));
#26257=CARTESIAN_POINT('Ctrl Pts',(100.074133594767,1.26739085804168,-1.80314625389966));
#26258=CARTESIAN_POINT('Ctrl Pts',(100.078191799491,1.32886041074648,-1.75994069085812));
#26259=CARTESIAN_POINT('Ctrl Pts',(100.082250004215,1.38809053945869,-1.71360771970359));
#26260=CARTESIAN_POINT('Ctrl Pts',(100.086308208939,1.44475811611921,-1.66441881325214));
#26261=CARTESIAN_POINT('Ctrl Pts',(100.090368560473,1.50145567020147,-1.61520388563161));
#26262=CARTESIAN_POINT('Ctrl Pts',(100.094428912007,1.55558762779912,-1.56313034662586));
#26263=CARTESIAN_POINT('Ctrl Pts',(100.09848926354,1.60686747152173,-1.50850685413271));
#26264=CARTESIAN_POINT('Ctrl Pts',(100.102556967611,1.65824017343895,-1.45378444872314));
#26265=CARTESIAN_POINT('Ctrl Pts',(100.106624671681,1.70675013601905,-1.39650323279177));
#26266=CARTESIAN_POINT('Ctrl Pts',(100.110692375751,1.75215120358949,-1.33700492136713));
#26267=CARTESIAN_POINT('Ctrl Pts',(100.113871121251,1.78763029370135,-1.2905094078142));
#26268=CARTESIAN_POINT('Ctrl Pts',(100.117049866752,1.82121165407053,-1.24266065374487));
#26269=CARTESIAN_POINT('Ctrl Pts',(100.120228612252,1.85279711796351,-1.19363262340894));
#26270=CARTESIAN_POINT('Ctrl Pts',(100.124309031285,1.89334202098052,-1.13069744722091));
#26271=CARTESIAN_POINT('Ctrl Pts',(100.128389450318,1.93075359612356,-1.0655746909329));
#26272=CARTESIAN_POINT('Ctrl Pts',(100.13246986935,1.96478922686938,-0.998608679102096));
#26273=CARTESIAN_POINT('Ctrl Pts',(100.136544285542,1.9987747866604,-0.931741183211151));
#26274=CARTESIAN_POINT('Ctrl Pts',(100.140618701734,2.02939404978258,-0.863036236644584));
#26275=CARTESIAN_POINT('Ctrl Pts',(100.144693117926,2.05644818337446,-0.792866236572012));
#26276=CARTESIAN_POINT('Ctrl Pts',(100.148762713041,2.08347030500095,-0.722779265571762));
#26277=CARTESIAN_POINT('Ctrl Pts',(100.152832308155,2.1069355090926,-0.651231127219556));
#26278=CARTESIAN_POINT('Ctrl Pts',(100.15690190327,2.12669204873535,-0.578616392652206));
#26279=CARTESIAN_POINT('Ctrl Pts',(100.160968878032,2.14643586743594,-0.50604841363288));
#26280=CARTESIAN_POINT('Ctrl Pts',(100.165035852795,2.16247563638747,-0.432415659130984));
#26281=CARTESIAN_POINT('Ctrl Pts',(100.169102827558,2.17470910480003,-0.358128900676611));
#26282=CARTESIAN_POINT('Ctrl Pts',(100.173168485386,2.1869386118692,-0.2838661971632));
#26283=CARTESIAN_POINT('Ctrl Pts',(100.177234143213,2.19536418859232,-0.208950379172764));
#26284=CARTESIAN_POINT('Ctrl Pts',(100.181299801041,2.19993478236944,-0.133801918226653));
#26285=CARTESIAN_POINT('Ctrl Pts',(100.185365443619,2.20450535900327,-0.0586537391457808));
#26286=CARTESIAN_POINT('Ctrl Pts',(100.189431086198,2.20522095433587,0.0167266063313277));
#26287=CARTESIAN_POINT('Ctrl Pts',(100.193496728776,2.2020825414925,0.0919156159416376));
#26288=CARTESIAN_POINT('Ctrl Pts',(100.197566376062,2.19894103727403,0.167178687647775));
#26289=CARTESIAN_POINT('Ctrl Pts',(100.201636023348,2.1919379634564,0.242249570886276));
#26290=CARTESIAN_POINT('Ctrl Pts',(100.205705670634,2.18112638065457,0.316707612179906));
#26291=CARTESIAN_POINT('Ctrl Pts',(100.209777369737,2.17030934691738,0.39120319339508));
#26292=CARTESIAN_POINT('Ctrl Pts',(100.213849068839,2.15568007182915,0.46508485016155));
#26293=CARTESIAN_POINT('Ctrl Pts',(100.217920767942,2.13734272129844,0.537942461340027));
#26294=CARTESIAN_POINT('Ctrl Pts',(100.221999535866,2.11897353554306,0.61092655962566));
#26295=CARTESIAN_POINT('Ctrl Pts',(100.22607830379,2.09688355492054,0.682882605652555));
#26296=CARTESIAN_POINT('Ctrl Pts',(100.230157071714,2.07122662006758,0.753416410972987));
#26297=CARTESIAN_POINT('Ctrl Pts',(100.233231157233,2.05188950323143,0.806576324352992));
#26298=CARTESIAN_POINT('Ctrl Pts',(100.236305242752,2.03052727456381,0.85892869107479));
#26299=CARTESIAN_POINT('Ctrl Pts',(100.239379328271,2.00722316170751,0.910313780575081));
#26300=CARTESIAN_POINT('Ctrl Pts',(100.243411081307,1.97665913634629,0.977706827817865));
#26301=CARTESIAN_POINT('Ctrl Pts',(100.247442834343,1.94263306376122,1.04369995973938));
#26302=CARTESIAN_POINT('Ctrl Pts',(100.25147458738,1.90529626114647,1.10790891198747));
#26303=CARTESIAN_POINT('Ctrl Pts',(100.25557233437,1.86734830918308,1.17316887172939));
#26304=CARTESIAN_POINT('Ctrl Pts',(100.259670081361,1.82598039289948,1.23658522006357));
#26305=CARTESIAN_POINT('Ctrl Pts',(100.263767828351,1.78140262335438,1.29777528621335));
#26306=CARTESIAN_POINT('Ctrl Pts',(100.267789135409,1.73765641361766,1.35782390450241));
#26307=CARTESIAN_POINT('Ctrl Pts',(100.271810442467,1.69081936945625,1.41572816748967));
#26308=CARTESIAN_POINT('Ctrl Pts',(100.275831749524,1.64113541697714,1.47115279394877));
#26309=CARTESIAN_POINT('Ctrl Pts',(100.279850713013,1.59148041970876,1.5265451196013));
#26310=CARTESIAN_POINT('Ctrl Pts',(100.283869676501,1.53898213005258,1.57946031247005));
#26311=CARTESIAN_POINT('Ctrl Pts',(100.28788863999,1.48392491646616,1.62959591380529));
#26312=CARTESIAN_POINT('Ctrl Pts',(100.291906624003,1.42888112105103,1.67971929643126));
#26313=CARTESIAN_POINT('Ctrl Pts',(100.295924608017,1.37128000066142,1.72706410412449));
#26314=CARTESIAN_POINT('Ctrl Pts',(100.299942592031,1.31144169603398,1.77136576626724));
#26315=CARTESIAN_POINT('Ctrl Pts',(100.304099085624,1.24954062102563,1.81719461333045));
#26316=CARTESIAN_POINT('Ctrl Pts',(100.308255579218,1.18524572013854,1.85976630705441));
#26317=CARTESIAN_POINT('Ctrl Pts',(100.312412072811,1.1189455096022,1.89883568181691));
#26318=CARTESIAN_POINT('Ctrl Pts',(100.316434556042,1.05478289775656,1.93664541285184));
#26319=CARTESIAN_POINT('Ctrl Pts',(100.320457039272,0.988742795484717,1.97117505493495));
#26320=CARTESIAN_POINT('Ctrl Pts',(100.324479522503,0.92120178309576,2.00224955358247));
#26321=CARTESIAN_POINT('Ctrl Pts',(100.328703021278,0.850285543869137,2.03487693807064));
#26322=CARTESIAN_POINT('Ctrl Pts',(100.332926520052,0.777715028177847,2.06369458611144));
#26323=CARTESIAN_POINT('Ctrl Pts',(100.337150018827,0.703946408049919,2.08855822389361));
#26324=CARTESIAN_POINT('Ctrl Pts',(100.341373517602,0.630177787921981,2.11342186167578));
#26325=CARTESIAN_POINT('Ctrl Pts',(100.345597016376,0.555211675809381,2.13433139831774));
#26326=CARTESIAN_POINT('Ctrl Pts',(100.349820515151,0.479516069206331,2.15120439274675));
#26327=CARTESIAN_POINT('',(100.349869898682,1.9893770426062,0.948680653513814));
#26328=CARTESIAN_POINT('Origin',(100.349869898682,0.,0.));
#26329=CARTESIAN_POINT('Ctrl Pts',(100.349869898682,1.9893770426062,0.948680653513815));
#26330=CARTESIAN_POINT('Ctrl Pts',(100.345705551524,2.02247380987769,0.879276951909368));
#26331=CARTESIAN_POINT('Ctrl Pts',(100.341541204365,2.05195987186717,0.808086644086603));
#26332=CARTESIAN_POINT('Ctrl Pts',(100.337376857207,2.07765243739774,0.735510944429262));
#26333=CARTESIAN_POINT('Ctrl Pts',(100.333215187647,2.10332848308289,0.662981909607237));
#26334=CARTESIAN_POINT('Ctrl Pts',(100.329053518087,2.12521573587352,0.589069675070232));
#26335=CARTESIAN_POINT('Ctrl Pts',(100.324891848527,2.1431798897202,0.514194477118237));
#26336=CARTESIAN_POINT('Ctrl Pts',(100.320730691219,2.16114183239345,0.439328495411571));
#26337=CARTESIAN_POINT('Ctrl Pts',(100.316569533911,2.17518152259502,0.363500217611781));
#26338=CARTESIAN_POINT('Ctrl Pts',(100.312408376603,2.18521504163324,0.287143207859524));
#26339=CARTESIAN_POINT('Ctrl Pts',(100.308247312157,2.19524833675862,0.210787902127007));
#26340=CARTESIAN_POINT('Ctrl Pts',(100.304086247711,2.20127557988319,0.133904330784247));
#26341=CARTESIAN_POINT('Ctrl Pts',(100.299925183266,2.20326454118416,0.0569329567170542));
#26342=CARTESIAN_POINT('Ctrl Pts',(100.295763137625,2.20525397148981,-0.0200565674943));
#26343=CARTESIAN_POINT('Ctrl Pts',(100.291601091984,2.20320321502967,-0.0971334889875312));
#26344=CARTESIAN_POINT('Ctrl Pts',(100.287439046344,2.19713218054514,-0.173856783626463));
#26345=CARTESIAN_POINT('Ctrl Pts',(100.28327494463,2.19105814693721,-0.250617979982078));
#26346=CARTESIAN_POINT('Ctrl Pts',(100.279110842917,2.18095992145872,-0.327024757020367));
#26347=CARTESIAN_POINT('Ctrl Pts',(100.274946741204,2.16690920950204,-0.40264187285382));
#26348=CARTESIAN_POINT('Ctrl Pts',(100.270776328819,2.15283720377383,-0.478373585982651));
#26349=CARTESIAN_POINT('Ctrl Pts',(100.266605916434,2.13480083408059,-0.55331280862868));
#26350=CARTESIAN_POINT('Ctrl Pts',(100.262435504048,2.11292277344509,-0.627035368585478));
#26351=CARTESIAN_POINT('Ctrl Pts',(100.258261651188,2.0910266640139,-0.700818747617783));
#26352=CARTESIAN_POINT('Ctrl Pts',(100.254087798328,2.06528269850951,-0.773383043315252));
#26353=CARTESIAN_POINT('Ctrl Pts',(100.249913945468,2.03586236903032,-0.844322458759825));
#26354=CARTESIAN_POINT('Ctrl Pts',(100.245732052254,2.00638536532792,-0.915398529243178));
#26355=CARTESIAN_POINT('Ctrl Pts',(100.24155015904,1.97321804347586,-0.984843063660913));
#26356=CARTESIAN_POINT('Ctrl Pts',(100.237368265825,1.93657857844273,-1.05227344807171));
#26357=CARTESIAN_POINT('Ctrl Pts',(100.235151904771,1.91716003301833,-1.08801086895061));
#26358=CARTESIAN_POINT('Ctrl Pts',(100.232935543717,1.89676694883971,-1.12318300253146));
#26359=CARTESIAN_POINT('Ctrl Pts',(100.230719182663,1.87543663427232,-1.15773633908128));
#26360=CARTESIAN_POINT('Ctrl Pts',(100.226681843158,1.83658117725961,-1.22067894964221));
#26361=CARTESIAN_POINT('Ctrl Pts',(100.222644503653,1.79446431510442,-1.28180751700185));
#26362=CARTESIAN_POINT('Ctrl Pts',(100.218607164148,1.74928100490527,-1.3407579818437));
#26363=CARTESIAN_POINT('Ctrl Pts',(100.214576367462,1.70417091773602,-1.39961291292253));
#26364=CARTESIAN_POINT('Ctrl Pts',(100.210545570776,1.65600453538297,-1.45629636238109));
#26365=CARTESIAN_POINT('Ctrl Pts',(100.20651477409,1.60502159852659,-1.51047067772372));
#26366=CARTESIAN_POINT('Ctrl Pts',(100.202489410823,1.55410738546927,-1.5645719673642));
#26367=CARTESIAN_POINT('Ctrl Pts',(100.198464047556,1.50038448930946,-1.6161704872544));
#26368=CARTESIAN_POINT('Ctrl Pts',(100.194438684289,1.44413353989373,-1.66496075598015));
#26369=CARTESIAN_POINT('Ctrl Pts',(100.190416300267,1.38792422282207,-1.71371491414644));
#26370=CARTESIAN_POINT('Ctrl Pts',(100.186393916244,1.32919092952845,-1.75966462457535));
#26371=CARTESIAN_POINT('Ctrl Pts',(100.182371532221,1.26825084872205,-1.80254147933295));
#26372=CARTESIAN_POINT('Ctrl Pts',(100.178350765927,1.20733527689301,-1.84540108980979));
#26373=CARTESIAN_POINT('Ctrl Pts',(100.174329999633,1.14421507644506,-1.88519001645548));
#26374=CARTESIAN_POINT('Ctrl Pts',(100.170309233339,1.07923881312582,-1.92168144712977));
#26375=CARTESIAN_POINT('Ctrl Pts',(100.166288725414,1.01426672509177,-1.95817053291498));
#26376=CARTESIAN_POINT('Ctrl Pts',(100.162268217489,0.947439236549497,-1.99136230620485));
#26377=CARTESIAN_POINT('Ctrl Pts',(100.158247709563,0.879130542096939,-2.02107533010335));
#26378=CARTESIAN_POINT('Ctrl Pts',(100.154223272099,0.810755084507366,-2.05081739473672));
#26379=CARTESIAN_POINT('Ctrl Pts',(100.150198834634,0.740895977443084,-2.07707372443632));
#26380=CARTESIAN_POINT('Ctrl Pts',(100.146174397169,0.66994767428634,-2.09971095956523));
#26381=CARTESIAN_POINT('Ctrl Pts',(100.142148026805,0.598965295331431,-2.12235906714381));
#26382=CARTESIAN_POINT('Ctrl Pts',(100.138121656441,0.526893150576154,-2.14138449574319));
#26383=CARTESIAN_POINT('Ctrl Pts',(100.134095286077,0.454138437003612,-2.15670449529738));
#26384=CARTESIAN_POINT('Ctrl Pts',(100.130061528505,0.38125023988055,-2.17205260255531));
#26385=CARTESIAN_POINT('Ctrl Pts',(100.126027770933,0.307677454727682,-2.18368162615086));
#26386=CARTESIAN_POINT('Ctrl Pts',(100.121994013361,0.233834487177226,-2.19156050169886));
#26387=CARTESIAN_POINT('Ctrl Pts',(100.118518831122,0.170216938348896,-2.19834834848393));
#26388=CARTESIAN_POINT('Ctrl Pts',(100.115043648883,0.106399111850957,-2.20235359730959));
#26389=CARTESIAN_POINT('Ctrl Pts',(100.111568466644,0.0426447683184777,
-2.20358739870582));
#26390=CARTESIAN_POINT('Ctrl Pts',(100.107492140298,-0.0321379314998587,
-2.20503462558225));
#26391=CARTESIAN_POINT('Ctrl Pts',(100.103415813953,-0.107137919792663,
-2.20267349357564));
#26392=CARTESIAN_POINT('Ctrl Pts',(100.099339487607,-0.181935437885235,
-2.19647797540552));
#26393=CARTESIAN_POINT('Ctrl Pts',(100.095269175343,-0.256622602116876,
-2.19029159790433));
#26394=CARTESIAN_POINT('Ctrl Pts',(100.091198863078,-0.331107418229155,
-2.1802821054808));
#26395=CARTESIAN_POINT('Ctrl Pts',(100.087128550814,-0.404969172531764,
-2.16647547165874));
#26396=CARTESIAN_POINT('Ctrl Pts',(100.083063058635,-0.478743459358434,
-2.15268518772469));
#26397=CARTESIAN_POINT('Ctrl Pts',(100.078997566455,-0.55189568428568,-2.13510678388212));
#26398=CARTESIAN_POINT('Ctrl Pts',(100.074932074276,-0.624010943631892,
-2.11381795389945));
#26399=CARTESIAN_POINT('Ctrl Pts',(100.070869199899,-0.696079767387687,
-2.09254283196412));
#26400=CARTESIAN_POINT('Ctrl Pts',(100.066806325523,-0.767112494745006,
-2.06756215981608));
#26401=CARTESIAN_POINT('Ctrl Pts',(100.062743451146,-0.836706396294933,
-2.03900426836217));
#26402=CARTESIAN_POINT('Ctrl Pts',(100.058681885859,-0.906277874164999,
-2.01045557847623));
#26403=CARTESIAN_POINT('Ctrl Pts',(100.054620320571,-0.974411006142448,
-1.97833213865823));
#26404=CARTESIAN_POINT('Ctrl Pts',(100.050558755283,-1.04072167636616,-1.9428109512615));
#26405=CARTESIAN_POINT('Ctrl Pts',(100.046497192096,-1.10703231230171,-1.90728978223219));
#26406=CARTESIAN_POINT('Ctrl Pts',(100.042435628908,-1.17152006911247,-1.86837109573711));
#26407=CARTESIAN_POINT('Ctrl Pts',(100.038374065721,-1.23382556728059,-1.82627776351921));
#26408=CARTESIAN_POINT('Ctrl Pts',(100.034308450996,-1.296193217134,-1.78414244188442));
#26409=CARTESIAN_POINT('Ctrl Pts',(100.030242836272,-1.35637386531743,-1.73882641771799));
#26410=CARTESIAN_POINT('Ctrl Pts',(100.026177221548,-1.41403790925473,-1.69059539547182));
#26411=CARTESIAN_POINT('Ctrl Pts',(100.022109535129,-1.47173133677111,-1.64233979638436));
#26412=CARTESIAN_POINT('Ctrl Pts',(100.01804184871,-1.52690525613829,-1.59116656516457));
#26413=CARTESIAN_POINT('Ctrl Pts',(100.013974162291,-1.57926588176533,-1.53737935288984));
#26414=CARTESIAN_POINT('Ctrl Pts',(100.00989933106,-1.63171847781615,-1.48349766441954));
#26415=CARTESIAN_POINT('Ctrl Pts',(100.005824499829,-1.68134759452345,-1.42699318221482));
#26416=CARTESIAN_POINT('Ctrl Pts',(100.001749668597,-1.72789910523482,-1.36820345056161));
#26417=CARTESIAN_POINT('Ctrl Pts',(99.9986390292732,-1.76343553646106,-1.32332462227489));
#26418=CARTESIAN_POINT('Ctrl Pts',(99.9955283899492,-1.79717931958817,-1.27711478052259));
#26419=CARTESIAN_POINT('Ctrl Pts',(99.9924177506252,-1.82903497614255,-1.22973454698451));
#26420=CARTESIAN_POINT('Ctrl Pts',(99.9883380320037,-1.87081484892997,-1.16759361680217));
#26421=CARTESIAN_POINT('Ctrl Pts',(99.9842583133821,-1.9095019130363,-1.1032056749545));
#26422=CARTESIAN_POINT('Ctrl Pts',(99.9801785947606,-1.94484752698673,-1.03691084321343));
#26423=CARTESIAN_POINT('Ctrl Pts',(99.9761047238386,-1.98014247800006,-0.97071103573465));
#26424=CARTESIAN_POINT('Ctrl Pts',(99.9720308529165,-2.01210526712443,-0.902610182078885));
#26425=CARTESIAN_POINT('Ctrl Pts',(99.9679569819944,-2.0405305570293,-0.832977218073647));
#26426=CARTESIAN_POINT('Ctrl Pts',(99.9638876981338,-2.06892384087561,-0.763422658782331));
#26427=CARTESIAN_POINT('Ctrl Pts',(99.9598184142732,-2.09378736062871,-0.692339855024764));
#26428=CARTESIAN_POINT('Ctrl Pts',(99.9557491304126,-2.1149624750193,-0.62012073764731));
#26429=CARTESIAN_POINT('Ctrl Pts',(99.9516823233637,-2.13612470095763,-0.547945577182193));
#26430=CARTESIAN_POINT('Ctrl Pts',(99.9476155163147,-2.15360284351699,-0.474635931076114));
#26431=CARTESIAN_POINT('Ctrl Pts',(99.9435487092658,-2.16728748085921,-0.400600767985965));
#26432=CARTESIAN_POINT('Ctrl Pts',(99.9394830758517,-2.18096816896875,-0.326586970612548));
#26433=CARTESIAN_POINT('Ctrl Pts',(99.9354174424376,-2.19085743937203,-0.251848539451298));
#26434=CARTESIAN_POINT('Ctrl Pts',(99.9313518090235,-2.19689689986293,-0.176805009467076));
#26435=CARTESIAN_POINT('Ctrl Pts',(99.9272860476566,-2.20293655042664,-0.101759117726364));
#26436=CARTESIAN_POINT('Ctrl Pts',(99.9232202862896,-2.20512611409972,-0.0264085823242432));
#26437=CARTESIAN_POINT('Ctrl Pts',(99.9191545249226,-2.2034591668547,0.0488231502875364));
#26438=CARTESIAN_POINT('Ctrl Pts',(99.9150845382916,-2.20179048726689,0.124133066027335));
#26439=CARTESIAN_POINT('Ctrl Pts',(99.9110145516604,-2.19625730423869,0.199323455888921));
#26440=CARTESIAN_POINT('Ctrl Pts',(99.9069445650293,-2.18690532399787,0.273972815932136));
#26441=CARTESIAN_POINT('Ctrl Pts',(99.9028724035345,-2.17754834637388,0.348662066078422));
#26442=CARTESIAN_POINT('Ctrl Pts',(99.8988002420397,-2.16436859091822,0.422809241954582));
#26443=CARTESIAN_POINT('Ctrl Pts',(99.8947280805448,-2.14746303997753,0.496002512020312));
#26444=CARTESIAN_POINT('Ctrl Pts',(99.8906486544299,-2.13052733001547,0.569326356795161));
#26445=CARTESIAN_POINT('Ctrl Pts',(99.8865692283149,-2.10985267906245,0.641692438675049));
#26446=CARTESIAN_POINT('Ctrl Pts',(99.8824898021999,-2.08558601042208,0.712704001063348));
#26447=CARTESIAN_POINT('Ctrl Pts',(99.8794155463353,-2.06729864688573,0.766218320475076));
#26448=CARTESIAN_POINT('Ctrl Pts',(99.8763412904706,-2.04697237237334,0.818963707625186));
#26449=CARTESIAN_POINT('Ctrl Pts',(99.8732670346059,-2.02468756933049,0.870779103216547));
#26450=CARTESIAN_POINT('Ctrl Pts',(99.8691983003044,-1.9951939466352,0.939356048879436));
#26451=CARTESIAN_POINT('Ctrl Pts',(99.865129566003,-1.9621542300046,1.00656781621544));
#26452=CARTESIAN_POINT('Ctrl Pts',(99.8610608317015,-1.92571655130637,1.07202227776511));
#26453=CARTESIAN_POINT('Ctrl Pts',(99.8569981432433,-1.8893330163485,1.13737947874556));
#26454=CARTESIAN_POINT('Ctrl Pts',(99.8529354547851,-1.84956177394102,1.20098414327725));
#26455=CARTESIAN_POINT('Ctrl Pts',(99.8488727663269,-1.80659876662032,1.26246461195787));
#26456=CARTESIAN_POINT('Ctrl Pts',(99.8448149078923,-1.76368683689073,1.32387198812388));
#26457=CARTESIAN_POINT('Ctrl Pts',(99.8407570494577,-1.71759095361078,1.38315979527332));
#26458=CARTESIAN_POINT('Ctrl Pts',(99.8366991910231,-1.66855182652232,1.43998291733237));
#26459=CARTESIAN_POINT('Ctrl Pts',(99.8326439525906,-1.61954436209969,1.49676935090138));
#26460=CARTESIAN_POINT('Ctrl Pts',(99.8285887141581,-1.56759773647102,1.55109389558607));
#26461=CARTESIAN_POINT('Ctrl Pts',(99.8245334757256,-1.51299380749293,1.60264335973043));
#26462=CARTESIAN_POINT('Ctrl Pts',(99.8204795373842,-1.45840738428668,1.65417629735053));
#26463=CARTESIAN_POINT('Ctrl Pts',(99.8164255990427,-1.40116569683704,1.70293559234757));
#26464=CARTESIAN_POINT('Ctrl Pts',(99.8123716607012,-1.34158729132383,1.74864505825465));
#26465=CARTESIAN_POINT('Ctrl Pts',(99.8083177042632,-1.28200861985567,1.79435472820643));
#26466=CARTESIAN_POINT('Ctrl Pts',(99.8042637478252,-1.22009359045887,1.83701425211435));
#26467=CARTESIAN_POINT('Ctrl Pts',(99.8002097913871,-1.1561923405857,1.87638889134714));
#26468=CARTESIAN_POINT('Ctrl Pts',(99.7961516982078,-1.09222588455107,1.91580370927892));
#26469=CARTESIAN_POINT('Ctrl Pts',(99.7920936050285,-1.02626956904168,1.9519266971401));
#26470=CARTESIAN_POINT('Ctrl Pts',(99.7880355118492,-0.958700267890422,
1.98456791174977));
#26471=CARTESIAN_POINT('Ctrl Pts',(99.7839753115554,-0.891095882218119,
2.01722607490502));
#26472=CARTESIAN_POINT('Ctrl Pts',(99.7799151112615,-0.82187728464676,2.04639867878928));
#26473=CARTESIAN_POINT('Ctrl Pts',(99.7758549109677,-0.75144110058728,2.07194408041052));
#26474=CARTESIAN_POINT('Ctrl Pts',(99.7717874216498,-0.680878466843862,
2.09753534209649));
#26475=CARTESIAN_POINT('Ctrl Pts',(99.7677199323318,-0.609094338978657,
2.11948625489022));
#26476=CARTESIAN_POINT('Ctrl Pts',(99.7636524430139,-0.536499815403239,
2.13770529963143));
#26477=CARTESIAN_POINT('Ctrl Pts',(99.7604737348715,-0.479767815601417,
2.15194332740185));
#26478=CARTESIAN_POINT('Ctrl Pts',(99.7572950267292,-0.422541202822639,
2.16390320940677));
#26479=CARTESIAN_POINT('Ctrl Pts',(99.7541163185868,-0.365018595209633,
2.17356330139041));
#26480=CARTESIAN_POINT('Ctrl Pts',(99.7474958281946,-0.245212732581249,
2.19368296739992));
#26481=CARTESIAN_POINT('Ctrl Pts',(99.7408753378023,-0.123701771398941,
2.20390030207451));
#26482=CARTESIAN_POINT('Ctrl Pts',(99.7342548474101,-0.00178926204916046,
2.20399927371615));
#26483=CARTESIAN_POINT('Origin',(25.4947388265965,0.,-6.40787078036307));
#26484=CARTESIAN_POINT('',(25.4947388265965,-7.48009298981943E-16,6.107959450045));
#26485=CARTESIAN_POINT('Origin',(25.4947388265965,0.,0.));
#26486=CARTESIAN_POINT('',(25.4947388265965,-7.47987577963046E-16,6.10778208446569));
#26487=CARTESIAN_POINT('Origin',(25.4947388265965,0.,0.));
#26488=CARTESIAN_POINT('Origin',(27.4542764744824,0.,0.));
#26489=CARTESIAN_POINT('',(27.7542764744824,-7.48069377062962E-16,6.10845002480549));
#26490=CARTESIAN_POINT('Origin',(27.7542764744824,0.,0.));
#26491=CARTESIAN_POINT('',(27.4541877916966,-7.84808779432149E-16,6.40845001169777));
#26492=CARTESIAN_POINT('Origin',(27.4542764744824,-7.48069377062961E-16,
6.10845002480549));
#26493=CARTESIAN_POINT('Origin',(27.4541877916966,-7.84808779432149E-16,
0.));
#26494=CARTESIAN_POINT('Origin',(26.6245076505395,0.,0.));
#26495=CARTESIAN_POINT('',(25.7946501438108,-7.8474870135113E-16,6.40795943693727));
#26496=CARTESIAN_POINT('',(26.6245076505395,-7.84778743602106E-16,6.40820475053297));
#26497=CARTESIAN_POINT('Origin',(25.7946501438108,-7.8474870135113E-16,
0.));
#26498=CARTESIAN_POINT('Origin',(25.7947388265966,0.,0.));
#26499=CARTESIAN_POINT('Origin',(25.7947388265966,-7.48009298981944E-16,
6.107959450045));
#26500=CARTESIAN_POINT('Origin',(27.7542764744824,0.,-6.40853872070288));
#26501=CARTESIAN_POINT('',(27.7542764744824,-7.4809109808186E-16,6.1086273903848));
#26502=CARTESIAN_POINT('Origin',(27.7542764744824,0.,0.));
#26503=CARTESIAN_POINT('Ctrl Pts',(90.0988178106407,1.30236646373779,-1.19759169991716));
#26504=CARTESIAN_POINT('Ctrl Pts',(90.1385586184198,1.70110773626567,-0.764007006172047));
#26505=CARTESIAN_POINT('Ctrl Pts',(90.2180163315385,2.02395293608162,0.525231536151233));
#26506=CARTESIAN_POINT('Ctrl Pts',(90.3371909499971,0.652775565002029,1.98853514061584));
#26507=CARTESIAN_POINT('Ctrl Pts',(90.4563416660163,-1.31672770966033,1.62464706040724));
#26508=CARTESIAN_POINT('Ctrl Pts',(90.5754923820352,-2.07940182116321,-0.225715520989952));
#26509=CARTESIAN_POINT('Ctrl Pts',(90.6946430980545,-0.936716819385667,
-1.87038353007312));
#26510=CARTESIAN_POINT('Ctrl Pts',(90.8137938140736,1.06439707893563,-1.80053599719708));
#26511=CARTESIAN_POINT('Ctrl Pts',(90.9329445300927,2.09011102819176,-0.0810387888271981));
#26512=CARTESIAN_POINT('Ctrl Pts',(91.052095246112,1.20054819198944,1.71286342585472));
#26513=CARTESIAN_POINT('Ctrl Pts',(91.171245962131,-0.789155321291253,1.93709542934556));
#26514=CARTESIAN_POINT('Ctrl Pts',(91.2903966781501,-2.05570548030766,0.386289109614587));
#26515=CARTESIAN_POINT('Ctrl Pts',(91.4095473941693,-1.43849345547043,-1.51851496410962));
#26516=CARTESIAN_POINT('Ctrl Pts',(91.5286981101884,0.496895874116886,-2.03180509569764));
#26517=CARTESIAN_POINT('Ctrl Pts',(91.6478488262076,1.97694974251289,-0.683237063999725));
#26518=CARTESIAN_POINT('Ctrl Pts',(91.7669995422267,1.6454082772736,1.29142367419714));
#26519=CARTESIAN_POINT('Ctrl Pts',(91.8861502582457,-0.193917899418074,
2.0826756182632));
#26520=CARTESIAN_POINT('Ctrl Pts',(92.005300974265,-1.85554561362532,0.965449717325565));
#26521=CARTESIAN_POINT('Ctrl Pts',(92.1244516902841,-1.81682754149423,-1.03647495873235));
#26522=CARTESIAN_POINT('Ctrl Pts',(92.2436024063033,-0.113243288550902,
-2.08861639028052));
#26523=CARTESIAN_POINT('Ctrl Pts',(92.3627531223225,1.69411245684142,-1.22683558804683));
#26524=CARTESIAN_POINT('Ctrl Pts',(92.4819038383415,1.94905310597792,0.759167013834017));
#26525=CARTESIAN_POINT('Ctrl Pts',(92.6010545543606,0.417961509270532,2.04950011481713));
#26526=CARTESIAN_POINT('Ctrl Pts',(92.7202052703798,-1.49613285327444,1.46175546640634));
#26527=CARTESIAN_POINT('Ctrl Pts',(92.8393559863988,-2.03923249641387,-0.465481880699497));
#26528=CARTESIAN_POINT('Ctrl Pts',(92.958506702418,-0.713663204520452,-1.96617074130422));
#26529=CARTESIAN_POINT('Ctrl Pts',(93.0776574184373,1.26587774694564,-1.66514146098521));
#26530=CARTESIAN_POINT('Ctrl Pts',(93.1968081344563,2.08542030441444,0.161755088931124));
#26531=CARTESIAN_POINT('Ctrl Pts',(93.3159588504756,0.993969316150796,1.84042591624436));
#26532=CARTESIAN_POINT('Ctrl Pts',(93.4351095664945,-1.00831434394197,1.83260599657131));
#26533=CARTESIAN_POINT('Ctrl Pts',(93.5542602825138,-2.0866201376949,0.145461183012646));
#26534=CARTESIAN_POINT('Ctrl Pts',(93.6734109985329,-1.25283290778611,-1.67497828640997));
#26535=CARTESIAN_POINT('Ctrl Pts',(93.7925617145521,0.728998961157423,-1.96053642389964));
#26536=CARTESIAN_POINT('Ctrl Pts',(93.9117124305713,2.04280611266453,-0.449539476415141));
#26537=CARTESIAN_POINT('Ctrl Pts',(94.0308631465901,1.48466961417535,1.47339699047405));
#26538=CARTESIAN_POINT('Ctrl Pts',(94.1500138626095,-0.433957162547644,
2.04617294867045));
#26539=CARTESIAN_POINT('Ctrl Pts',(94.2691645786286,-1.95492341252519,0.743920026586493));
#26540=CARTESIAN_POINT('Ctrl Pts',(94.3883152946477,-1.68447811070772,-1.24003066467813));
#26541=CARTESIAN_POINT('Ctrl Pts',(94.5074660106668,0.129553772013031,-2.0876681668678));
#26542=CARTESIAN_POINT('Ctrl Pts',(94.6266167266861,1.82486789716038,-1.0222522744945));
#26543=CARTESIAN_POINT('Ctrl Pts',(94.7457674427052,1.84794800509362,0.97991363153406));
#26544=CARTESIAN_POINT('Ctrl Pts',(94.8649181587243,0.177644432504533,2.08412691801531));
#26545=CARTESIAN_POINT('Ctrl Pts',(94.9840688747434,-1.65544520447039,1.27853186498882));
#26546=CARTESIAN_POINT('Ctrl Pts',(95.1032195907626,-1.97155282381159,-0.698657296330842));
#26547=CARTESIAN_POINT('Ctrl Pts',(95.2223703067817,-0.48101038161002,-2.03562559612007));
#26548=CARTESIAN_POINT('Ctrl Pts',(95.3415210228009,1.4503102254182,-1.50723017646382));
#26549=CARTESIAN_POINT('Ctrl Pts',(95.4606717388199,2.05262608737329,0.402329094436875));
#26550=CARTESIAN_POINT('Ctrl Pts',(95.5798224548391,0.773999677688958,1.94321050165266));
#26551=CARTESIAN_POINT('Ctrl Pts',(95.6989731708583,-1.21388825846436,1.70341358769916));
#26552=CARTESIAN_POINT('Ctrl Pts',(95.8181238868774,-2.0894188332659,-0.0973216008372093));
#26553=CARTESIAN_POINT('Ctrl Pts',(95.9372746028964,-1.05029177469469,-1.80887527010699));
#26554=CARTESIAN_POINT('Ctrl Pts',(96.0564253189157,0.951279544295426,-1.86284990898372));
#26555=CARTESIAN_POINT('Ctrl Pts',(96.1755760349347,2.0811373456516,-0.209785374442143));
#26556=CARTESIAN_POINT('Ctrl Pts',(96.294726750954,1.30392632887128,1.63551786406429));
#26557=CARTESIAN_POINT('Ctrl Pts',(96.4138774669731,-0.668149240282063,
1.98209968152566));
#26558=CARTESIAN_POINT('Ctrl Pts',(96.5330281829921,-2.02796027789557,0.512366730060481));
#26559=CARTESIAN_POINT('Ctrl Pts',(96.6521788990114,-1.52943177897067,-1.42687805655579));
#26560=CARTESIAN_POINT('Ctrl Pts',(96.7713296150304,0.370605208206405,-2.05859037557912));
#26561=CARTESIAN_POINT('Ctrl Pts',(96.8904803310495,1.93103479854338,-0.803894994145272));
#26562=CARTESIAN_POINT('Ctrl Pts',(97.0096310470688,1.72194338215499,1.18745675437928));
#26563=CARTESIAN_POINT('Ctrl Pts',(97.1287817630879,-0.065066251703002,
2.0906718866246));
#26564=CARTESIAN_POINT('Ctrl Pts',(97.247932479107,-1.7924518438776,1.07808113898674));
#26565=CARTESIAN_POINT('Ctrl Pts',(97.3670831951263,-1.87730815926342,-0.922418901837522));
#26566=CARTESIAN_POINT('Ctrl Pts',(97.4862339111451,-0.241876354077899,
-2.07765213228422));
#26567=CARTESIAN_POINT('Ctrl Pts',(97.6053846271646,1.61520101083011,-1.32901025214378));
#26568=CARTESIAN_POINT('Ctrl Pts',(97.7245353431835,1.9921744856802,0.637482059999133));
#26569=CARTESIAN_POINT('Ctrl Pts',(97.8436860592028,0.54360105305752,2.01981198109672));
#26570=CARTESIAN_POINT('Ctrl Pts',(97.9628367752219,-1.4031060626124,1.55126913908458));
#26571=CARTESIAN_POINT('Ctrl Pts',(98.081987491241,-2.06406439651977,-0.338793068912289));
#26572=CARTESIAN_POINT('Ctrl Pts',(98.2011382072602,-0.833598848803122,
-1.91839918354454));
#26573=CARTESIAN_POINT('Ctrl Pts',(98.3202889232793,1.16074243271934,-1.74006311968733));
#26574=CARTESIAN_POINT('Ctrl Pts',(98.4394396392984,2.09142705758357,0.032795483461962));
#26575=CARTESIAN_POINT('Ctrl Pts',(98.5585903553176,1.10561369120534,1.77560137656009));
#26576=CARTESIAN_POINT('Ctrl Pts',(98.6777410713367,-0.893338462267605,
1.891319617894));
#26577=CARTESIAN_POINT('Ctrl Pts',(98.7968917873559,-2.07367233759831,0.27390912055697));
#26578=CARTESIAN_POINT('Ctrl Pts',(98.9160425033749,-1.35377720344853,-1.59449827219737));
#26579=CARTESIAN_POINT('Ctrl Pts',(99.0351932193941,0.606662148098891,-2.00177724927629));
#26580=CARTESIAN_POINT('Ctrl Pts',(99.1543439354132,2.01118446085511,-0.574701107001492));
#26581=CARTESIAN_POINT('Ctrl Pts',(99.2734946514324,1.57273344194911,1.37899033502367));
#26582=CARTESIAN_POINT('Ctrl Pts',(99.3926453674515,-0.306893054534305,
2.06906590760142));
#26583=CARTESIAN_POINT('Ctrl Pts',(99.5117960834707,-1.90532100320877,0.863066202672188));
#26584=CARTESIAN_POINT('Ctrl Pts',(99.6309467994897,-1.75773992851836,-1.13367603950222));
#26585=CARTESIAN_POINT('Ctrl Pts',(99.750097515509,0.000460101095811506,
-2.09183477779575));
#26586=CARTESIAN_POINT('Ctrl Pts',(99.869248231528,1.75844121890259,-1.13258284903887));
#26587=CARTESIAN_POINT('Ctrl Pts',(99.9883989475472,1.90465462099256,0.863446991429658));
#26588=CARTESIAN_POINT('Ctrl Pts',(100.107549663566,0.306334449084961,2.07039782385695));
#26589=CARTESIAN_POINT('Ctrl Pts',(100.226715227927,-1.57465064547374,1.37565407054423));
#26590=CARTESIAN_POINT('Ctrl Pts',(100.30616388695,-1.86309197916195,0.0785106641831038));
#26591=CARTESIAN_POINT('Ctrl Pts',(100.345895640631,-1.70077331743764,-0.487600721360894));
#26592=CARTESIAN_POINT('Ctrl Pts',(90.1836630036807,1.41054030214643,-1.29706300437212));
#26593=CARTESIAN_POINT('Ctrl Pts',(90.2234038114599,1.84240080430918,-0.827465005690515));
#26594=CARTESIAN_POINT('Ctrl Pts',(90.3028615245785,2.19206134792296,0.568856977147052));
#26595=CARTESIAN_POINT('Ctrl Pts',(90.422036143037,0.706994742516013,2.15370176994804));
#26596=CARTESIAN_POINT('Ctrl Pts',(90.5411868590562,-1.42609438521506,1.75958934698854));
#26597=CARTESIAN_POINT('Ctrl Pts',(90.6603375750753,-2.25211578674213,-0.244463327366812));
#26598=CARTESIAN_POINT('Ctrl Pts',(90.7794882910944,-1.01452000049959,-2.02573655195885));
#26599=CARTESIAN_POINT('Ctrl Pts',(90.8986390071135,1.15280531181421,-1.95008752162037));
#26600=CARTESIAN_POINT('Ctrl Pts',(91.0177897231328,2.26371449458543,-0.0877698258214138));
#26601=CARTESIAN_POINT('Ctrl Pts',(91.1369404391518,1.30026506104129,1.85513291497586));
#26602=CARTESIAN_POINT('Ctrl Pts',(91.2560911551711,-0.854702125959167,
2.09798950470033));
#26603=CARTESIAN_POINT('Ctrl Pts',(91.3752418711901,-2.22645124091666,0.418374069482609));
#26604=CARTESIAN_POINT('Ctrl Pts',(91.4943925872093,-1.55797392654873,-1.64464197745212));
#26605=CARTESIAN_POINT('Ctrl Pts',(91.6135433032284,0.538167770690726,-2.20056570357529));
#26606=CARTESIAN_POINT('Ctrl Pts',(91.7326940192475,2.14115409508415,-0.739986356778505));
#26607=CARTESIAN_POINT('Ctrl Pts',(91.8518447352668,1.78207497904909,1.39868861055673));
#26608=CARTESIAN_POINT('Ctrl Pts',(91.9709954512857,-0.210024612927857,
2.25566150361919));
#26609=CARTESIAN_POINT('Ctrl Pts',(92.090146167305,-2.00966620637468,1.04563943705615));
#26610=CARTESIAN_POINT('Ctrl Pts',(92.209296883324,-1.96773223257935,-1.1225639957448));
#26611=CARTESIAN_POINT('Ctrl Pts',(92.3284475993433,-0.122649213486525,
-2.26209571287564));
#26612=CARTESIAN_POINT('Ctrl Pts',(92.4475983153624,1.8348245008436,-1.32873587368108));
#26613=CARTESIAN_POINT('Ctrl Pts',(92.5667490313815,2.11094037934247,0.822223006264858));
#26614=CARTESIAN_POINT('Ctrl Pts',(92.6858997474007,0.452677161142528,2.21973046119938));
#26615=CARTESIAN_POINT('Ctrl Pts',(92.8050504634197,-1.62040082086588,1.58316806725156));
#26616=CARTESIAN_POINT('Ctrl Pts',(92.924201179439,-2.20861002008845,-0.504144548348667));
#26617=CARTESIAN_POINT('Ctrl Pts',(93.043351895458,-0.772939675708481,-2.12947979599473));
#26618=CARTESIAN_POINT('Ctrl Pts',(93.1625026114772,1.37102085271187,-1.80344719008944));
#26619=CARTESIAN_POINT('Ctrl Pts',(93.2816533274963,2.25863416188464,0.175190377184455));
#26620=CARTESIAN_POINT('Ctrl Pts',(93.4008040435155,1.07652785799153,1.99329067528883));
#26621=CARTESIAN_POINT('Ctrl Pts',(93.5199547595345,-1.09206437585973,1.98482123741135));
#26622=CARTESIAN_POINT('Ctrl Pts',(93.6391054755538,-2.25993365265399,0.157543108449209));
#26623=CARTESIAN_POINT('Ctrl Pts',(93.7582561915729,-1.35689251642417,-1.81410105679525));
#26624=CARTESIAN_POINT('Ctrl Pts',(93.8774069075921,0.789549211812653,-2.1233774953017));
#26625=CARTESIAN_POINT('Ctrl Pts',(93.996557623611,2.21248045892906,-0.486877976778926));
#26626=CARTESIAN_POINT('Ctrl Pts',(94.1157083396304,1.60798545146521,1.5957765298718));
#26627=CARTESIAN_POINT('Ctrl Pts',(94.2348590556494,-0.470001404536919,
2.21612694247214));
#26628=CARTESIAN_POINT('Ctrl Pts',(94.3540097716686,-2.11729827030588,0.805709612686535));
#26629=CARTESIAN_POINT('Ctrl Pts',(94.4731604876876,-1.8243899312468,-1.34302692608189));
#26630=CARTESIAN_POINT('Ctrl Pts',(94.5923112037068,0.140314436687032,-2.26106873055054));
#26631=CARTESIAN_POINT('Ctrl Pts',(94.711461919726,1.97644041574166,-1.10715998321782));
#26632=CARTESIAN_POINT('Ctrl Pts',(94.8306126357451,2.00143754467901,1.06130471598179));
#26633=CARTESIAN_POINT('Ctrl Pts',(94.9497633517643,0.192399480849997,2.25723334752628));
#26634=CARTESIAN_POINT('Ctrl Pts',(95.0689140677833,-1.79294556786947,1.38472601480337));
#26635=CARTESIAN_POINT('Ctrl Pts',(95.1880647838026,-2.13530891129945,-0.756687385081276));
#26636=CARTESIAN_POINT('Ctrl Pts',(95.3072154998216,-0.520962837959247,
-2.20470353265046));
#26637=CARTESIAN_POINT('Ctrl Pts',(95.4263662158408,1.57077219087492,-1.63241988158377));
#26638=CARTESIAN_POINT('Ctrl Pts',(95.5455169318599,2.22311607530774,0.435746326575808));
#26639=CARTESIAN_POINT('Ctrl Pts',(95.6646676478791,0.838287662978745,2.10461249153227));
#26640=CARTESIAN_POINT('Ctrl Pts',(95.7838183638982,-1.31471314606197,1.84489817848784));
#26641=CARTESIAN_POINT('Ctrl Pts',(95.9029690799174,-2.26296480633173,-0.105405079194289));
#26642=CARTESIAN_POINT('Ctrl Pts',(96.0221197959364,-1.13752842880178,-1.95911944992743));
#26643=CARTESIAN_POINT('Ctrl Pts',(96.1412705119557,1.0302922972887,-2.01757719246707));
#26644=CARTESIAN_POINT('Ctrl Pts',(96.2604212279747,2.25399546293495,-0.227210031654438));
#26645=CARTESIAN_POINT('Ctrl Pts',(96.3795719439939,1.41222972881548,1.77136307358693));
#26646=CARTESIAN_POINT('Ctrl Pts',(96.498722660013,-0.723645346764778,2.14673178518397));
#26647=CARTESIAN_POINT('Ctrl Pts',(96.6178733760322,-2.19640153733235,0.554923627375294));
#26648=CARTESIAN_POINT('Ctrl Pts',(96.7370240920512,-1.65646553691972,-1.54539375902228));
#26649=CARTESIAN_POINT('Ctrl Pts',(96.8561748080704,0.401387471894955,-2.22957575399431));
#26650=CARTESIAN_POINT('Ctrl Pts',(96.9753255240896,2.0914254812546,-0.870666067891006));
#26651=CARTESIAN_POINT('Ctrl Pts',(97.0944762401087,1.86496704742619,1.28608625586138));
#26652=CARTESIAN_POINT('Ctrl Pts',(97.2136269561279,-0.0704706185947552,
2.26432193760961));
#26653=CARTESIAN_POINT('Ctrl Pts',(97.332777672147,-1.94133190299583,1.16762596232738));
#26654=CARTESIAN_POINT('Ctrl Pts',(97.4519283881662,-2.03323633702113,-0.999034505825096));
#26655=CARTESIAN_POINT('Ctrl Pts',(97.5710791041852,-0.261966470315861,
-2.25022076967224));
#26656=CARTESIAN_POINT('Ctrl Pts',(97.6902298202045,1.74935871375617,-1.43939710888626));
#26657=CARTESIAN_POINT('Ctrl Pts',(97.8093805362235,2.15764339700129,0.69043096744322));
#26658=CARTESIAN_POINT('Ctrl Pts',(97.9285312522427,0.588752255971226,2.18757644750652));
#26659=CARTESIAN_POINT('Ctrl Pts',(98.0476819682618,-1.51964727640531,1.68011669609097));
#26660=CARTESIAN_POINT('Ctrl Pts',(98.166832684281,-2.23550444408775,-0.366933033899782));
#26661=CARTESIAN_POINT('Ctrl Pts',(98.2859834003001,-0.902837108293679,
-2.07774035906009));
#26662=CARTESIAN_POINT('Ctrl Pts',(98.4051341163192,1.25715305741451,-1.88459180033968));
#26663=CARTESIAN_POINT('Ctrl Pts',(98.5242848323384,2.26513983265089,0.0355194581859003));
#26664=CARTESIAN_POINT('Ctrl Pts',(98.6434355483575,1.1974453531107,1.92308184517942));
#26665=CARTESIAN_POINT('Ctrl Pts',(98.7625862643768,-0.967538661022872,
2.04841157965873));
#26666=CARTESIAN_POINT('Ctrl Pts',(98.8817369803958,-2.24591041544012,0.296659860667986));
#26667=CARTESIAN_POINT('Ctrl Pts',(99.000887696415,-1.46622118947291,-1.72693641709899));
#26668=CARTESIAN_POINT('Ctrl Pts',(99.1200384124339,0.657051170700659,-2.16804376083236));
#26669=CARTESIAN_POINT('Ctrl Pts',(99.2391891284533,2.17823233020374,-0.622435463200776));
#26670=CARTESIAN_POINT('Ctrl Pts',(99.3583398444722,1.70336381208397,1.49352850981649));
#26671=CARTESIAN_POINT('Ctrl Pts',(99.4774905604915,-0.33238342196486,2.24092137791455));
#26672=CARTESIAN_POINT('Ctrl Pts',(99.5966412765106,-2.06357591229645,0.934752004282814));
#26673=CARTESIAN_POINT('Ctrl Pts',(99.7157919925298,-1.90373683513884,-1.22783854454161));
#26674=CARTESIAN_POINT('Ctrl Pts',(99.8349427085489,0.00049831683842665,
-2.26558141787846));
#26675=CARTESIAN_POINT('Ctrl Pts',(99.9540934245681,1.90449637431464,-1.22665455428283));
#26676=CARTESIAN_POINT('Ctrl Pts',(100.073244140587,2.06285418074182,0.935164421143912));
#26677=CARTESIAN_POINT('Ctrl Pts',(100.192394856606,0.331778419055773,2.24236392239785));
#26678=CARTESIAN_POINT('Ctrl Pts',(100.311560420967,-1.70544025747331,1.48991513705402));
#26679=CARTESIAN_POINT('Ctrl Pts',(100.39100907999,-2.01783936886045,0.0850317165421618));
#26680=CARTESIAN_POINT('Ctrl Pts',(100.430740833671,-1.84203860883819,-0.528100567686047));
#26681=CARTESIAN_POINT('Ctrl Pts',(90.2685081967207,1.51871414055506,-1.39653430882706));
#26682=CARTESIAN_POINT('Ctrl Pts',(90.3082490044998,1.98369387235267,-0.890923005208982));
#26683=CARTESIAN_POINT('Ctrl Pts',(90.3877067176185,2.36016975976431,0.612482418142867));
#26684=CARTESIAN_POINT('Ctrl Pts',(90.5068813360772,0.761213920029996,2.31886839928025));
#26685=CARTESIAN_POINT('Ctrl Pts',(90.626032052096,-1.53546106076978,1.89453163356984));
#26686=CARTESIAN_POINT('Ctrl Pts',(90.7451827681155,-2.42482975232106,-0.263211133743666));
#26687=CARTESIAN_POINT('Ctrl Pts',(90.8643334841343,-1.09232318161353,-2.18108957384459));
#26688=CARTESIAN_POINT('Ctrl Pts',(90.9834842001537,1.24121354469281,-2.09963904604366));
#26689=CARTESIAN_POINT('Ctrl Pts',(91.1026349161728,2.43731796097908,-0.0945008628156303));
#26690=CARTESIAN_POINT('Ctrl Pts',(91.2217856321918,1.39998193009314,1.99740240409698));
#26691=CARTESIAN_POINT('Ctrl Pts',(91.3409363482112,-0.920248930627077,
2.2588835800551));
#26692=CARTESIAN_POINT('Ctrl Pts',(91.4600870642302,-2.39719700152565,0.450459029350631));
#26693=CARTESIAN_POINT('Ctrl Pts',(91.5792377802492,-1.67745439762702,-1.77076899079462));
#26694=CARTESIAN_POINT('Ctrl Pts',(91.6983884962685,0.57943966726456,-2.36932631145295));
#26695=CARTESIAN_POINT('Ctrl Pts',(91.8175392122875,2.30535844765541,-0.796735649557284));
#26696=CARTESIAN_POINT('Ctrl Pts',(91.9366899283068,1.91874168082458,1.5059535469163));
#26697=CARTESIAN_POINT('Ctrl Pts',(92.0558406443258,-0.22613132643764,2.42864738897517));
#26698=CARTESIAN_POINT('Ctrl Pts',(92.174991360345,-2.16378679912404,1.12582915678676));
#26699=CARTESIAN_POINT('Ctrl Pts',(92.2941420763643,-2.11863692366447,-1.20865303275725));
#26700=CARTESIAN_POINT('Ctrl Pts',(92.4132927923833,-0.132055138422147,
-2.43557503547077));
#26701=CARTESIAN_POINT('Ctrl Pts',(92.5324435084023,1.97553654484576,-1.43063615931535));
#26702=CARTESIAN_POINT('Ctrl Pts',(92.6515942244216,2.272827652707,0.8852789986957));
#26703=CARTESIAN_POINT('Ctrl Pts',(92.7707449404406,0.487392813014522,2.38996080758163));
#26704=CARTESIAN_POINT('Ctrl Pts',(92.88989565646,-1.74466878845731,1.70458066809679));
#26705=CARTESIAN_POINT('Ctrl Pts',(93.0090463724789,-2.37798754376304,-0.542807215997835));
#26706=CARTESIAN_POINT('Ctrl Pts',(93.128197088498,-0.832216146896508,-2.29278885068523));
#26707=CARTESIAN_POINT('Ctrl Pts',(93.2473478045172,1.4761639584781,-1.94175291919367));
#26708=CARTESIAN_POINT('Ctrl Pts',(93.3664985205364,2.43184801935483,0.188625665437788));
#26709=CARTESIAN_POINT('Ctrl Pts',(93.4856492365556,1.15908639983226,2.14615543433331));
#26710=CARTESIAN_POINT('Ctrl Pts',(93.6047999525747,-1.17581440777752,2.13703647825138));
#26711=CARTESIAN_POINT('Ctrl Pts',(93.7239506685937,-2.43324716761307,0.169625033885773));
#26712=CARTESIAN_POINT('Ctrl Pts',(93.8431013846129,-1.46095212506224,-1.95322382718053));
#26713=CARTESIAN_POINT('Ctrl Pts',(93.9622521006321,0.850099462467886,-2.28621856670378));
#26714=CARTESIAN_POINT('Ctrl Pts',(94.081402816651,2.38215480519359,-0.524216477142713));
#26715=CARTESIAN_POINT('Ctrl Pts',(94.2005535326705,1.73130128875504,1.71815606926955));
#26716=CARTESIAN_POINT('Ctrl Pts',(94.3197042486894,-0.506045646526193,
2.38608093627382));
#26717=CARTESIAN_POINT('Ctrl Pts',(94.4388549647086,-2.27967312808658,0.867499198786582));
#26718=CARTESIAN_POINT('Ctrl Pts',(94.5580056807278,-1.96430175178589,-1.44602318748566));
#26719=CARTESIAN_POINT('Ctrl Pts',(94.6771563967469,0.151075101361031,-2.43446929423327));
#26720=CARTESIAN_POINT('Ctrl Pts',(94.796307112766,2.12801293432294,-1.19206769194113));
#26721=CARTESIAN_POINT('Ctrl Pts',(94.9154578287851,2.15492708426441,1.14269580042952));
#26722=CARTESIAN_POINT('Ctrl Pts',(95.0346085448042,0.207154529195459,2.43033977703725));
#26723=CARTESIAN_POINT('Ctrl Pts',(95.1537592608234,-1.93044593126855,1.49092016461792));
#26724=CARTESIAN_POINT('Ctrl Pts',(95.2729099768426,-2.29906499878732,-0.814717473831705));
#26725=CARTESIAN_POINT('Ctrl Pts',(95.3920606928618,-0.560915294308474,
-2.37378146918088));
#26726=CARTESIAN_POINT('Ctrl Pts',(95.5112114088808,1.69123415633164,-1.75760958670372));
#26727=CARTESIAN_POINT('Ctrl Pts',(95.6303621249,2.39360606324219,0.469163558714741));
#26728=CARTESIAN_POINT('Ctrl Pts',(95.749512840919,0.90257564826853,2.26601448141187));
#26729=CARTESIAN_POINT('Ctrl Pts',(95.8686635569383,-1.41553803365958,1.98638276927655));
#26730=CARTESIAN_POINT('Ctrl Pts',(95.9878142729574,-2.43651077939756,-0.113488557551372));
#26731=CARTESIAN_POINT('Ctrl Pts',(96.1069649889766,-1.22476508290887,-2.10936362974787));
#26732=CARTESIAN_POINT('Ctrl Pts',(96.2261157049957,1.10930505028198,-2.17230447595042));
#26733=CARTESIAN_POINT('Ctrl Pts',(96.3452664210148,2.42685358021832,-0.244634688866736));
#26734=CARTESIAN_POINT('Ctrl Pts',(96.4644171370341,1.52053312875968,1.90720828310958));
#26735=CARTESIAN_POINT('Ctrl Pts',(96.5835678530531,-0.77914145324749,2.31136388884227));
#26736=CARTESIAN_POINT('Ctrl Pts',(96.7027185690724,-2.36484279676913,0.597480524690107));
#26737=CARTESIAN_POINT('Ctrl Pts',(96.8218692850914,-1.78349929486876,-1.66390946148877));
#26738=CARTESIAN_POINT('Ctrl Pts',(96.9410200011106,0.432169735583501,-2.40056113240953));
#26739=CARTESIAN_POINT('Ctrl Pts',(97.0601707171294,2.2518161639658,-0.937437141636736));
#26740=CARTESIAN_POINT('Ctrl Pts',(97.1793214331488,2.00799071269739,1.38471575734347));
#26741=CARTESIAN_POINT('Ctrl Pts',(97.2984721491679,-0.0758749854865103,
2.4379719885946));
#26742=CARTESIAN_POINT('Ctrl Pts',(97.417622865187,-2.09021196211405,1.25717078566802));
#26743=CARTESIAN_POINT('Ctrl Pts',(97.5367735812062,-2.18916451477885,-1.07565010981266));
#26744=CARTESIAN_POINT('Ctrl Pts',(97.6559242972254,-0.282056586553822,
-2.42278940706025));
#26745=CARTESIAN_POINT('Ctrl Pts',(97.7750750132444,1.88351641668224,-1.54978396562876));
#26746=CARTESIAN_POINT('Ctrl Pts',(97.8942257292636,2.32311230832238,0.743379874887306));
#26747=CARTESIAN_POINT('Ctrl Pts',(98.0133764452828,0.633903458884932,2.35534091391632));
#26748=CARTESIAN_POINT('Ctrl Pts',(98.1325271613019,-1.63618849019823,1.80896425309736));
#26749=CARTESIAN_POINT('Ctrl Pts',(98.2516778773212,-2.40694449165574,-0.395072998887273));
#26750=CARTESIAN_POINT('Ctrl Pts',(98.3708285933402,-0.972075367784237,
-2.23708153457564));
#26751=CARTESIAN_POINT('Ctrl Pts',(98.4899793093593,1.3535636821097,-2.02912048099205));
#26752=CARTESIAN_POINT('Ctrl Pts',(98.6091300253786,2.4388526077182,0.0382434329098399));
#26753=CARTESIAN_POINT('Ctrl Pts',(98.7282807413975,1.28927701501606,2.07056231379875));
#26754=CARTESIAN_POINT('Ctrl Pts',(98.8474314574167,-1.04173885977815,2.20550354142346));
#26755=CARTESIAN_POINT('Ctrl Pts',(98.966582173436,-2.41814849328193,0.319410600779003));
#26756=CARTESIAN_POINT('Ctrl Pts',(99.0857328894549,-1.5786651754973,-1.85937456200061));
#26757=CARTESIAN_POINT('Ctrl Pts',(99.2048836054743,0.707440193302429,-2.33431027238844));
#26758=CARTESIAN_POINT('Ctrl Pts',(99.3240343214933,2.34528019955236,-0.670169819400066));
#26759=CARTESIAN_POINT('Ctrl Pts',(99.4431850375124,1.8339941822188,1.60806668460931));
#26760=CARTESIAN_POINT('Ctrl Pts',(99.5623357535317,-0.357873789395414,
2.41277684822769));
#26761=CARTESIAN_POINT('Ctrl Pts',(99.6814864695508,-2.22183082138415,1.00643780589344));
#26762=CARTESIAN_POINT('Ctrl Pts',(99.8006371855698,-2.04973374175933,-1.322001049581));
#26763=CARTESIAN_POINT('Ctrl Pts',(99.9197879015891,0.000536532581040912,
-2.43932805796117));
#26764=CARTESIAN_POINT('Ctrl Pts',(100.038938617608,2.05055152972668,-1.32072625952678));
#26765=CARTESIAN_POINT('Ctrl Pts',(100.158089333627,2.22105374049109,1.00688185085817));
#26766=CARTESIAN_POINT('Ctrl Pts',(100.277240049646,0.357222389026584,2.41433002093876));
#26767=CARTESIAN_POINT('Ctrl Pts',(100.396405614007,-1.83622986947288,1.6041762035638));
#26768=CARTESIAN_POINT('Ctrl Pts',(100.47585427303,-2.17258675855896,0.0915527689012232));
#26769=CARTESIAN_POINT('Ctrl Pts',(100.515586026711,-1.98330390023875,-0.568600414011198));
#26770=CARTESIAN_POINT('Ctrl Pts',(90.3533533897608,1.6268879789637,-1.49600561328201));
#26771=CARTESIAN_POINT('Ctrl Pts',(90.3930941975399,2.12498694039619,-0.954381004727451));
#26772=CARTESIAN_POINT('Ctrl Pts',(90.4725519106586,2.52827817160566,0.656107859138686));
#26773=CARTESIAN_POINT('Ctrl Pts',(90.5917265291171,0.81543309754398,2.48403502861246));
#26774=CARTESIAN_POINT('Ctrl Pts',(90.7108772451363,-1.64482773632451,2.02947392015113));
#26775=CARTESIAN_POINT('Ctrl Pts',(90.8300279611553,-2.59754371789998,-0.281958940120525));
#26776=CARTESIAN_POINT('Ctrl Pts',(90.9491786771745,-1.17012636272745,-2.33644259573031));
#26777=CARTESIAN_POINT('Ctrl Pts',(91.0683293931936,1.3296217775714,-2.24919057046694));
#26778=CARTESIAN_POINT('Ctrl Pts',(91.1874801092128,2.61092142737275,-0.101231899809847));
#26779=CARTESIAN_POINT('Ctrl Pts',(91.306630825232,1.499698799145,2.1396718932181));
#26780=CARTESIAN_POINT('Ctrl Pts',(91.4257815412509,-0.985795735294989,
2.41977765540987));
#26781=CARTESIAN_POINT('Ctrl Pts',(91.5449322572702,-2.56794276213465,0.482543989218656));
#26782=CARTESIAN_POINT('Ctrl Pts',(91.6640829732894,-1.79693486870532,-1.89689600413712));
#26783=CARTESIAN_POINT('Ctrl Pts',(91.7832336893085,0.620711563838398,-2.53808691933059));
#26784=CARTESIAN_POINT('Ctrl Pts',(91.9023844053276,2.46956280022668,-0.853484942336065));
#26785=CARTESIAN_POINT('Ctrl Pts',(92.0215351213467,2.05540838260006,1.61321848327588));
#26786=CARTESIAN_POINT('Ctrl Pts',(92.1406858373659,-0.242238039947421,
2.60163327433116));
#26787=CARTESIAN_POINT('Ctrl Pts',(92.2598365533851,-2.3179073918734,1.20601887651735));
#26788=CARTESIAN_POINT('Ctrl Pts',(92.3789872694042,-2.26954161474959,-1.2947420697697));
#26789=CARTESIAN_POINT('Ctrl Pts',(92.4981379854234,-0.141461063357769,
-2.6090543580659));
#26790=CARTESIAN_POINT('Ctrl Pts',(92.6172887014424,2.11624858884793,-1.53253644494961));
#26791=CARTESIAN_POINT('Ctrl Pts',(92.7364394174617,2.43471492607153,0.94833499112654));
#26792=CARTESIAN_POINT('Ctrl Pts',(92.8555901334807,0.522108464886517,2.56019115396389));
#26793=CARTESIAN_POINT('Ctrl Pts',(92.9747408494998,-1.86893675604876,1.82599326894201));
#26794=CARTESIAN_POINT('Ctrl Pts',(93.093891565519,-2.54736506743762,-0.581469883647004));
#26795=CARTESIAN_POINT('Ctrl Pts',(93.2130422815382,-0.891492618084537,
-2.45609790537574));
#26796=CARTESIAN_POINT('Ctrl Pts',(93.3321929975572,1.58130706424433,-2.08005864829791));
#26797=CARTESIAN_POINT('Ctrl Pts',(93.4513437135765,2.60506187682501,0.20206095369112));
#26798=CARTESIAN_POINT('Ctrl Pts',(93.5704944295954,1.24164494167299,2.29902019337778));
#26799=CARTESIAN_POINT('Ctrl Pts',(93.6896451456148,-1.25956443969529,2.2892517190914));
#26800=CARTESIAN_POINT('Ctrl Pts',(93.8087958616338,-2.60656068257214,0.181706959322336));
#26801=CARTESIAN_POINT('Ctrl Pts',(93.9279465776529,-1.5650117337003,-2.09234659756582));
#26802=CARTESIAN_POINT('Ctrl Pts',(94.0470972936722,0.910649713123118,-2.44905963810584));
#26803=CARTESIAN_POINT('Ctrl Pts',(94.1662480096911,2.55182915145811,-0.561554977506499));
#26804=CARTESIAN_POINT('Ctrl Pts',(94.2853987257105,1.85461712604488,1.8405356086673));
#26805=CARTESIAN_POINT('Ctrl Pts',(94.4045494417295,-0.542089888515468,
2.5560349300755));
#26806=CARTESIAN_POINT('Ctrl Pts',(94.5237001577486,-2.44204798586726,0.929288784886628));
#26807=CARTESIAN_POINT('Ctrl Pts',(94.6428508737678,-2.10421357232497,-1.54901944888943));
#26808=CARTESIAN_POINT('Ctrl Pts',(94.7620015897869,0.161835766035032,-2.60786985791601));
#26809=CARTESIAN_POINT('Ctrl Pts',(94.881152305806,2.27958545290423,-1.27697540066444));
#26810=CARTESIAN_POINT('Ctrl Pts',(95.0003030218252,2.30841662384981,1.22408688487725));
#26811=CARTESIAN_POINT('Ctrl Pts',(95.1194537378444,0.221909577540923,2.60344620654823));
#26812=CARTESIAN_POINT('Ctrl Pts',(95.2386044538635,-2.06794629466763,1.59711431443246));
#26813=CARTESIAN_POINT('Ctrl Pts',(95.3577551698827,-2.46282108627517,-0.872747562582139));
#26814=CARTESIAN_POINT('Ctrl Pts',(95.4769058859017,-0.6008677506577,-2.54285940571127));
#26815=CARTESIAN_POINT('Ctrl Pts',(95.596056601921,1.81169612178837,-1.88279929182366));
#26816=CARTESIAN_POINT('Ctrl Pts',(95.71520731794,2.56409605117663,0.502580790853675));
#26817=CARTESIAN_POINT('Ctrl Pts',(95.8343580339592,0.966863633558315,2.42741647129147));
#26818=CARTESIAN_POINT('Ctrl Pts',(95.9535087499783,-1.51636292125719,2.12786736006524));
#26819=CARTESIAN_POINT('Ctrl Pts',(96.0726594659974,-2.61005675246339,-0.121572035908453));
#26820=CARTESIAN_POINT('Ctrl Pts',(96.1918101820166,-1.31200173701596,-2.25960780956831));
#26821=CARTESIAN_POINT('Ctrl Pts',(96.3109608980357,1.18831780327526,-2.32703175943377));
#26822=CARTESIAN_POINT('Ctrl Pts',(96.4301116140548,2.59971169750167,-0.262059346079031));
#26823=CARTESIAN_POINT('Ctrl Pts',(96.549262330074,1.62883652870388,2.04305349263221));
#26824=CARTESIAN_POINT('Ctrl Pts',(96.6684130460932,-0.834637559730204,
2.47599599250058));
#26825=CARTESIAN_POINT('Ctrl Pts',(96.7875637621122,-2.5332840562059,0.640037422004922));
#26826=CARTESIAN_POINT('Ctrl Pts',(96.9067144781315,-1.91053305281782,-1.78242516395526));
#26827=CARTESIAN_POINT('Ctrl Pts',(97.0258651941505,0.462951999272051,-2.57154651082474));
#26828=CARTESIAN_POINT('Ctrl Pts',(97.1450159101697,2.41220684667701,-1.00420821538247));
#26829=CARTESIAN_POINT('Ctrl Pts',(97.2641666261889,2.15101437796858,1.48334525882557));
#26830=CARTESIAN_POINT('Ctrl Pts',(97.383317342208,-0.0812793523782635,
2.61162203957959));
#26831=CARTESIAN_POINT('Ctrl Pts',(97.5024680582271,-2.23909202123227,1.34671560900866));
#26832=CARTESIAN_POINT('Ctrl Pts',(97.6216187742462,-2.34509269253657,-1.15226571380024));
#26833=CARTESIAN_POINT('Ctrl Pts',(97.7407694902653,-0.302146702791784,
-2.59535804444827));
#26834=CARTESIAN_POINT('Ctrl Pts',(97.8599202062845,2.0176741196083,-1.66017082237124));
#26835=CARTESIAN_POINT('Ctrl Pts',(97.9790709223037,2.48858121964347,0.796328782331391));
#26836=CARTESIAN_POINT('Ctrl Pts',(98.0982216383227,0.679054661798639,2.52310538032613));
#26837=CARTESIAN_POINT('Ctrl Pts',(98.217372354342,-1.75272970399117,1.93781181010375));
#26838=CARTESIAN_POINT('Ctrl Pts',(98.3365230703609,-2.57838453922373,-0.423212963874765));
#26839=CARTESIAN_POINT('Ctrl Pts',(98.4556737863803,-1.0413136272748,-2.39642271009119));
#26840=CARTESIAN_POINT('Ctrl Pts',(98.5748245023993,1.44997430680488,-2.17364916164441));
#26841=CARTESIAN_POINT('Ctrl Pts',(98.6939752184185,2.61256538278553,0.040967407633777));
#26842=CARTESIAN_POINT('Ctrl Pts',(98.8131259344376,1.38110867692141,2.2180427824181));
#26843=CARTESIAN_POINT('Ctrl Pts',(98.9322766504567,-1.11593905853341,2.3625955031882));
#26844=CARTESIAN_POINT('Ctrl Pts',(99.0514273664759,-2.59038657112374,0.342161340890021));
#26845=CARTESIAN_POINT('Ctrl Pts',(99.1705780824951,-1.69110916152168,-1.99181270690224));
#26846=CARTESIAN_POINT('Ctrl Pts',(99.289728798514,0.757829215904196,-2.50057678394453));
#26847=CARTESIAN_POINT('Ctrl Pts',(99.4088795145334,2.512328068901,-0.717904175599352));
#26848=CARTESIAN_POINT('Ctrl Pts',(99.5280302305524,1.96462455235365,1.72260485940214));
#26849=CARTESIAN_POINT('Ctrl Pts',(99.6471809465717,-0.383364156825967,
2.58463231854081));
#26850=CARTESIAN_POINT('Ctrl Pts',(99.7663316625907,-2.38008573047184,1.07812360750406));
#26851=CARTESIAN_POINT('Ctrl Pts',(99.8854823786097,-2.19573064837981,-1.41616355462039));
#26852=CARTESIAN_POINT('Ctrl Pts',(100.004633094629,0.000574748323657545,
-2.6130746980439));
#26853=CARTESIAN_POINT('Ctrl Pts',(100.123783810648,2.19660668513872,-1.41479796477074));
#26854=CARTESIAN_POINT('Ctrl Pts',(100.242934526667,2.37925330024036,1.07859928057243));
#26855=CARTESIAN_POINT('Ctrl Pts',(100.362085242686,0.382666358997397,2.58629611947964));
#26856=CARTESIAN_POINT('Ctrl Pts',(100.481250807047,-1.96701948147245,1.71843727007359));
#26857=CARTESIAN_POINT('Ctrl Pts',(100.56069946607,-2.32733414825746,0.0980738212602812));
#26858=CARTESIAN_POINT('Ctrl Pts',(100.600431219751,-2.12456919163931,-0.60910026033635));
#26859=CARTESIAN_POINT('Ctrl Pts',(100.349869898682,0.479414994925324,2.1549256777474));
#26860=CARTESIAN_POINT('Ctrl Pts',(100.349869898682,0.426652918711037,2.16183856744932));
#26861=CARTESIAN_POINT('Ctrl Pts',(100.349869898682,0.373742092670596,2.16669187525473));
#26862=CARTESIAN_POINT('Ctrl Pts',(100.349869898682,0.320765011501736,2.16941984999731));
#26863=CARTESIAN_POINT('Ctrl Pts',(100.349869898682,0.243016014546236,2.17342341711117));
#26864=CARTESIAN_POINT('Ctrl Pts',(100.349869898682,0.16512364757463,2.17285169457014));
#26865=CARTESIAN_POINT('Ctrl Pts',(100.349869898682,0.0874187569404108,
2.16789484102443));
#26866=CARTESIAN_POINT('Ctrl Pts',(100.349869898682,0.00882392242687584,
2.16288121728784));
#26867=CARTESIAN_POINT('Ctrl Pts',(100.349869898682,-0.0695801139311062,
2.15338096217544));
#26868=CARTESIAN_POINT('Ctrl Pts',(100.349869898682,-0.147434733898743,
2.13954043576136));
#26869=CARTESIAN_POINT('Ctrl Pts',(100.349869898682,-0.214042289617913,
2.12769934483199));
#26870=CARTESIAN_POINT('Ctrl Pts',(100.349869898682,-0.280247772641109,
2.11268039048099));
#26871=CARTESIAN_POINT('Ctrl Pts',(100.349869898682,-0.345809014350907,
2.09455055013332));
#26872=CARTESIAN_POINT('Ctrl Pts',(100.349869898682,-0.357788807056817,
2.09123774330581));
#26873=CARTESIAN_POINT('Ctrl Pts',(100.349869898682,-0.369741677068303,
2.08782245032927));
#26874=CARTESIAN_POINT('Ctrl Pts',(100.349869898682,-0.381659087973601,
2.08430749424));
#26875=CARTESIAN_POINT('Ctrl Pts',(100.349869898682,-0.455832594990877,
2.06243054275909));
#26876=CARTESIAN_POINT('Ctrl Pts',(100.349869898682,-0.528720372073745,
2.03667310778326));
#26877=CARTESIAN_POINT('Ctrl Pts',(100.349869898682,-0.599998286829302,
2.00720683896365));
#26878=CARTESIAN_POINT('Ctrl Pts',(100.349869898682,-0.671071640285958,
1.97782513572434));
#26879=CARTESIAN_POINT('Ctrl Pts',(100.349869898682,-0.740545253992376,
1.94475525166359));
#26880=CARTESIAN_POINT('Ctrl Pts',(100.349869898682,-0.808069062003364,
1.90812458173475));
#26881=CARTESIAN_POINT('Ctrl Pts',(100.349869898682,-0.875592870014457,
1.87149391180587));
#26882=CARTESIAN_POINT('Ctrl Pts',(100.349869898682,-0.941167756180382,
1.83130189692078));
#26883=CARTESIAN_POINT('Ctrl Pts',(100.349869898682,-1.00440156213989,1.78764176103565));
#26884=CARTESIAN_POINT('Ctrl Pts',(100.349869898682,-1.02779687561389,1.77148833566688));
#26885=CARTESIAN_POINT('Ctrl Pts',(100.349869898682,-1.05087124668116,1.75485987879234));
#26886=CARTESIAN_POINT('Ctrl Pts',(100.349869898682,-1.07360298298091,1.73776016033232));
#26887=CARTESIAN_POINT('Ctrl Pts',(100.349869898682,-1.0834417566988,1.7303590424261));
#26888=CARTESIAN_POINT('Ctrl Pts',(100.349869898682,-1.09320813055685,1.72287579541146));
#26889=CARTESIAN_POINT('Ctrl Pts',(100.349869898682,-1.10289990339264,1.71531171169829));
#26890=CARTESIAN_POINT('Ctrl Pts',(100.349869898682,-1.16103677703682,1.66993795124006));
#26891=CARTESIAN_POINT('Ctrl Pts',(100.349869898682,-1.21650251586315,1.62165059602811));
#26892=CARTESIAN_POINT('Ctrl Pts',(100.349869898682,-1.26898476694497,1.57056955339216));
#26893=CARTESIAN_POINT('Ctrl Pts',(100.349869898682,-1.31991541650645,1.52099868651621));
#26894=CARTESIAN_POINT('Ctrl Pts',(100.349869898682,-1.36803686624987,1.46879626023262));
#26895=CARTESIAN_POINT('Ctrl Pts',(100.349869898682,-1.41302321718474,1.41404528417547));
#26896=CARTESIAN_POINT('Ctrl Pts',(100.349869898682,-1.44122551234148,1.37972146917835));
#26897=CARTESIAN_POINT('Ctrl Pts',(100.349869898682,-1.46819484166188,1.34439554635872));
#26898=CARTESIAN_POINT('Ctrl Pts',(100.349869898682,-1.49384116343081,1.30808394627531));
#26899=CARTESIAN_POINT('Ctrl Pts',(100.349869898682,-1.52549362611721,1.26326849175988));
#26900=CARTESIAN_POINT('Ctrl Pts',(100.349869898682,-1.55513111765511,1.21695133144359));
#26901=CARTESIAN_POINT('Ctrl Pts',(100.349869898682,-1.58271301197475,1.16927838686888));
#26902=CARTESIAN_POINT('Ctrl Pts',(100.349869898682,-1.58818639734863,1.1598181085232));
#26903=CARTESIAN_POINT('Ctrl Pts',(100.349869898682,-1.59357707452801,1.15030730513006));
#26904=CARTESIAN_POINT('Ctrl Pts',(100.349869898682,-1.59888102457638,1.14075431016912));
#26905=CARTESIAN_POINT('Ctrl Pts',(100.349869898682,-1.63352381179593,1.07835885607847));
#26906=CARTESIAN_POINT('Ctrl Pts',(100.349869898682,-1.66452248560294,1.01407626558591));
#26907=CARTESIAN_POINT('Ctrl Pts',(100.349869898682,-1.69186815495425,0.948254794830066));
#26908=CARTESIAN_POINT('Ctrl Pts',(100.349869898682,-1.71949907167233,0.881746729024396));
#26909=CARTESIAN_POINT('Ctrl Pts',(100.349869898682,-1.74340046296127,0.813666407870188));
#26910=CARTESIAN_POINT('Ctrl Pts',(100.349869898682,-1.76351145671393,0.744362695339321));
#26911=CARTESIAN_POINT('Ctrl Pts',(100.349869898682,-1.77818378696145,0.693800949354107));
#26912=CARTESIAN_POINT('Ctrl Pts',(100.349869898682,-1.79083752897198,0.642587752401212));
#26913=CARTESIAN_POINT('Ctrl Pts',(100.349869898682,-1.80143159096359,0.590860235567238));
#26914=CARTESIAN_POINT('Ctrl Pts',(100.349869898682,-1.80788893402656,0.559331033429622));
#26915=CARTESIAN_POINT('Ctrl Pts',(100.349869898682,-1.81358077732524,0.527610800354061));
#26916=CARTESIAN_POINT('Ctrl Pts',(100.349869898682,-1.81849513035551,0.495731460558721));
#26917=CARTESIAN_POINT('Ctrl Pts',(100.349869898682,-1.82044661710907,0.483072193115095));
#26918=CARTESIAN_POINT('Ctrl Pts',(100.349869898682,-1.82227577945532,0.470385589327665));
#26919=CARTESIAN_POINT('Ctrl Pts',(100.349869898682,-1.82398080210445,0.457681045001183));
#26920=CARTESIAN_POINT('Ctrl Pts',(100.349869898682,-1.83331587288179,0.388123130012532));
#26921=CARTESIAN_POINT('Ctrl Pts',(100.349869898682,-1.83891415246051,0.31818414360954));
#26922=CARTESIAN_POINT('Ctrl Pts',(100.349869898682,-1.84071131029445,0.248192856326947));
#26923=CARTESIAN_POINT('Ctrl Pts',(100.349869898682,-1.84233496365043,0.184958795110429));
#26924=CARTESIAN_POINT('Ctrl Pts',(100.349869898682,-1.84085536620104,0.121681523396419));
#26925=CARTESIAN_POINT('Ctrl Pts',(100.349869898682,-1.83619001506015,0.0586141186189469));
#26926=CARTESIAN_POINT('Ctrl Pts',(100.349869898682,-1.83446389372265,0.0352799708132087));
#26927=CARTESIAN_POINT('Ctrl Pts',(100.349869898682,-1.83230134629309,0.0119746999217672));
#26928=CARTESIAN_POINT('Ctrl Pts',(100.349869898682,-1.82969704876538,-0.0112882622057083));
#26929=CARTESIAN_POINT('Ctrl Pts',(100.349869898682,-1.82803245302927,-0.0261573112120664));
#26930=CARTESIAN_POINT('Ctrl Pts',(100.349869898682,-1.82618711014666,-0.0410101441524499));
#26931=CARTESIAN_POINT('Ctrl Pts',(100.349869898682,-1.82416216292868,-0.0558261756737488));
#26932=CARTESIAN_POINT('Ctrl Pts',(100.349869898682,-1.81512268037586,-0.121965805017932));
#26933=CARTESIAN_POINT('Ctrl Pts',(100.349869898682,-1.80249961741194,-0.187453075270775));
#26934=CARTESIAN_POINT('Ctrl Pts',(100.349869898682,-1.78620616216057,-0.251987814725561));
#26935=CARTESIAN_POINT('Ctrl Pts',(100.349869898682,-1.77003269803693,-0.316047296106174));
#26936=CARTESIAN_POINT('Ctrl Pts',(100.349869898682,-1.75024259013835,-0.379169001456227));
#26937=CARTESIAN_POINT('Ctrl Pts',(100.349869898682,-1.72670765863925,-0.441032704914));
#26938=CARTESIAN_POINT('Ctrl Pts',(100.349869898682,-1.72060689789578,-0.457069108228596));
#26939=CARTESIAN_POINT('Ctrl Pts',(100.349869898682,-1.71425427817134,-0.473020805173369));
#26940=CARTESIAN_POINT('Ctrl Pts',(100.349869898682,-1.70764710160355,-0.488881825071062));
#26941=CARTESIAN_POINT('',(90.3490368852675,0.43141198410659,1.72456317283204));
#26942=CARTESIAN_POINT('Ctrl Pts',(90.3498698986825,0.431841315399937,1.72595542684201));
#26943=CARTESIAN_POINT('Ctrl Pts',(90.3498698986825,0.474841144465499,1.72062771663675));
#26944=CARTESIAN_POINT('Ctrl Pts',(90.3498698986825,0.517549233669024,1.71363307981672));
#26945=CARTESIAN_POINT('Ctrl Pts',(90.3498698986825,0.55987274194016,1.70495472032253));
#26946=CARTESIAN_POINT('Ctrl Pts',(90.3498698986825,0.624504400691931,1.69170211456593));
#26947=CARTESIAN_POINT('Ctrl Pts',(90.3498698986825,0.688239505721175,1.67452610531965));
#26948=CARTESIAN_POINT('Ctrl Pts',(90.3498698986825,0.750879107318416,1.65371126258147));
#26949=CARTESIAN_POINT('Ctrl Pts',(90.3498698986825,0.78576267441883,1.64211961856032));
#26950=CARTESIAN_POINT('Ctrl Pts',(90.3498698986825,0.82030656319226,1.62939848267545));
#26951=CARTESIAN_POINT('Ctrl Pts',(90.3498698986825,0.854476163578898,1.61559006912157));
#26952=CARTESIAN_POINT('Ctrl Pts',(90.3498698986825,0.86779419338757,1.61020806695472));
#26953=CARTESIAN_POINT('Ctrl Pts',(90.3498698986825,0.881057426269843,1.6046599411249));
#26954=CARTESIAN_POINT('Ctrl Pts',(90.3498698986825,0.894257109673284,1.59895090028478));
#26955=CARTESIAN_POINT('Ctrl Pts',(90.3498698986825,0.95740243452862,1.57163969686851));
#26956=CARTESIAN_POINT('Ctrl Pts',(90.3498698986825,1.01896094569028,1.54070914056002));
#26957=CARTESIAN_POINT('Ctrl Pts',(90.3498698986825,1.07871772693759,1.50646956606796));
#26958=CARTESIAN_POINT('Ctrl Pts',(90.3498698986825,1.1384745081849,1.4722299915759));
#26959=CARTESIAN_POINT('Ctrl Pts',(90.3498698986825,1.19643034452649,1.43468089597475));
#26960=CARTESIAN_POINT('Ctrl Pts',(90.3498698986825,1.25236316356459,1.39408084780543));
#26961=CARTESIAN_POINT('Ctrl Pts',(90.3498698986825,1.26444032963695,1.38531437522781));
#26962=CARTESIAN_POINT('Ctrl Pts',(90.3498698986825,1.27642312556603,1.37640548370779));
#26963=CARTESIAN_POINT('Ctrl Pts',(90.3498698986825,1.28830921630361,1.3673564950876));
#26964=CARTESIAN_POINT('Ctrl Pts',(90.3498698986825,1.30329584009538,1.35594704254841));
#26965=CARTESIAN_POINT('Ctrl Pts',(90.3498698986825,1.31813332928755,1.34431096898488));
#26966=CARTESIAN_POINT('Ctrl Pts',(90.3498698986825,1.33279071859542,1.33247444330211));
#26967=CARTESIAN_POINT('Ctrl Pts',(90.3498698986825,1.38865459604757,1.2873617560211));
#26968=CARTESIAN_POINT('Ctrl Pts',(90.3498698986825,1.44196466536913,1.23929766435431));
#26969=CARTESIAN_POINT('Ctrl Pts',(90.3498698986825,1.49249617721103,1.18859455163048));
#26970=CARTESIAN_POINT('Ctrl Pts',(90.3498698986825,1.54366615097348,1.13725080882164));
#26971=CARTESIAN_POINT('Ctrl Pts',(90.3498698986825,1.59198784076943,1.08320041802009));
#26972=CARTESIAN_POINT('Ctrl Pts',(90.3498698986825,1.63721050702468,1.02671705930785));
#26973=CARTESIAN_POINT('Ctrl Pts',(90.3498698986825,1.6821386474709,0.970601564949918));
#26974=CARTESIAN_POINT('Ctrl Pts',(90.3498698986825,1.72400888489749,0.912084010178768));
#26975=CARTESIAN_POINT('Ctrl Pts',(90.3498698986825,1.76254479103065,0.851392268311232));
#26976=CARTESIAN_POINT('Ctrl Pts',(90.3498698986825,1.77300783767251,0.834913597127501));
#26977=CARTESIAN_POINT('Ctrl Pts',(90.3498698986825,1.7832248602594,0.818274445593801));
#26978=CARTESIAN_POINT('Ctrl Pts',(90.3498698986825,1.79318980004416,0.801478956440628));
#26979=CARTESIAN_POINT('Ctrl Pts',(90.3498698986825,1.79955534257004,0.790750100797067));
#26980=CARTESIAN_POINT('Ctrl Pts',(90.3498698986825,1.80581833349577,0.779956701588126));
#26981=CARTESIAN_POINT('Ctrl Pts',(90.3498698986825,1.8119692394867,0.769114285455295));
#26982=CARTESIAN_POINT('Ctrl Pts',(90.3498698986825,1.84875184073079,0.704276313663121));
#26983=CARTESIAN_POINT('Ctrl Pts',(90.3498698986825,1.88159981518028,0.637570922779398));
#26984=CARTESIAN_POINT('Ctrl Pts',(90.3498698986825,1.91026209575643,0.56929255805336));
#26985=CARTESIAN_POINT('Ctrl Pts',(90.3498698986825,1.9192117974947,0.547972865858894));
#26986=CARTESIAN_POINT('Ctrl Pts',(90.3498698986825,1.9277531868049,0.526499495860398));
#26987=CARTESIAN_POINT('Ctrl Pts',(90.3498698986825,1.93587796203388,0.504880604295509));
#26988=CARTESIAN_POINT('Ctrl Pts',(90.3498698986825,1.96125429222847,0.437357735621539));
#26989=CARTESIAN_POINT('Ctrl Pts',(90.3498698986825,1.98257013429095,0.368417422671432));
#26990=CARTESIAN_POINT('Ctrl Pts',(90.3498698986825,1.99995022625152,0.298378990239343));
#26991=CARTESIAN_POINT('Ctrl Pts',(90.3498698986825,2.01733031821208,0.228340557807258));
#26992=CARTESIAN_POINT('Ctrl Pts',(90.3498698986825,2.03077467779787,0.157203167161218));
#26993=CARTESIAN_POINT('Ctrl Pts',(90.3498698986825,2.04036047300214,0.0852645536046799));
#26994=CARTESIAN_POINT('Ctrl Pts',(90.3498698986825,2.04251882481325,0.0690667490876816));
#26995=CARTESIAN_POINT('Ctrl Pts',(90.3498698986825,2.04448173438142,0.0528237008312667));
#26996=CARTESIAN_POINT('Ctrl Pts',(90.3498698986825,2.04624695875266,0.0365679053387177));
#26997=CARTESIAN_POINT('Ctrl Pts',(90.3498698986825,2.05428355565192,-0.0374404064539693));
#26998=CARTESIAN_POINT('Ctrl Pts',(90.3498698986825,2.05824267691534,-0.1118154870067));
#26999=CARTESIAN_POINT('Ctrl Pts',(90.3498698986825,2.0582761742277,-0.18621558070567));
#27000=CARTESIAN_POINT('Ctrl Pts',(90.3498698986825,2.05831029294659,-0.261995865834513));
#27001=CARTESIAN_POINT('Ctrl Pts',(90.3498698986825,2.05427191440651,-0.337802955295744));
#27002=CARTESIAN_POINT('Ctrl Pts',(90.3498698986825,2.04627147702015,-0.413297832844443));
#27003=CARTESIAN_POINT('Ctrl Pts',(90.3498698986825,2.03818548363352,-0.489600046223829));
#27004=CARTESIAN_POINT('Ctrl Pts',(90.3498698986825,2.02605230739823,-0.565584325798713));
#27005=CARTESIAN_POINT('Ctrl Pts',(90.3498698986825,2.00993395348048,-0.640908956132829));
#27006=CARTESIAN_POINT('Ctrl Pts',(90.3498698986825,2.0038696133045,-0.669248958114903));
#27007=CARTESIAN_POINT('Ctrl Pts',(90.3498698986825,1.997240622828,-0.697495588968377));
#27008=CARTESIAN_POINT('Ctrl Pts',(90.3498698986825,1.99004837701445,-0.725630494083074));
#27009=CARTESIAN_POINT('Ctrl Pts',(90.3498698986825,1.9868300478939,-0.738220078307771));
#27010=CARTESIAN_POINT('Ctrl Pts',(90.3498698986825,1.98349864718324,-0.750787978975288));
#27011=CARTESIAN_POINT('Ctrl Pts',(90.3498698986825,1.98005882552642,-0.763316755998213));
#27012=CARTESIAN_POINT('Ctrl Pts',(90.3498698986825,1.9590923373259,-0.839682475452813));
#27013=CARTESIAN_POINT('Ctrl Pts',(90.3498698986825,1.93406748684485,-0.914733173083993));
#27014=CARTESIAN_POINT('Ctrl Pts',(90.3498698986825,1.9051109069263,-0.988108398973491));
#27015=CARTESIAN_POINT('Ctrl Pts',(90.3498698986825,1.87610067910297,-1.06161956726859));
#27016=CARTESIAN_POINT('Ctrl Pts',(90.3498698986825,1.84314408918446,-1.13345011149863));
#27017=CARTESIAN_POINT('Ctrl Pts',(90.3498698986825,1.80631634284738,-1.20323986435587));
#27018=CARTESIAN_POINT('Ctrl Pts',(90.3498698986825,1.77027623607485,-1.27153701513948));
#27019=CARTESIAN_POINT('Ctrl Pts',(90.3498698986825,1.73052856007933,-1.33788070101697));
#27020=CARTESIAN_POINT('Ctrl Pts',(90.3498698986825,1.68709628884852,-1.40192061396576));
#27021=CARTESIAN_POINT('Ctrl Pts',(90.3498698986825,1.66663353523184,-1.43209248670392));
#27022=CARTESIAN_POINT('Ctrl Pts',(90.3498698986825,1.64535222417335,-1.46175270636565));
#27023=CARTESIAN_POINT('Ctrl Pts',(90.3498698986825,1.62325119196239,-1.49086269246791));
#27024=CARTESIAN_POINT('Ctrl Pts',(90.3490368852675,0.431058928865748,1.7231518396082));
#27025=CARTESIAN_POINT('Ctrl Pts',(90.3493145564058,0.423441373996219,1.72505742620083));
#27026=CARTESIAN_POINT('Ctrl Pts',(90.3495922275442,0.415811182876356,1.72691249954867));
#27027=CARTESIAN_POINT('Ctrl Pts',(90.3498698986825,0.408169026503128,1.72871689651704));
#27028=CARTESIAN_POINT('Origin',(90.3498698986825,-2.40291074888303E-16,
0.));
#27029=CARTESIAN_POINT('Ctrl Pts',(90.3498698986825,-0.214101726762248,
-2.19357617843498));
#27030=CARTESIAN_POINT('Ctrl Pts',(90.3498698986825,-0.253065554508827,
-2.18618780244257));
#27031=CARTESIAN_POINT('Ctrl Pts',(90.3498698986825,-0.291777125231032,
-2.17767057969179));
#27032=CARTESIAN_POINT('Ctrl Pts',(90.3498698986825,-0.330194078040922,
-2.16800471972978));
#27033=CARTESIAN_POINT('Ctrl Pts',(90.3498698986825,-0.406738639557457,
-2.14874579994681));
#27034=CARTESIAN_POINT('Ctrl Pts',(90.3498698986825,-0.482115441150976,
-2.12492954084015));
#27035=CARTESIAN_POINT('Ctrl Pts',(90.3498698986825,-0.556039436089016,
-2.09682490938438));
#27036=CARTESIAN_POINT('Ctrl Pts',(90.3498698986825,-0.591892015180994,
-2.08319437544255));
#27037=CARTESIAN_POINT('Ctrl Pts',(90.3498698986825,-0.627402453821627,
-2.06855445597946));
#27038=CARTESIAN_POINT('Ctrl Pts',(90.3498698986825,-0.662535477352677,
-2.05293241695312));
#27039=CARTESIAN_POINT('Ctrl Pts',(90.3498698986825,-0.679780447079462,
-2.04526437238981));
#27040=CARTESIAN_POINT('Ctrl Pts',(90.3498698986825,-0.696934454724013,
-2.03735967383536));
#27041=CARTESIAN_POINT('Ctrl Pts',(90.3498698986825,-0.713993138554709,
-2.02922138301725));
#27042=CARTESIAN_POINT('Ctrl Pts',(90.3498698986825,-0.726153529799601,
-2.02341995065617));
#27043=CARTESIAN_POINT('Ctrl Pts',(90.3498698986825,-0.738263467090769,
-2.01750071137785));
#27044=CARTESIAN_POINT('Ctrl Pts',(90.3498698986825,-0.750313634121252,
-2.01146892060575));
#27045=CARTESIAN_POINT('Ctrl Pts',(90.3498698986825,-0.820320629230508,
-1.97642645637979));
#27046=CARTESIAN_POINT('Ctrl Pts',(90.3498698986825,-0.888389925908362,
-1.93755209172309));
#27047=CARTESIAN_POINT('Ctrl Pts',(90.3498698986825,-0.954242008517751,
-1.89510921264174));
#27048=CARTESIAN_POINT('Ctrl Pts',(90.3498698986825,-1.00375379708154,-1.86319795377422));
#27049=CARTESIAN_POINT('Ctrl Pts',(90.3498698986825,-1.0520116823982,-1.82926838600638));
#27050=CARTESIAN_POINT('Ctrl Pts',(90.3498698986825,-1.09888241457236,-1.7934195088416));
#27051=CARTESIAN_POINT('Ctrl Pts',(90.3498698986825,-1.12145931356829,-1.77615166510791));
#27052=CARTESIAN_POINT('Ctrl Pts',(90.3498698986825,-1.14371416086655,-1.75843836186297));
#27053=CARTESIAN_POINT('Ctrl Pts',(90.3498698986825,-1.16563083104683,-1.74028997732421));
#27054=CARTESIAN_POINT('Ctrl Pts',(90.3498698986825,-1.17633935367306,-1.73142264552316));
#27055=CARTESIAN_POINT('Ctrl Pts',(90.3498698986825,-1.18696862372856,-1.72245015180798));
#27056=CARTESIAN_POINT('Ctrl Pts',(90.3498698986825,-1.19751194217376,-1.7133777644169));
#27057=CARTESIAN_POINT('Ctrl Pts',(90.3498698986825,-1.25555020266794,-1.66343660163746));
#27058=CARTESIAN_POINT('Ctrl Pts',(90.3498698986825,-1.31081695977831,-1.61061924094653));
#27059=CARTESIAN_POINT('Ctrl Pts',(90.3498698986825,-1.36305428431188,-1.55517048742002));
#27060=CARTESIAN_POINT('Ctrl Pts',(90.3498698986825,-1.41423592353542,-1.50084232027651));
#27061=CARTESIAN_POINT('Ctrl Pts',(90.3498698986825,-1.46250982428705,-1.44398719088105));
#27062=CARTESIAN_POINT('Ctrl Pts',(90.3498698986825,-1.50759196665253,-1.38480940421943));
#27063=CARTESIAN_POINT('Ctrl Pts',(90.3498698986825,-1.55169882702195,-1.32691183688347));
#27064=CARTESIAN_POINT('Ctrl Pts',(90.3498698986825,-1.59275091350146,-1.26679030650822));
#27065=CARTESIAN_POINT('Ctrl Pts',(90.3498698986825,-1.63043591394234,-1.20462243846732));
#27066=CARTESIAN_POINT('Ctrl Pts',(90.3498698986825,-1.64313694391479,-1.18366991236746));
#27067=CARTESIAN_POINT('Ctrl Pts',(90.3498698986825,-1.6554550854017,-1.16248487188985));
#27068=CARTESIAN_POINT('Ctrl Pts',(90.3498698986825,-1.66737704460729,-1.14107396752519));
#27069=CARTESIAN_POINT('Ctrl Pts',(90.3498698986825,-1.67411655420061,-1.12897033649619));
#27070=CARTESIAN_POINT('Ctrl Pts',(90.3498698986825,-1.68072944440791,-1.11679452622329));
#27071=CARTESIAN_POINT('Ctrl Pts',(90.3498698986825,-1.68721321125449,-1.10454773595022));
#27072=CARTESIAN_POINT('Ctrl Pts',(90.3498698986825,-1.69280679091002,-1.09398236576683));
#27073=CARTESIAN_POINT('Ctrl Pts',(90.3498698986825,-1.69830255810943,-1.08336726810866));
#27074=CARTESIAN_POINT('Ctrl Pts',(90.3498698986825,-1.7036947776161,-1.07271211575908));
#27075=CARTESIAN_POINT('Ctrl Pts',(90.3498698986825,-1.73609336482417,-1.00869174674665));
#27076=CARTESIAN_POINT('Ctrl Pts',(90.3498698986825,-1.76480709245594,-0.9431339500233));
#27077=CARTESIAN_POINT('Ctrl Pts',(90.3498698986825,-1.78957581068588,-0.876226598183046));
#27078=CARTESIAN_POINT('Ctrl Pts',(90.3498698986825,-1.79745850836397,-0.854933190017841));
#27079=CARTESIAN_POINT('Ctrl Pts',(90.3498698986825,-1.80494126152076,-0.833502987124966));
#27080=CARTESIAN_POINT('Ctrl Pts',(90.3498698986825,-1.81201458800382,-0.811941804694486));
#27081=CARTESIAN_POINT('Ctrl Pts',(90.3498698986825,-1.8348025884842,-0.74247855614232));
#27082=CARTESIAN_POINT('Ctrl Pts',(90.3498698986825,-1.85334501760212,-0.671655559779614));
#27083=CARTESIAN_POINT('Ctrl Pts',(90.3498698986825,-1.86769676549779,-0.599832699437972));
#27084=CARTESIAN_POINT('Ctrl Pts',(90.3498698986825,-1.88119220525484,-0.532295205610333));
#27085=CARTESIAN_POINT('Ctrl Pts',(90.3498698986825,-1.89098144653552,-0.463872822086227));
#27086=CARTESIAN_POINT('Ctrl Pts',(90.3498698986825,-1.8970692592514,-0.394874641297999));
#27087=CARTESIAN_POINT('Ctrl Pts',(90.3498698986825,-1.89846100872212,-0.379100801649089));
#27088=CARTESIAN_POINT('Ctrl Pts',(90.3498698986825,-1.89965930467989,-0.363292543085896));
#27089=CARTESIAN_POINT('Ctrl Pts',(90.3498698986825,-1.90066249818027,-0.347482308863442));
#27090=CARTESIAN_POINT('Ctrl Pts',(90.3498698986825,-1.90518355320309,-0.27623091138485));
#27091=CARTESIAN_POINT('Ctrl Pts',(90.3498698986825,-1.90575774275523,-0.204834546543544));
#27092=CARTESIAN_POINT('Ctrl Pts',(90.3498698986825,-1.90246416416827,-0.133627830062588));
#27093=CARTESIAN_POINT('Ctrl Pts',(90.3498698986825,-1.89918981650835,-0.0628368835816743));
#27094=CARTESIAN_POINT('Ctrl Pts',(90.3498698986825,-1.8920923557442,0.00776763413713237));
#27095=CARTESIAN_POINT('Ctrl Pts',(90.3498698986825,-1.88120052057599,0.0778439105212068));
#27096=CARTESIAN_POINT('Ctrl Pts',(90.3498698986825,-1.87040101393505,0.14732616034363));
#27097=CARTESIAN_POINT('Ctrl Pts',(90.3498698986825,-1.85587082135331,0.21629000314705));
#27098=CARTESIAN_POINT('Ctrl Pts',(90.3498698986825,-1.8375952377848,0.284375112098305));
#27099=CARTESIAN_POINT('Ctrl Pts',(90.3498698986825,-1.83323021278472,0.300636874771505));
#27100=CARTESIAN_POINT('Ctrl Pts',(90.3498698986825,-1.82865134630035,0.316848351257566));
#27101=CARTESIAN_POINT('Ctrl Pts',(90.3498698986825,-1.82385810846294,0.333004312157772));
#27102=CARTESIAN_POINT('Ctrl Pts',(90.3498698986825,-1.81904913961758,0.34921329557804));
#27103=CARTESIAN_POINT('Ctrl Pts',(90.3498698986825,-1.81402317448659,0.365369472788698));
#27104=CARTESIAN_POINT('Ctrl Pts',(90.3498698986825,-1.8087903340904,0.381436299405338));
#27105=CARTESIAN_POINT('Ctrl Pts',(90.3498698986825,-1.78750081560853,0.446803284885943));
#27106=CARTESIAN_POINT('Ctrl Pts',(90.3498698986825,-1.76275858577996,0.510807133920073));
#27107=CARTESIAN_POINT('Ctrl Pts',(90.3498698986825,-1.73459751006973,0.573134766921553));
#27108=CARTESIAN_POINT('Ctrl Pts',(90.3498698986825,-1.70726855933418,0.633620695416873));
#27109=CARTESIAN_POINT('Ctrl Pts',(90.3498698986825,-1.67671932469926,0.69252867029316));
#27110=CARTESIAN_POINT('Ctrl Pts',(90.3498698986825,-1.64294315627481,0.749542922188809));
#27111=CARTESIAN_POINT('Ctrl Pts',(90.3498698986825,-1.61044975030382,0.80439186804012));
#27112=CARTESIAN_POINT('Ctrl Pts',(90.3498698986825,-1.57496942494184,0.857488626202311));
#27113=CARTESIAN_POINT('Ctrl Pts',(90.3498698986825,-1.53646769662716,0.908516538747599));
#27114=CARTESIAN_POINT('Ctrl Pts',(90.3498698986825,-1.52109669050735,0.92888836075008));
#27115=CARTESIAN_POINT('Ctrl Pts',(90.3498698986825,-1.50524382897346,0.948930000897399));
#27116=CARTESIAN_POINT('Ctrl Pts',(90.3498698986825,-1.4889058019033,0.968619417293814));
#27117=CARTESIAN_POINT('Ctrl Pts',(90.0997129159169,-1.85158348337331,1.20554584720227));
#27118=CARTESIAN_POINT('Ctrl Pts',(90.1394446688446,-2.25287748833822,0.589243178206973));
#27119=CARTESIAN_POINT('Ctrl Pts',(90.2188933271119,-2.38405002538366,-1.06497837133754));
#27120=CARTESIAN_POINT('Ctrl Pts',(90.3380588907191,-0.393267651591904,
-2.58386764348672));
#27121=CARTESIAN_POINT('Ctrl Pts',(90.4572096067382,1.95719317887114,-1.72895644355711));
#27122=CARTESIAN_POINT('Ctrl Pts',(90.5763603227573,2.51434751199701,0.707435449009888));
#27123=CARTESIAN_POINT('Ctrl Pts',(90.6955110387765,0.767367608217681,2.49699416595646));
#27124=CARTESIAN_POINT('Ctrl Pts',(90.8146617547956,-1.68275183884718,1.99769159455853));
#27125=CARTESIAN_POINT('Ctrl Pts',(90.9338124708148,-2.59088897700703,-0.331852868955999));
#27126=CARTESIAN_POINT('Ctrl Pts',(91.052963186834,-1.12483059132128,-2.35748208545346));
#27127=CARTESIAN_POINT('Ctrl Pts',(91.1721139028529,1.37197072238487,-2.22272057647922));
#27128=CARTESIAN_POINT('Ctrl Pts',(91.2912646188722,2.61155722900937,-0.0511948499463282));
#27129=CARTESIAN_POINT('Ctrl Pts',(91.4104153348913,1.45801849094823,2.16726666247893));
#27130=CARTESIAN_POINT('Ctrl Pts',(91.5295660509104,-1.03158781574602,2.39972247460381));
#27131=CARTESIAN_POINT('Ctrl Pts',(91.6487167669297,-2.57588976083882,0.433176917311585));
#27132=CARTESIAN_POINT('Ctrl Pts',(91.7678674829486,-1.75975190745909,-1.93031708468522));
#27133=CARTESIAN_POINT('Ctrl Pts',(91.887018198968,0.668950253188048,-2.52494630594999));
#27134=CARTESIAN_POINT('Ctrl Pts',(92.0061689149869,2.48465391237723,-0.805819131213874));
#27135=CARTESIAN_POINT('Ctrl Pts',(92.1253196310062,2.02352271608646,1.651727978272));
#27136=CARTESIAN_POINT('Ctrl Pts',(92.2444703470252,-0.291881605843824,
2.59569919906983));
#27137=CARTESIAN_POINT('Ctrl Pts',(92.3636210630443,-2.33981761373509,1.16107833831933));
#27138=CARTESIAN_POINT('Ctrl Pts',(92.4827717790636,-2.24364082358645,-1.33750708770756));
#27139=CARTESIAN_POINT('Ctrl Pts',(92.6019224950827,-0.091483701489442,
-2.61045590933086));
#27140=CARTESIAN_POINT('Ctrl Pts',(92.7210732111018,2.14450532932704,-1.49129012506569));
#27141=CARTESIAN_POINT('Ctrl Pts',(92.840223927121,2.41535772310533,0.994432707684751));
#27142=CARTESIAN_POINT('Ctrl Pts',(92.9593746431402,0.47287546714399,2.56889823265659));
#27143=CARTESIAN_POINT('Ctrl Pts',(93.0785253591591,-1.90293045211532,1.78933089016224));
#27144=CARTESIAN_POINT('Ctrl Pts',(93.1976760751785,-2.53496903377393,-0.629905816124492));
#27145=CARTESIAN_POINT('Ctrl Pts',(93.3168267911975,-0.844066071326822,
-2.47192269423254));
#27146=CARTESIAN_POINT('Ctrl Pts',(93.4359775072166,1.62030438400931,-2.04877110545688));
#27147=CARTESIAN_POINT('Ctrl Pts',(93.5551282232358,2.59989442679698,0.25179020789872));
#27148=CARTESIAN_POINT('Ctrl Pts',(93.674278939255,1.19704796093923,2.32162131245874));
#27149=CARTESIAN_POINT('Ctrl Pts',(93.793429655274,-1.30272410903316,2.26401396529279));
#27150=CARTESIAN_POINT('Ctrl Pts',(93.9125803712933,-2.60873329153225,0.131757174118624));
#27151=CARTESIAN_POINT('Ctrl Pts',(94.0317310873123,-1.52420639263788,-2.12123648184726));
#27152=CARTESIAN_POINT('Ctrl Pts',(94.1508818033315,0.957040665009202,-2.43041611762311));
#27153=CARTESIAN_POINT('Ctrl Pts',(94.2700325193506,2.56129495053503,-0.512462208991841));
#27154=CARTESIAN_POINT('Ctrl Pts',(94.3891832353698,1.81848370267727,1.87509102775788));
#27155=CARTESIAN_POINT('Ctrl Pts',(94.5083339513889,-0.590711348686661,
2.54438783242932));
#27156=CARTESIAN_POINT('Ctrl Pts',(94.6274846674082,-2.45860277299606,0.88211209259215));
#27157=CARTESIAN_POINT('Ctrl Pts',(94.746635383427,-2.07353155917781,-1.58849495195136));
#27158=CARTESIAN_POINT('Ctrl Pts',(94.8657860994464,0.211638842323955,-2.60347044148789));
#27159=CARTESIAN_POINT('Ctrl Pts',(94.9849368154654,2.30287209799251,-1.232732509334));
#27160=CARTESIAN_POINT('Ctrl Pts',(95.1040875314846,2.28384791226018,1.26763088197871));
#27161=CARTESIAN_POINT('Ctrl Pts',(95.2232382475037,0.171999267854588,2.60638937826619));
#27162=CARTESIAN_POINT('Ctrl Pts',(95.3423889635229,-2.0974624438256,1.55675965904262));
#27163=CARTESIAN_POINT('Ctrl Pts',(95.461539679542,-2.44489568766324,-0.91942069572478));
#27164=CARTESIAN_POINT('Ctrl Pts',(95.5806903955612,-0.551926903599348,
-2.55308167365726));
#27165=CARTESIAN_POINT('Ctrl Pts',(95.6998411115801,1.84680503441703,-1.84720342792373));
#27166=CARTESIAN_POINT('Ctrl Pts',(95.8189918275996,2.55320066331205,0.551376198383756));
#27167=CARTESIAN_POINT('Ctrl Pts',(95.9381425436185,0.919948031306832,2.44469731438807));
#27168=CARTESIAN_POINT('Ctrl Pts',(96.0572932596377,-1.55630720620991,2.0977981836154));
#27169=CARTESIAN_POINT('Ctrl Pts',(96.1764439756568,-2.60642641738223,-0.171437073158325));
#27170=CARTESIAN_POINT('Ctrl Pts',(96.295594691676,-1.26812347191844,-2.2835744347958));
#27171=CARTESIAN_POINT('Ctrl Pts',(96.4147454076951,1.23223575776735,-2.30313794127868));
#27172=CARTESIAN_POINT('Ctrl Pts',(96.5338961237143,2.60342473103421,-0.212200398490957));
#27173=CARTESIAN_POINT('Ctrl Pts',(96.6530468397333,1.58894216979488,2.07318887715146));
#27174=CARTESIAN_POINT('Ctrl Pts',(96.7721975557526,-0.881581758524136,
2.45879298483808));
#27175=CARTESIAN_POINT('Ctrl Pts',(96.8913482717716,-2.54426035849811,0.591260152097927));
#27176=CARTESIAN_POINT('Ctrl Pts',(97.0104989877908,-1.87548322584963,-1.81807920865716));
#27177=CARTESIAN_POINT('Ctrl Pts',(97.1296497038099,0.51190973312449,-2.56140542752596));
#27178=CARTESIAN_POINT('Ctrl Pts',(97.2488004198291,2.43020963014491,-0.957564876617346));
#27179=CARTESIAN_POINT('Ctrl Pts',(97.3679511358482,2.12156519947923,1.52374881277565));
#27180=CARTESIAN_POINT('Ctrl Pts',(97.4871018518674,-0.131194474865119,
2.60876165008183));
#27181=CARTESIAN_POINT('Ctrl Pts',(97.6062525678865,-2.26373291861835,1.30321242084377));
#27182=CARTESIAN_POINT('Ctrl Pts',(97.7254032839056,-2.32187945857944,-1.19654716766928));
#27183=CARTESIAN_POINT('Ctrl Pts',(97.8445539999248,-0.252350991148042,
-2.59984005266964));
#27184=CARTESIAN_POINT('Ctrl Pts',(97.9637047159438,2.04842156151389,-1.62074626677239));
#27185=CARTESIAN_POINT('Ctrl Pts',(98.0828554319631,2.47210470191559,0.843532877857234));
#27186=CARTESIAN_POINT('Ctrl Pts',(98.2020061479821,0.630452581901348,2.53483308047208));
#27187=CARTESIAN_POINT('Ctrl Pts',(98.3211568640014,-1.78892038175012,1.90331641207747));
#27188=CARTESIAN_POINT('Ctrl Pts',(98.4403075800203,-2.56900019101066,-0.472321453153471));
#27189=CARTESIAN_POINT('Ctrl Pts',(98.5594582960397,-0.994953629969765,
-2.41514296955291));
#27190=CARTESIAN_POINT('Ctrl Pts',(98.6786090120587,1.49082744648633,-2.14482734690619));
#27191=CARTESIAN_POINT('Ctrl Pts',(98.7977597280779,2.61047574120498,0.0909214290808899));
#27192=CARTESIAN_POINT('Ctrl Pts',(98.916910444097,1.33799068516524,2.24335068661261));
#27193=CARTESIAN_POINT('Ctrl Pts',(99.0360611601162,-1.16057298546944,2.34007116379782));
#27194=CARTESIAN_POINT('Ctrl Pts',(99.1552118761353,-2.59563744310819,0.292435184249233));
#27195=CARTESIAN_POINT('Ctrl Pts',(99.2743625921544,-1.65216189369095,-2.02315385011149));
#27196=CARTESIAN_POINT('Ctrl Pts',(99.3935133081736,0.805278172691334,-2.48485265297424));
#27197=CARTESIAN_POINT('Ctrl Pts',(99.5126640241926,2.52481192829851,-0.669445101955683));
#27198=CARTESIAN_POINT('Ctrl Pts',(99.6318147402118,1.93067675396188,1.75923640532605));
#27199=CARTESIAN_POINT('Ctrl Pts',(99.750965456231,-0.432581741288383,2.57618049601852));
#27200=CARTESIAN_POINT('Ctrl Pts',(99.8701161722501,-2.39957872863425,1.03171229065444));
#27201=CARTESIAN_POINT('Ctrl Pts',(99.9892668882692,-2.1674235249011,-1.45676723838871));
#27202=CARTESIAN_POINT('Ctrl Pts',(100.108417604288,0.050309877383694,-2.61313994288172));
#27203=CARTESIAN_POINT('Ctrl Pts',(100.227593394073,2.22361276397469,-1.36892539155596));
#27204=CARTESIAN_POINT('Ctrl Pts',(100.307052278519,2.31079582958269,0.288508099625264));
#27205=CARTESIAN_POINT('Ctrl Pts',(100.346794257624,1.99370331232002,0.952286295127252));
#27206=CARTESIAN_POINT('Ctrl Pts',(90.1837056635606,-1.72966766143192,1.12616778287543));
#27207=CARTESIAN_POINT('Ctrl Pts',(90.2234374164883,-2.10453882946033,0.550444999761564));
#27208=CARTESIAN_POINT('Ctrl Pts',(90.3028860747557,-2.22707443070803,-0.994855843967151));
#27209=CARTESIAN_POINT('Ctrl Pts',(90.4220516383629,-0.367373302556414,
-2.41373524039919));
#27210=CARTESIAN_POINT('Ctrl Pts',(90.5412023543819,1.82832358306688,-1.61511488695975));
#27211=CARTESIAN_POINT('Ctrl Pts',(90.660353070401,2.34879259841948,0.660855008532327));
#27212=CARTESIAN_POINT('Ctrl Pts',(90.7795037864203,0.716840989500684,2.33258186758639));
#27213=CARTESIAN_POINT('Ctrl Pts',(90.8986545024393,-1.57195258221161,1.86615541759267));
#27214=CARTESIAN_POINT('Ctrl Pts',(91.0178052184585,-2.42029426063201,-0.310002320144315));
#27215=CARTESIAN_POINT('Ctrl Pts',(91.1369559344777,-1.05076714923659,-2.20225583249695));
#27216=CARTESIAN_POINT('Ctrl Pts',(91.2561066504968,1.28163456427962,-2.07636757189643));
#27217=CARTESIAN_POINT('Ctrl Pts',(91.375257366516,2.43960163047397,-0.0478239718485028));
#27218=CARTESIAN_POINT('Ctrl Pts',(91.4944080825351,1.36201659617765,2.02456497017342));
#27219=CARTESIAN_POINT('Ctrl Pts',(91.6135587985541,-0.963663858986451,
2.24171494183538));
#27220=CARTESIAN_POINT('Ctrl Pts',(91.7327095145733,-2.4062826541417,0.404654779155604));
#27221=CARTESIAN_POINT('Ctrl Pts',(91.8518602305924,-1.64388265169106,-1.80321712073536));
#27222=CARTESIAN_POINT('Ctrl Pts',(91.9710109466116,0.624903835250292,-2.35869352447292));
#27223=CARTESIAN_POINT('Ctrl Pts',(92.0901616626308,2.32105414672393,-0.752760707113499));
#27224=CARTESIAN_POINT('Ctrl Pts',(92.2093123786497,1.89028571253566,1.54297145937729));
#27225=CARTESIAN_POINT('Ctrl Pts',(92.3284630946691,-0.27266292831427,2.42478775802007));
#27226=CARTESIAN_POINT('Ctrl Pts',(92.4476138106881,-2.1857544617719,1.08462819646738));
#27227=CARTESIAN_POINT('Ctrl Pts',(92.5667645267073,-2.09591034445596,-1.24944015612463));
#27228=CARTESIAN_POINT('Ctrl Pts',(92.6859152427263,-0.0854600407895548,
-2.438572826183));
#27229=CARTESIAN_POINT('Ctrl Pts',(92.8050659587456,2.00330233619691,-1.39309748996006));
#27230=CARTESIAN_POINT('Ctrl Pts',(92.9242166747647,2.2563207016914,0.92895519505221));
#27231=CARTESIAN_POINT('Ctrl Pts',(93.0433673907839,0.441739414262496,2.39975147674171));
#27232=CARTESIAN_POINT('Ctrl Pts',(93.162518106803,-1.77763373595305,1.67151403331608));
#27233=CARTESIAN_POINT('Ctrl Pts',(93.281668822822,-2.36805631494502,-0.5884302434549));
#27234=CARTESIAN_POINT('Ctrl Pts',(93.4008195388413,-0.78848931241601,-2.30916120400046));
#27235=CARTESIAN_POINT('Ctrl Pts',(93.5199702548604,1.5136169229547,-1.91387164478739));
#27236=CARTESIAN_POINT('Ctrl Pts',(93.6391209708795,2.42870675481237,0.235211311819554));
#27237=CARTESIAN_POINT('Ctrl Pts',(93.7582716868987,1.11822943216551,2.16875627931995));
#27238=CARTESIAN_POINT('Ctrl Pts',(93.8774224029177,-1.21694743088614,2.11494203526961));
#27239=CARTESIAN_POINT('Ctrl Pts',(93.996573118937,-2.43696363257869,0.123081743427209));
#27240=CARTESIAN_POINT('Ctrl Pts',(94.1157238349562,-1.4238464159825,-1.98156560470953));
#27241=CARTESIAN_POINT('Ctrl Pts',(94.2348745509751,0.894025197246792,-2.27038758998694));
#27242=CARTESIAN_POINT('Ctrl Pts',(94.3540252669942,2.39264882578134,-0.47871960327938));
#27243=CARTESIAN_POINT('Ctrl Pts',(94.4731759830136,1.69874730553947,1.75162737304458));
#27244=CARTESIAN_POINT('Ctrl Pts',(94.5923266990326,-0.551816499898084,
2.3768549414126));
#27245=CARTESIAN_POINT('Ctrl Pts',(94.7114774150519,-2.29671832080214,0.82403022818876));
#27246=CARTESIAN_POINT('Ctrl Pts',(94.8306281310708,-1.93700176906645,-1.48390195387379));
#27247=CARTESIAN_POINT('Ctrl Pts',(94.9497788470901,0.197703676208935,-2.43204731008477));
#27248=CARTESIAN_POINT('Ctrl Pts',(95.0689295631092,2.15124158974171,-1.15156436409024));
#27249=CARTESIAN_POINT('Ctrl Pts',(95.1880802791283,2.13347003412901,1.18416488528859));
#27250=CARTESIAN_POINT('Ctrl Pts',(95.3072309951474,0.160674133286185,2.4347740521391));
#27251=CARTESIAN_POINT('Ctrl Pts',(95.4263817111665,-1.95935694648968,1.45425624231758));
#27252=CARTESIAN_POINT('Ctrl Pts',(95.5455324271858,-2.28391376597346,-0.858882280451714));
#27253=CARTESIAN_POINT('Ctrl Pts',(95.6646831432049,-0.515585781144895,
-2.38497634461189));
#27254=CARTESIAN_POINT('Ctrl Pts',(95.7838338592239,1.72520384507921,-1.72557600672961));
#27255=CARTESIAN_POINT('Ctrl Pts',(95.9029845752431,2.38508749950162,0.515071336610853));
#27256=CARTESIAN_POINT('Ctrl Pts',(96.0221352912623,0.859374894104378,2.28372845440529));
#27257=CARTESIAN_POINT('Ctrl Pts',(96.1412860072814,-1.45383358082807,1.95967057979992));
#27258=CARTESIAN_POINT('Ctrl Pts',(96.2604367233005,-2.43480865244838,-0.160148955785822));
#27259=CARTESIAN_POINT('Ctrl Pts',(96.3795874393196,-1.18462504109399,-2.13321456353832));
#27260=CARTESIAN_POINT('Ctrl Pts',(96.4987381553389,1.15110032067646,-2.15148992881971));
#27261=CARTESIAN_POINT('Ctrl Pts',(96.6178888713579,2.43200460939413,-0.198228257223413));
#27262=CARTESIAN_POINT('Ctrl Pts',(96.7370395873772,1.48431972506719,1.9366816506249));
#27263=CARTESIAN_POINT('Ctrl Pts',(96.8561903033962,-0.823534813482703,
2.29689600831927));
#27264=CARTESIAN_POINT('Ctrl Pts',(96.9753410194154,-2.37673586088587,0.552329167850369));
#27265=CARTESIAN_POINT('Ctrl Pts',(97.0944917354345,-1.75199374721148,-1.6983694450584));
#27266=CARTESIAN_POINT('Ctrl Pts',(97.2136424514538,0.478203504680524,-2.39275202851578));
#27267=CARTESIAN_POINT('Ctrl Pts',(97.3327931674727,2.270194698488,-0.89451489262075));
#27268=CARTESIAN_POINT('Ctrl Pts',(97.4519438834919,1.98187267822947,1.42341896504805));
#27269=CARTESIAN_POINT('Ctrl Pts',(97.5710945995111,-0.122556094591716,
2.43699012388549));
#27270=CARTESIAN_POINT('Ctrl Pts',(97.6902453155302,-2.11467949385656,1.21740359025193));
#27271=CARTESIAN_POINT('Ctrl Pts',(97.8093960315494,-2.1689974280453,-1.11776161317067));
#27272=CARTESIAN_POINT('Ctrl Pts',(97.9285467475685,-0.235735170808409,
-2.42865596089974));
#27273=CARTESIAN_POINT('Ctrl Pts',(98.0476974635877,1.91354511624583,-1.51402971035114));
#27274=CARTESIAN_POINT('Ctrl Pts',(98.1668481796068,2.30933122755397,0.787991226583058));
#27275=CARTESIAN_POINT('Ctrl Pts',(98.285998895626,0.588941007938949,2.36792931336405));
#27276=CARTESIAN_POINT('Ctrl Pts',(98.4051496116451,-1.67113055445514,1.77799428273429));
#27277=CARTESIAN_POINT('Ctrl Pts',(98.5243003276642,-2.39984672174115,-0.44122187881679));
#27278=CARTESIAN_POINT('Ctrl Pts',(98.6434510436833,-0.929441817685516,
-2.25612008839036));
#27279=CARTESIAN_POINT('Ctrl Pts',(98.7626017597025,1.39266527602884,-2.00360315082291));
#27280=CARTESIAN_POINT('Ctrl Pts',(98.8817524757218,2.43859135224549,0.0849347906938011));
#27281=CARTESIAN_POINT('Ctrl Pts',(99.0009031917407,1.24989191154976,2.09563931128596));
#27282=CARTESIAN_POINT('Ctrl Pts',(99.12005390776,-1.08415611811398,2.18599131706251));
#27283=CARTESIAN_POINT('Ctrl Pts',(99.2392046237789,-2.42473006832328,0.27318005685557));
#27284=CARTESIAN_POINT('Ctrl Pts',(99.3583553397983,-1.5433768040321,-1.88994113420365));
#27285=CARTESIAN_POINT('Ctrl Pts',(99.4775060558172,0.752255367510413,-2.32123980142798));
#27286=CARTESIAN_POINT('Ctrl Pts',(99.5966567718365,2.35856799479508,-0.625366101153133));
#27287=CARTESIAN_POINT('Ctrl Pts',(99.7158074878556,1.80355310791724,1.64340109232476));
#27288=CARTESIAN_POINT('Ctrl Pts',(99.8349582038747,-0.404098791953626,
2.40655424612925));
#27289=CARTESIAN_POINT('Ctrl Pts',(99.9541089198937,-2.24158066068779,0.963780137958278));
#27290=CARTESIAN_POINT('Ctrl Pts',(100.073259635913,-2.02471150413276,-1.36084773119917));
#27291=CARTESIAN_POINT('Ctrl Pts',(100.192410351932,0.0469972694953342,
-2.44108013199815));
#27292=CARTESIAN_POINT('Ctrl Pts',(100.311586141717,2.07720101412182,-1.2787897504754));
#27293=CARTESIAN_POINT('Ctrl Pts',(100.391045026163,2.15864359046838,0.269511547528967));
#27294=CARTESIAN_POINT('Ctrl Pts',(100.430787005268,1.86242974015249,0.889583874503776));
#27295=CARTESIAN_POINT('Ctrl Pts',(90.2676984112045,-1.60775183949052,1.04678971854859));
#27296=CARTESIAN_POINT('Ctrl Pts',(90.3074301641321,-1.95620017058246,0.511646821316155));
#27297=CARTESIAN_POINT('Ctrl Pts',(90.3868788223997,-2.07009883603241,-0.924733316596755));
#27298=CARTESIAN_POINT('Ctrl Pts',(90.5060443860065,-0.341478953520925,
-2.24360283731166));
#27299=CARTESIAN_POINT('Ctrl Pts',(90.6251951020259,1.69945398726261,-1.50127333036239));
#27300=CARTESIAN_POINT('Ctrl Pts',(90.7443458180448,2.18323768484195,0.614274568054768));
#27301=CARTESIAN_POINT('Ctrl Pts',(90.863496534064,0.66631437078369,2.16816956921632));
#27302=CARTESIAN_POINT('Ctrl Pts',(90.9826472500832,-1.46115332557605,1.73461924062682));
#27303=CARTESIAN_POINT('Ctrl Pts',(91.1017979661023,-2.249699544257,-0.288151771332628));
#27304=CARTESIAN_POINT('Ctrl Pts',(91.2209486821215,-0.976703707151896,
-2.04702957954045));
#27305=CARTESIAN_POINT('Ctrl Pts',(91.3400993981407,1.19129840617438,-1.93001456731364));
#27306=CARTESIAN_POINT('Ctrl Pts',(91.4592501141596,2.26764603193859,-0.044453093750678));
#27307=CARTESIAN_POINT('Ctrl Pts',(91.578400830179,1.26601470140709,1.8818632778679));
#27308=CARTESIAN_POINT('Ctrl Pts',(91.6975515461979,-0.895739902226873,
2.08370740906695));
#27309=CARTESIAN_POINT('Ctrl Pts',(91.8167022622172,-2.23667554744459,0.376132640999623));
#27310=CARTESIAN_POINT('Ctrl Pts',(91.9358529782361,-1.52801339592303,-1.67611715678549));
#27311=CARTESIAN_POINT('Ctrl Pts',(92.0550036942554,0.580857417312533,-2.19244074299585));
#27312=CARTESIAN_POINT('Ctrl Pts',(92.1741544102744,2.15745438107064,-0.699702283013127));
#27313=CARTESIAN_POINT('Ctrl Pts',(92.2933051262937,1.75704870898488,1.43421494048258));
#27314=CARTESIAN_POINT('Ctrl Pts',(92.4124558423127,-0.253444250784714,
2.25387631697032));
#27315=CARTESIAN_POINT('Ctrl Pts',(92.531606558332,-2.0316913098087,1.00817805461546));
#27316=CARTESIAN_POINT('Ctrl Pts',(92.6507572743511,-1.94817986532546,-1.16137322454171));
#27317=CARTESIAN_POINT('Ctrl Pts',(92.7699079903702,-0.0794363800896707,
-2.26668974303514));
#27318=CARTESIAN_POINT('Ctrl Pts',(92.8890587063892,1.86209934306679,-1.29490485485441));
#27319=CARTESIAN_POINT('Ctrl Pts',(93.0082094224086,2.09728368027748,0.863477682419669));
#27320=CARTESIAN_POINT('Ctrl Pts',(93.1273601384276,0.410603361381006,2.23060472082685));
#27321=CARTESIAN_POINT('Ctrl Pts',(93.2465108544467,-1.6523370197908,1.55369717646994));
#27322=CARTESIAN_POINT('Ctrl Pts',(93.3656615704659,-2.2011435961161,-0.54695467078531));
#27323=CARTESIAN_POINT('Ctrl Pts',(93.484812286485,-0.732912553505195,-2.14639971376836));
#27324=CARTESIAN_POINT('Ctrl Pts',(93.6039630025041,1.40692946190011,-1.77897218411791));
#27325=CARTESIAN_POINT('Ctrl Pts',(93.7231137185235,2.25751908282776,0.218632415740387));
#27326=CARTESIAN_POINT('Ctrl Pts',(93.8422644345423,1.03941090339178,2.01589124618118));
#27327=CARTESIAN_POINT('Ctrl Pts',(93.9614151505618,-1.13117075273913,1.96587010524642));
#27328=CARTESIAN_POINT('Ctrl Pts',(94.0805658665806,-2.26519397362513,0.114406312735795));
#27329=CARTESIAN_POINT('Ctrl Pts',(94.1997165826001,-1.32348643932714,-1.84189472757179));
#27330=CARTESIAN_POINT('Ctrl Pts',(94.318867298619,0.831009729484381,-2.11035906235078));
#27331=CARTESIAN_POINT('Ctrl Pts',(94.4380180146384,2.22400270102766,-0.444976997566919));
#27332=CARTESIAN_POINT('Ctrl Pts',(94.5571687306571,1.57901090840168,1.62816371833129));
#27333=CARTESIAN_POINT('Ctrl Pts',(94.6763194466765,-0.512921651109511,
2.20932205039589));
#27334=CARTESIAN_POINT('Ctrl Pts',(94.7954701626955,-2.13483386860821,0.765948363785368));
#27335=CARTESIAN_POINT('Ctrl Pts',(94.9146208787147,-1.8004719789551,-1.37930895579624));
#27336=CARTESIAN_POINT('Ctrl Pts',(95.0337715947338,0.183768510093922,-2.26062417868165));
#27337=CARTESIAN_POINT('Ctrl Pts',(95.152922310753,1.99961108149091,-1.0703962188465));
#27338=CARTESIAN_POINT('Ctrl Pts',(95.2720730267721,1.98309215599787,1.10069888859847));
#27339=CARTESIAN_POINT('Ctrl Pts',(95.3912237427913,0.149348998717781,2.26315872601198));
#27340=CARTESIAN_POINT('Ctrl Pts',(95.5103744588103,-1.82125144915379,1.35175282559255));
#27341=CARTESIAN_POINT('Ctrl Pts',(95.6295251748296,-2.12293184428369,-0.79834386517865));
#27342=CARTESIAN_POINT('Ctrl Pts',(95.7486758908488,-0.479244658690441,
-2.21687101556651));
#27343=CARTESIAN_POINT('Ctrl Pts',(95.8678266068677,1.60360265574138,-1.60394858553549));
#27344=CARTESIAN_POINT('Ctrl Pts',(95.9869773228869,2.21697433569119,0.47876647483795));
#27345=CARTESIAN_POINT('Ctrl Pts',(96.106128038906,0.79880175690192,2.1227595944225));
#27346=CARTESIAN_POINT('Ctrl Pts',(96.2252787549253,-1.35135995544623,1.82154297598446));
#27347=CARTESIAN_POINT('Ctrl Pts',(96.3444294709443,-2.26319088751455,-0.148860838413323));
#27348=CARTESIAN_POINT('Ctrl Pts',(96.4635801869636,-1.10112661026953,-1.98285469228083));
#27349=CARTESIAN_POINT('Ctrl Pts',(96.5827309029826,1.06996488358556,-1.99984191636073));
#27350=CARTESIAN_POINT('Ctrl Pts',(96.7018816190017,2.26058448775406,-0.18425611595587));
#27351=CARTESIAN_POINT('Ctrl Pts',(96.8210323350211,1.3796972803395,1.80017442409833));
#27352=CARTESIAN_POINT('Ctrl Pts',(96.9401830510401,-0.765487868441268,
2.13499903180046));
#27353=CARTESIAN_POINT('Ctrl Pts',(97.0593337670593,-2.20921136327364,0.513398183602814));
#27354=CARTESIAN_POINT('Ctrl Pts',(97.1784844830784,-1.62850426857331,-1.57865968145962));
#27355=CARTESIAN_POINT('Ctrl Pts',(97.2976351990974,0.444497276236559,-2.22409862950561));
#27356=CARTESIAN_POINT('Ctrl Pts',(97.4167859151166,2.1101797668311,-0.831464908624157));
#27357=CARTESIAN_POINT('Ctrl Pts',(97.5359366311357,1.84218015697973,1.32308911732048));
#27358=CARTESIAN_POINT('Ctrl Pts',(97.6550873471549,-0.113917714318317,
2.26521859768917));
#27359=CARTESIAN_POINT('Ctrl Pts',(97.7742380631742,-1.96562606909477,1.13159475966008));
#27360=CARTESIAN_POINT('Ctrl Pts',(97.8933887791931,-2.01611539751116,-1.03897605867206));
#27361=CARTESIAN_POINT('Ctrl Pts',(98.0125394952124,-0.219119350468773,
-2.25747186912984));
#27362=CARTESIAN_POINT('Ctrl Pts',(98.1316902112315,1.77866867097777,-1.40731315392992));
#27363=CARTESIAN_POINT('Ctrl Pts',(98.2508409272507,2.14655775319236,0.732449575308886));
#27364=CARTESIAN_POINT('Ctrl Pts',(98.3699916432698,0.547429433976551,2.20102554625602));
#27365=CARTESIAN_POINT('Ctrl Pts',(98.4891423592887,-1.55334072716016,1.65267215339111));
#27366=CARTESIAN_POINT('Ctrl Pts',(98.6082930753081,-2.23069325247167,-0.41012230448011));
#27367=CARTESIAN_POINT('Ctrl Pts',(98.7274437913271,-0.863930005401265,
-2.09709720722778));
#27368=CARTESIAN_POINT('Ctrl Pts',(98.8465945073463,1.29450310557135,-1.86237895473961));
#27369=CARTESIAN_POINT('Ctrl Pts',(98.9657452233654,2.266706963286,0.0789481523067152));
#27370=CARTESIAN_POINT('Ctrl Pts',(99.0848959393846,1.16179313793426,1.94792793595931));
#27371=CARTESIAN_POINT('Ctrl Pts',(99.2040466554037,-1.00773925075854,2.03191147032719));
#27372=CARTESIAN_POINT('Ctrl Pts',(99.3231973714228,-2.25382269353839,0.253924929461906));
#27373=CARTESIAN_POINT('Ctrl Pts',(99.4423480874419,-1.43459171437324,-1.75672841829582));
#27374=CARTESIAN_POINT('Ctrl Pts',(99.561498803461,0.69923256232949,-2.15762694988174));
#27375=CARTESIAN_POINT('Ctrl Pts',(99.6806495194802,2.19232406129163,-0.581287100350585));
#27376=CARTESIAN_POINT('Ctrl Pts',(99.7998002354995,1.6764294618726,1.52756577932349));
#27377=CARTESIAN_POINT('Ctrl Pts',(99.9189509515185,-0.37561584261887,2.23692799623998));
#27378=CARTESIAN_POINT('Ctrl Pts',(100.038101667538,-2.08358259274135,0.895847985262117));
#27379=CARTESIAN_POINT('Ctrl Pts',(100.157252383557,-1.88199948336444,-1.26492822400963));
#27380=CARTESIAN_POINT('Ctrl Pts',(100.276403099576,0.0436846616069731,
-2.26902032111459));
#27381=CARTESIAN_POINT('Ctrl Pts',(100.395578889361,1.93078926426895,-1.18865410939485));
#27382=CARTESIAN_POINT('Ctrl Pts',(100.475037773807,2.00649135135404,0.250514995432669));
#27383=CARTESIAN_POINT('Ctrl Pts',(100.514779752912,1.73115616798497,0.826881453880298));
#27384=CARTESIAN_POINT('Ctrl Pts',(90.3516911588482,-1.48583601754912,0.967411654221745));
#27385=CARTESIAN_POINT('Ctrl Pts',(90.3914229117759,-1.80786151170457,0.472848642870747));
#27386=CARTESIAN_POINT('Ctrl Pts',(90.4708715700433,-1.91312324135679,-0.854610789226363));
#27387=CARTESIAN_POINT('Ctrl Pts',(90.5900371336504,-0.315584604485434,
-2.07347043422413));
#27388=CARTESIAN_POINT('Ctrl Pts',(90.7091878496695,1.57058439145835,-1.38743177376504));
#27389=CARTESIAN_POINT('Ctrl Pts',(90.8283385656886,2.01768277126442,0.567694127577208));
#27390=CARTESIAN_POINT('Ctrl Pts',(90.9474892817076,0.615787752066693,2.00375727084625));
#27391=CARTESIAN_POINT('Ctrl Pts',(91.066639997727,-1.35035406894049,1.60308306366094));
#27392=CARTESIAN_POINT('Ctrl Pts',(91.185790713746,-2.07910482788197,-0.266301222520941));
#27393=CARTESIAN_POINT('Ctrl Pts',(91.3049414297653,-0.902640265067203,
-1.89180332658395));
#27394=CARTESIAN_POINT('Ctrl Pts',(91.4240921457842,1.10096224806914,-1.78366156273085));
#27395=CARTESIAN_POINT('Ctrl Pts',(91.5432428618034,2.09569043340321,-0.0410822156528534));
#27396=CARTESIAN_POINT('Ctrl Pts',(91.6623935778227,1.17001280663651,1.73916158556239));
#27397=CARTESIAN_POINT('Ctrl Pts',(91.7815442938416,-0.827815945467298,
1.92569987629852));
#27398=CARTESIAN_POINT('Ctrl Pts',(91.9006950098609,-2.06706844074748,0.347610502843638));
#27399=CARTESIAN_POINT('Ctrl Pts',(92.0198457258799,-1.41214414015499,-1.54901719283562));
#27400=CARTESIAN_POINT('Ctrl Pts',(92.1389964418991,0.536810999374776,-2.02618796151878));
#27401=CARTESIAN_POINT('Ctrl Pts',(92.2581471579182,1.99385461541733,-0.64664385891275));
#27402=CARTESIAN_POINT('Ctrl Pts',(92.3772978739375,1.62381170543408,1.32545842158787));
#27403=CARTESIAN_POINT('Ctrl Pts',(92.4964485899565,-0.234225573255156,
2.08296487592058));
#27404=CARTESIAN_POINT('Ctrl Pts',(92.6155993059758,-1.87762815784551,0.931727912763529));
#27405=CARTESIAN_POINT('Ctrl Pts',(92.7347500219948,-1.80044938619497,-1.07330629295879));
#27406=CARTESIAN_POINT('Ctrl Pts',(92.853900738014,-0.0734127193897878,
-2.09480665988727));
#27407=CARTESIAN_POINT('Ctrl Pts',(92.9730514540332,1.72089634993666,-1.19671221974878));
#27408=CARTESIAN_POINT('Ctrl Pts',(93.0922021700523,1.93824665886355,0.798000169787126));
#27409=CARTESIAN_POINT('Ctrl Pts',(93.2113528860714,0.379467308499514,2.06145796491198));
#27410=CARTESIAN_POINT('Ctrl Pts',(93.3305036020905,-1.52704030362853,1.43588031962378));
#27411=CARTESIAN_POINT('Ctrl Pts',(93.4496543181096,-2.03423087728717,-0.505479098115718));
#27412=CARTESIAN_POINT('Ctrl Pts',(93.5688050341289,-0.67733579459438,-1.98363822353627));
#27413=CARTESIAN_POINT('Ctrl Pts',(93.6879557501479,1.3002420008455,-1.64407272344841));
#27414=CARTESIAN_POINT('Ctrl Pts',(93.8071064661672,2.08633141084316,0.202053519661223));
#27415=CARTESIAN_POINT('Ctrl Pts',(93.9262571821861,0.960592374618062,1.86302621304239));
#27416=CARTESIAN_POINT('Ctrl Pts',(94.0454078982054,-1.04539407459211,1.81679817522325));
#27417=CARTESIAN_POINT('Ctrl Pts',(94.1645586142245,-2.0934243146716,0.10573088204438));
#27418=CARTESIAN_POINT('Ctrl Pts',(94.2837093302435,-1.22312646267178,-1.70222385043407));
#27419=CARTESIAN_POINT('Ctrl Pts',(94.4028600462628,0.767994261721968,-1.95033053471462));
#27420=CARTESIAN_POINT('Ctrl Pts',(94.5220107622818,2.05535657627397,-0.411234391854458));
#27421=CARTESIAN_POINT('Ctrl Pts',(94.6411614783011,1.45927451126389,1.504700063618));
#27422=CARTESIAN_POINT('Ctrl Pts',(94.7603121943202,-0.474026802320936,
2.04178915937917));
#27423=CARTESIAN_POINT('Ctrl Pts',(94.8794629103393,-1.97294941641427,0.707866499381977));
#27424=CARTESIAN_POINT('Ctrl Pts',(94.9986136263584,-1.66394218884373,-1.27471595771868));
#27425=CARTESIAN_POINT('Ctrl Pts',(95.1177643423775,0.169833343978903,-2.08920104727853));
#27426=CARTESIAN_POINT('Ctrl Pts',(95.2369150583968,1.84798057324012,-0.989228073602758));
#27427=CARTESIAN_POINT('Ctrl Pts',(95.3560657744157,1.83271427786672,1.01723289190835));
#27428=CARTESIAN_POINT('Ctrl Pts',(95.475216490435,0.138023864149379,2.09154339988488));
#27429=CARTESIAN_POINT('Ctrl Pts',(95.5943672064542,-1.68314595181788,1.2492494088675));
#27430=CARTESIAN_POINT('Ctrl Pts',(95.7135179224733,-1.96194992259393,-0.737805449905584));
#27431=CARTESIAN_POINT('Ctrl Pts',(95.8326686384925,-0.442903536235988,
-2.04876568652113));
#27432=CARTESIAN_POINT('Ctrl Pts',(95.9518193545115,1.48200146640357,-1.48232116434138));
#27433=CARTESIAN_POINT('Ctrl Pts',(96.0709700705307,2.04886117188075,0.442461613065045));
#27434=CARTESIAN_POINT('Ctrl Pts',(96.1901207865498,0.738228619699466,1.96179073443972));
#27435=CARTESIAN_POINT('Ctrl Pts',(96.3092715025689,-1.24888633006439,1.68341537216896));
#27436=CARTESIAN_POINT('Ctrl Pts',(96.4284222185881,-2.0915731225807,-0.13757272104082));
#27437=CARTESIAN_POINT('Ctrl Pts',(96.5475729346072,-1.01762817944508,-1.83249482102335));
#27438=CARTESIAN_POINT('Ctrl Pts',(96.6667236506264,0.988829446494665,-1.84819390390174));
#27439=CARTESIAN_POINT('Ctrl Pts',(96.7858743666454,2.08916436611398,-0.170283974688326));
#27440=CARTESIAN_POINT('Ctrl Pts',(96.9050250826647,1.27507483561182,1.66366719757177));
#27441=CARTESIAN_POINT('Ctrl Pts',(97.0241757986838,-0.707440923399836,
1.97310205528165));
#27442=CARTESIAN_POINT('Ctrl Pts',(97.1433265147031,-2.0416868656614,0.474467199355257));
#27443=CARTESIAN_POINT('Ctrl Pts',(97.262477230722,-1.50501478993517,-1.45894991786086));
#27444=CARTESIAN_POINT('Ctrl Pts',(97.3816279467414,0.410791047792594,-2.05544523049543));
#27445=CARTESIAN_POINT('Ctrl Pts',(97.5007786627603,1.95016483517421,-0.768414924627563));
#27446=CARTESIAN_POINT('Ctrl Pts',(97.6199293787795,1.70248763572999,1.22275926959289));
#27447=CARTESIAN_POINT('Ctrl Pts',(97.7390800947986,-0.105279334044914,
2.09344707149284));
#27448=CARTESIAN_POINT('Ctrl Pts',(97.8582308108178,-1.81657264433298,1.04578592906823));
#27449=CARTESIAN_POINT('Ctrl Pts',(97.9773815268368,-1.86323336697702,-0.960190504173446));
#27450=CARTESIAN_POINT('Ctrl Pts',(98.0965322428562,-0.20250353012914,-2.08628777735995));
#27451=CARTESIAN_POINT('Ctrl Pts',(98.215682958875,1.64379222570971,-1.30059659750868));
#27452=CARTESIAN_POINT('Ctrl Pts',(98.3348336748945,1.98378427883073,0.676907924034713));
#27453=CARTESIAN_POINT('Ctrl Pts',(98.4539843909134,0.505917860014153,2.03412177914799));
#27454=CARTESIAN_POINT('Ctrl Pts',(98.5731351069327,-1.43555089986518,1.52735002404793));
#27455=CARTESIAN_POINT('Ctrl Pts',(98.6922858229516,-2.06153978320217,-0.379022730143428));
#27456=CARTESIAN_POINT('Ctrl Pts',(98.8114365389709,-0.798418193117015,
-1.93807432606522));
#27457=CARTESIAN_POINT('Ctrl Pts',(98.9305872549901,1.19634093511385,-1.72115475865633));
#27458=CARTESIAN_POINT('Ctrl Pts',(99.0497379710091,2.09482257432651,0.0729615139196275));
#27459=CARTESIAN_POINT('Ctrl Pts',(99.1688886870284,1.07369436431878,1.80021656063267));
#27460=CARTESIAN_POINT('Ctrl Pts',(99.2880394030473,-0.931322383403096,
1.87783162359188));
#27461=CARTESIAN_POINT('Ctrl Pts',(99.4071901190665,-2.08291531875349,0.234669802068244));
#27462=CARTESIAN_POINT('Ctrl Pts',(99.5263408350856,-1.32580662471439,-1.62351570238799));
#27463=CARTESIAN_POINT('Ctrl Pts',(99.6454915511049,0.646209757148569,-1.99401409833549));
#27464=CARTESIAN_POINT('Ctrl Pts',(99.764642267124,2.02608012778821,-0.537208099548037));
#27465=CARTESIAN_POINT('Ctrl Pts',(99.8837929831432,1.54930581582797,1.41173046632221));
#27466=CARTESIAN_POINT('Ctrl Pts',(100.002943699162,-0.347132893284113,
2.06730174635073));
#27467=CARTESIAN_POINT('Ctrl Pts',(100.122094415182,-1.92558452479489,0.827915832565954));
#27468=CARTESIAN_POINT('Ctrl Pts',(100.241245131201,-1.73928746259611,-1.1690087168201));
#27469=CARTESIAN_POINT('Ctrl Pts',(100.36039584722,0.0403720537186134,-2.09696051023103));
#27470=CARTESIAN_POINT('Ctrl Pts',(100.479571637005,1.78437751441608,-1.09851846831429));
#27471=CARTESIAN_POINT('Ctrl Pts',(100.559030521451,1.85433911223973,0.231518443336371));
#27472=CARTESIAN_POINT('Ctrl Pts',(100.598772500556,1.59988259581745,0.764179033256822));
#27473=CARTESIAN_POINT('',(100.350702918754,-0.0938353553295348,-1.775226569468));
#27474=CARTESIAN_POINT('Ctrl Pts',(100.349869898683,-0.0938337030310376,
-1.77668351508419));
#27475=CARTESIAN_POINT('Ctrl Pts',(100.349869898683,-0.0511432819576657,
-1.78421672036901));
#27476=CARTESIAN_POINT('Ctrl Pts',(100.349869898683,-0.00826292637260597,
-1.79006544278199));
#27477=CARTESIAN_POINT('Ctrl Pts',(100.349869898683,0.0347219594181997,
-1.79419129823274));
#27478=CARTESIAN_POINT('Ctrl Pts',(100.349869898683,0.0995747997289625,
-1.80041612446574));
#27479=CARTESIAN_POINT('Ctrl Pts',(100.349869898683,0.164664857862777,-1.80272216545712));
#27480=CARTESIAN_POINT('Ctrl Pts',(100.349869898683,0.229725300885458,-1.80133298954638));
#27481=CARTESIAN_POINT('Ctrl Pts',(100.349869898683,0.296581023837173,-1.79990548067148));
#27482=CARTESIAN_POINT('Ctrl Pts',(100.349869898682,0.363406212846286,-1.79457604187679));
#27483=CARTESIAN_POINT('Ctrl Pts',(100.349869898682,0.429927457817056,-1.78553511431891));
#27484=CARTESIAN_POINT('Ctrl Pts',(100.349869898682,0.46188858927035,-1.78119126485752));
#27485=CARTESIAN_POINT('Ctrl Pts',(100.349869898682,0.49377972082037,-1.7759898677578));
#27486=CARTESIAN_POINT('Ctrl Pts',(100.349869898682,0.525570989729067,-1.76994792489354));
#27487=CARTESIAN_POINT('Ctrl Pts',(100.349869898682,0.544239449495205,-1.76639997694611));
#27488=CARTESIAN_POINT('Ctrl Pts',(100.349869898682,0.562873475889264,-1.76256213670098));
#27489=CARTESIAN_POINT('Ctrl Pts',(100.349869898682,0.581467005198649,-1.75843743329571));
#27490=CARTESIAN_POINT('Ctrl Pts',(100.349869898682,0.596154585183419,-1.75517920780392));
#27491=CARTESIAN_POINT('Ctrl Pts',(100.349869898682,0.610820358907282,-1.75174098890037));
#27492=CARTESIAN_POINT('Ctrl Pts',(100.349869898682,0.625435174434094,-1.74813099328831));
#27493=CARTESIAN_POINT('Ctrl Pts',(100.349869898682,0.693327091226846,-1.73136105724182));
#27494=CARTESIAN_POINT('Ctrl Pts',(100.349869898682,0.760228106371345,-1.71086602232306));
#27495=CARTESIAN_POINT('Ctrl Pts',(100.349869898682,0.825842051564602,-1.68688364802346));
#27496=CARTESIAN_POINT('Ctrl Pts',(100.349869898682,0.892658275793112,-1.66246183199006));
#27497=CARTESIAN_POINT('Ctrl Pts',(100.349869898682,0.958140785980623,-1.63442357221684));
#27498=CARTESIAN_POINT('Ctrl Pts',(100.349869898682,1.02198275116856,-1.60296574252318));
#27499=CARTESIAN_POINT('Ctrl Pts',(100.349869898682,1.08621375452109,-1.57131621609384));
#27500=CARTESIAN_POINT('Ctrl Pts',(100.349869898682,1.1487852181858,-1.53620505098691));
#27501=CARTESIAN_POINT('Ctrl Pts',(100.349869898682,1.20937529811015,-1.49778156541698));
#27502=CARTESIAN_POINT('Ctrl Pts',(100.349869898682,1.22829221885182,-1.48578531071566));
#27503=CARTESIAN_POINT('Ctrl Pts',(100.349869898682,1.24701586973985,-1.47346582697558));
#27504=CARTESIAN_POINT('Ctrl Pts',(100.349869898682,1.26553601308475,-1.46082671008806));
#27505=CARTESIAN_POINT('Ctrl Pts',(100.349869898682,1.27472938384671,-1.45455267184294));
#27506=CARTESIAN_POINT('Ctrl Pts',(100.349869898682,1.28386964618851,-1.44820182666929));
#27507=CARTESIAN_POINT('Ctrl Pts',(100.349869898682,1.29294880238582,-1.44177972141044));
#27508=CARTESIAN_POINT('Ctrl Pts',(100.349869898682,1.35324423932221,-1.39912998235782));
#27509=CARTESIAN_POINT('Ctrl Pts',(100.349869898682,1.41093556061047,-1.35328021416844));
#27510=CARTESIAN_POINT('Ctrl Pts',(100.349869898682,1.4657028486192,-1.30444825214604));
#27511=CARTESIAN_POINT('Ctrl Pts',(100.349869898682,1.52027452528291,-1.25579070237076));
#27512=CARTESIAN_POINT('Ctrl Pts',(100.349869898682,1.57194408047454,-1.20417182309451));
#27513=CARTESIAN_POINT('Ctrl Pts',(100.349869898682,1.62038013382389,-1.14975844237987));
#27514=CARTESIAN_POINT('Ctrl Pts',(100.349869898682,1.64885755147716,-1.11776672419916));
#27515=CARTESIAN_POINT('Ctrl Pts',(100.349869898682,1.67621688120137,-1.08480813775943));
#27516=CARTESIAN_POINT('Ctrl Pts',(100.349869898682,1.70238609206081,-1.05090953536274));
#27517=CARTESIAN_POINT('Ctrl Pts',(100.349869898682,1.73605338905434,-1.00729819680594));
#27518=CARTESIAN_POINT('Ctrl Pts',(100.349869898682,1.76775143347145,-0.962131310211133));
#27519=CARTESIAN_POINT('Ctrl Pts',(100.349869898682,1.79747650045091,-0.915546859126332));
#27520=CARTESIAN_POINT('Ctrl Pts',(100.349869898682,1.80400780711809,-0.905311143386221));
#27521=CARTESIAN_POINT('Ctrl Pts',(100.349869898682,1.81043884326659,-0.895014695114994));
#27522=CARTESIAN_POINT('Ctrl Pts',(100.349869898682,1.81676859411663,-0.88466146049614));
#27523=CARTESIAN_POINT('Ctrl Pts',(100.349869898683,1.85447403403412,-0.822988690884629));
#27524=CARTESIAN_POINT('Ctrl Pts',(100.349869898683,1.88860369126805,-0.759280016585824));
#27525=CARTESIAN_POINT('Ctrl Pts',(100.349869898683,1.91920882291116,-0.69389751131988));
#27526=CARTESIAN_POINT('Ctrl Pts',(100.349869898683,1.95083266173162,-0.626338716529564));
#27527=CARTESIAN_POINT('Ctrl Pts',(100.349869898683,1.97869389269075,-0.556992193784614));
#27528=CARTESIAN_POINT('Ctrl Pts',(100.349869898683,2.0028101728334,-0.486216002267792));
#27529=CARTESIAN_POINT('Ctrl Pts',(100.349869898683,2.02692645297605,-0.41543981075097));
#27530=CARTESIAN_POINT('Ctrl Pts',(100.349869898683,2.04729804958241,-0.343233053659112));
#27531=CARTESIAN_POINT('Ctrl Pts',(100.349869898683,2.063899203451,-0.269924895638601));
#27532=CARTESIAN_POINT('Ctrl Pts',(100.349869898683,2.06724025486579,-0.255171323265941));
#27533=CARTESIAN_POINT('Ctrl Pts',(100.349869898683,2.07042844291423,-0.240373072421456));
#27534=CARTESIAN_POINT('Ctrl Pts',(100.349869898683,2.07346332984018,-0.225532735420184));
#27535=CARTESIAN_POINT('Ctrl Pts',(100.349869898683,2.07629732325745,-0.211674750461333));
#27536=CARTESIAN_POINT('Ctrl Pts',(100.349869898683,2.07899763861497,-0.197780066263633));
#27537=CARTESIAN_POINT('Ctrl Pts',(100.349869898683,2.08156385697044,-0.183850777551013));
#27538=CARTESIAN_POINT('Ctrl Pts',(100.349869898683,2.08418234040355,-0.169637796940397));
#27539=CARTESIAN_POINT('Ctrl Pts',(100.349869898683,2.08665986231528,-0.155395799266699));
#27540=CARTESIAN_POINT('Ctrl Pts',(100.349869898683,2.08899516018126,-0.141135229261509));
#27541=CARTESIAN_POINT('Ctrl Pts',(100.349869898683,2.10161552092171,-0.0640685987247987));
#27542=CARTESIAN_POINT('Ctrl Pts',(100.349869898683,2.11009928121374,0.0136100998382424));
#27543=CARTESIAN_POINT('Ctrl Pts',(100.349869898683,2.11445263267422,0.0915223436362172));
#27544=CARTESIAN_POINT('Ctrl Pts',(100.349869898683,2.11878556589602,0.169069160749906));
#27545=CARTESIAN_POINT('Ctrl Pts',(100.349869898683,2.1190269676162,0.246848345957318));
#27546=CARTESIAN_POINT('Ctrl Pts',(100.349869898682,2.11513535441828,0.324505766001828));
#27547=CARTESIAN_POINT('Ctrl Pts',(100.349869898682,2.11414398385978,0.344288636489222));
#27548=CARTESIAN_POINT('Ctrl Pts',(100.349869898682,2.11288414907951,0.364063658710047));
#27549=CARTESIAN_POINT('Ctrl Pts',(100.349869898682,2.11135463994554,0.383825055241067));
#27550=CARTESIAN_POINT('Ctrl Pts',(100.349869898682,2.11020352169258,0.398697607320445));
#27551=CARTESIAN_POINT('Ctrl Pts',(100.349869898682,2.10890040119927,0.41355265810877));
#27552=CARTESIAN_POINT('Ctrl Pts',(100.349869898682,2.10744539990257,0.428386817866786));
#27553=CARTESIAN_POINT('Ctrl Pts',(100.349869898682,2.09968291124935,0.507527638608771));
#27554=CARTESIAN_POINT('Ctrl Pts',(100.349869898682,2.08760086541998,0.586080887221537));
#27555=CARTESIAN_POINT('Ctrl Pts',(100.349869898682,2.07117840522959,0.663672733754418));
#27556=CARTESIAN_POINT('Ctrl Pts',(100.349869898682,2.05490267436401,0.740571322448959));
#27557=CARTESIAN_POINT('Ctrl Pts',(100.349869898682,2.03436391310342,0.816526640045261));
#27558=CARTESIAN_POINT('Ctrl Pts',(100.349869898682,2.00949149356056,0.891179159993276));
#27559=CARTESIAN_POINT('Ctrl Pts',(100.349869898682,2.00307587526026,0.910435110236372));
#27560=CARTESIAN_POINT('Ctrl Pts',(100.349869898682,1.99637165302191,0.929604358635672));
#27561=CARTESIAN_POINT('Ctrl Pts',(100.349869898682,1.98937704260631,0.948680653513866));
#27562=CARTESIAN_POINT('Ctrl Pts',(100.349869898682,-0.11727379276914,-1.77237437355361));
#27563=CARTESIAN_POINT('Ctrl Pts',(100.350147572039,-0.109438590926001,
-1.77289281020614));
#27564=CARTESIAN_POINT('Ctrl Pts',(100.350425245396,-0.101599951227993,
-1.77335929004107));
#27565=CARTESIAN_POINT('Ctrl Pts',(100.350702918754,-0.0937585630115176,
-1.77377377203577));
#27566=CARTESIAN_POINT('Origin',(100.349869898682,0.,0.));
#27567=CARTESIAN_POINT('Origin',(33.1926516271063,0.,0.));
#27568=CARTESIAN_POINT('',(33.4926516271063,-5.13007994755883E-16,4.18902817623056));
#27569=CARTESIAN_POINT('Origin',(33.4926516271063,0.,0.));
#27570=CARTESIAN_POINT('',(33.1926516271063,-5.49747398730303E-16,4.48902817623056));
#27571=CARTESIAN_POINT('Origin',(33.1926516271063,-5.13007994755883E-16,
4.18902817623056));
#27572=CARTESIAN_POINT('Origin',(33.1926516271063,0.,0.));
#27573=CARTESIAN_POINT('Origin',(32.5726008112287,0.,0.));
#27574=CARTESIAN_POINT('',(31.6525499953511,-5.49747398730303E-16,4.48902817623056));
#27575=CARTESIAN_POINT('',(32.5726008112287,-5.49747398730304E-16,4.48902817623056));
#27576=CARTESIAN_POINT('Origin',(31.6525499953511,0.,0.));
#27577=CARTESIAN_POINT('Origin',(33.4926516271063,0.,-2.21164758166987));
#27578=CARTESIAN_POINT('Origin',(31.3525499953512,0.,0.));
#27579=CARTESIAN_POINT('',(31.6525499953511,-7.4821050118432E-16,6.1096023907077));
#27580=CARTESIAN_POINT('Origin',(31.6525499953511,0.,0.));
#27581=CARTESIAN_POINT('',(31.3524613125654,-7.84949903553507E-16,6.40960237759997));
#27582=CARTESIAN_POINT('Origin',(31.3525499953512,-7.4821050118432E-16,
6.1096023907077));
#27583=CARTESIAN_POINT('Origin',(31.3524613125654,-7.84949903553507E-16,
0.));
#27584=CARTESIAN_POINT('Origin',(31.0318089645314,0.,0.));
#27585=CARTESIAN_POINT('',(30.7109792509259,-7.84926680813535E-16,6.40941274953751));
#27586=CARTESIAN_POINT('',(31.0318089645314,-7.84938295393988E-16,6.40950758978419));
#27587=CARTESIAN_POINT('Origin',(30.7109792509259,-7.84926680813535E-16,
0.));
#27588=CARTESIAN_POINT('Origin',(31.6525499953511,0.,-4.48902817623056));
#27589=CARTESIAN_POINT('Origin',(30.7110679337117,0.,0.));
#27590=CARTESIAN_POINT('',(30.4110679337117,-7.48187278444348E-16,6.10941276264524));
#27591=CARTESIAN_POINT('Origin',(30.7110679337117,-7.48187278444348E-16,
6.10941276264524));
#27592=CARTESIAN_POINT('Origin',(30.4110679337117,0.,0.));
#27593=CARTESIAN_POINT('Origin',(30.4110679337117,0.,-6.40932409296331));
#27594=CARTESIAN_POINT('',(30.4110679337117,-2.70848713173399E-16,2.21164758166987));
#27595=CARTESIAN_POINT('Origin',(30.4110679337117,0.,0.));
#27596=CARTESIAN_POINT('Origin',(28.3729800631879,0.,0.));
#27597=CARTESIAN_POINT('',(28.6729800631879,-7.48102635692981E-16,6.1087216021292));
#27598=CARTESIAN_POINT('Origin',(28.6729800631879,0.,0.));
#27599=CARTESIAN_POINT('',(28.3728913804021,-7.84842038062168E-16,6.40872158902147));
#27600=CARTESIAN_POINT('Origin',(28.3729800631879,-7.48102635692982E-16,
6.1087216021292));
#27601=CARTESIAN_POINT('Origin',(28.3728913804021,-7.84842038062168E-16,
0.));
#27602=CARTESIAN_POINT('Origin',(28.2136282688352,0.,0.));
#27603=CARTESIAN_POINT('',(28.0541877916966,-7.84830500451046E-16,6.40862737727707));
#27604=CARTESIAN_POINT('',(28.2136282688352,-7.84836272467075E-16,6.40867450936473));
#27605=CARTESIAN_POINT('Origin',(28.0541877916966,-7.84830500451046E-16,
0.));
#27606=CARTESIAN_POINT('Origin',(28.6729800631879,0.,0.));
#27607=CARTESIAN_POINT('',(28.6729800631879,-2.70848713173399E-16,2.21164758166987));
#27608=CARTESIAN_POINT('Origin',(28.6729800631879,0.,0.));
#27609=CARTESIAN_POINT('Origin',(28.0542764744824,0.,0.));
#27610=CARTESIAN_POINT('Origin',(28.0542764744824,-7.4809109808186E-16,
6.1086273903848));
#27611=CARTESIAN_POINT('Origin',(25.1947388265965,0.,0.));
#27612=CARTESIAN_POINT('',(25.1946501438108,-7.84726980332233E-16,6.40778207135796));
#27613=CARTESIAN_POINT('Origin',(25.1947388265965,-7.47987577963046E-16,
6.10778208446569));
#27614=CARTESIAN_POINT('Origin',(25.1946501438108,-7.84726980332233E-16,
0.));
#27615=CARTESIAN_POINT('Origin',(25.0105689136245,0.,0.));
#27616=CARTESIAN_POINT('',(24.8263103178667,-7.84713645805033E-16,6.40767318668028));
#27617=CARTESIAN_POINT('',(25.0105689136245,-7.847203162791E-16,6.40772765523458));
#27618=CARTESIAN_POINT('Origin',(24.8263103178667,-7.84713645805033E-16,
0.));
#27619=CARTESIAN_POINT('Origin',(24.8263990006525,0.,0.));
#27620=CARTESIAN_POINT('',(24.5263990006525,-7.47974243435846E-16,6.10767319978801));
#27621=CARTESIAN_POINT('Origin',(24.8263990006525,-7.47974243435846E-16,
6.10767319978801));
#27622=CARTESIAN_POINT('Origin',(24.5263990006525,0.,0.));
#27623=CARTESIAN_POINT('Origin',(24.5263990006525,0.,-6.40758453010608));
#27624=CARTESIAN_POINT('',(24.5263990006525,-2.70848713173399E-16,2.21164758166987));
#27625=CARTESIAN_POINT('Origin',(24.5263990006525,0.,0.));
#27626=CARTESIAN_POINT('Origin',(22.4730782633311,0.,0.));
#27627=CARTESIAN_POINT('',(22.7730782633312,-7.47889049228833E-16,6.1069775362949));
#27628=CARTESIAN_POINT('Origin',(22.7730782633312,0.,0.));
#27629=CARTESIAN_POINT('',(22.4729895805454,-7.8462845159802E-16,6.40697752318717));
#27630=CARTESIAN_POINT('Origin',(22.4730782633311,-7.47889049228834E-16,
6.1069775362949));
#27631=CARTESIAN_POINT('Origin',(22.4729895805454,-7.8462845159802E-16,
0.));
#27632=CARTESIAN_POINT('Origin',(22.2310089528171,0.,0.));
#27633=CARTESIAN_POINT('',(21.9888509595172,-7.84610924957793E-16,6.40683440730886));
#27634=CARTESIAN_POINT('',(22.2310089528171,-7.84619691488374E-16,6.40690599146347));
#27635=CARTESIAN_POINT('Origin',(21.9888509595172,-7.84610924957793E-16,
0.));
#27636=CARTESIAN_POINT('Origin',(22.7730782633312,0.,-2.21164758166987));
#27637=CARTESIAN_POINT('',(22.7730782633312,-2.70848713173399E-16,2.21164758166987));
#27638=CARTESIAN_POINT('Origin',(22.7730782633312,0.,0.));
#27639=CARTESIAN_POINT('Origin',(21.9889396423029,0.,0.));
#27640=CARTESIAN_POINT('',(21.688939642303,-7.47871522588606E-16,6.10683442041659));
#27641=CARTESIAN_POINT('Origin',(21.9889396423029,-7.47871522588606E-16,
6.10683442041659));
#27642=CARTESIAN_POINT('Origin',(21.688939642303,0.,0.));
#27643=CARTESIAN_POINT('Origin',(21.688939642303,0.,-6.40674575073467));
#27644=CARTESIAN_POINT('',(21.688939642303,-5.41697426346798E-16,4.42329516333974));
#27645=CARTESIAN_POINT('Origin',(21.688939642303,0.,0.));
#27646=CARTESIAN_POINT('Origin',(21.1989257366328,0.,0.));
#27647=CARTESIAN_POINT('',(21.1989257366328,-5.41697426346798E-16,4.42329516333974));
#27648=CARTESIAN_POINT('Origin',(21.1989257366328,0.,0.));
#27649=CARTESIAN_POINT('',(20.8989257366328,-5.04958022372377E-16,4.12329516333974));
#27650=CARTESIAN_POINT('Origin',(21.1989257366328,-5.04958022372377E-16,
4.12329516333974));
#27651=CARTESIAN_POINT('Origin',(20.8989257366328,0.,0.));
#27652=CARTESIAN_POINT('Origin',(20.8989257366328,0.,-4.42329516333974));
#27653=CARTESIAN_POINT('Origin',(21.2939326894679,0.,0.));
#27654=CARTESIAN_POINT('',(21.2939326894679,-5.41697426346798E-16,4.42329516333974));
#27655=CARTESIAN_POINT('Origin',(23.6497386319918,0.,0.));
#27656=CARTESIAN_POINT('',(23.6497386319918,-2.70848713173399E-16,2.21164758166987));
#27657=CARTESIAN_POINT('Origin',(29.5420239984498,0.,0.));
#27658=CARTESIAN_POINT('',(29.5420239984498,-2.70848713173399E-16,2.21164758166987));
#27693=UNCERTAINTY_MEASURE_WITH_UNIT(LENGTH_MEASURE(0.01),#27708,
'DISTANCE_ACCURACY_VALUE',
'Maximum model space distance between geometric entities at asserted c
onnectivities');
#27695=UNCERTAINTY_MEASURE_WITH_UNIT(LENGTH_MEASURE(0.01),#27708,
'DISTANCE_ACCURACY_VALUE',
'Maximum model space distance between geometric entities at asserted c
onnectivities');
#27705=(
GEOMETRIC_REPRESENTATION_CONTEXT(3)
GLOBAL_UNCERTAINTY_ASSIGNED_CONTEXT((#27693))
GLOBAL_UNIT_ASSIGNED_CONTEXT((#27708,#27710,#27711))
REPRESENTATION_CONTEXT('','3D')
);
#27707=(
GEOMETRIC_REPRESENTATION_CONTEXT(3)
GLOBAL_UNCERTAINTY_ASSIGNED_CONTEXT((#27695))
GLOBAL_UNIT_ASSIGNED_CONTEXT((#27708,#27710,#27711))
REPRESENTATION_CONTEXT('','3D')
);
#27708=(
LENGTH_UNIT()
NAMED_UNIT(*)
SI_UNIT(.MILLI.,.METRE.)
);
#27710=(
NAMED_UNIT(*)
PLANE_ANGLE_UNIT()
SI_UNIT($,.RADIAN.)
);
#27711=(
NAMED_UNIT(*)
SI_UNIT($,.STERADIAN.)
SOLID_ANGLE_UNIT()
);
#27721=SHAPE_DEFINITION_REPRESENTATION(#27732,#27753);
#27732=PRODUCT_DEFINITION_SHAPE('',$,#27765);
#27753=SHAPE_REPRESENTATION('',(#4156),#27705);
#27755=PRODUCT_DEFINITION_CONTEXT('part definition',#27790,'design');
#27765=PRODUCT_DEFINITION('Shaft','Shaft',#27776,#27755);
#27776=PRODUCT_DEFINITION_FORMATION('',$,#27801);
#27790=APPLICATION_CONTEXT(
'Core Data for Automotive Mechanical Design Process');
#27791=PRODUCT_CONTEXT('part definition',#27790,'mechanical');
#27801=PRODUCT('Shaft','Shaft',$,(#27791));
#27804=PRESENTATION_STYLE_ASSIGNMENT((#27806));
#27806=SURFACE_STYLE_USAGE(.BOTH.,#27808);
#27808=SURFACE_SIDE_STYLE('',(#27810));
#27810=SURFACE_STYLE_FILL_AREA(#27812);
#27812=FILL_AREA_STYLE('Opaque(160,160,160)',(#27814));
#27814=FILL_AREA_STYLE_COLOUR('Opaque(160,160,160)',#27816);
#27816=COLOUR_RGB('Opaque(160,160,160)', 0.09019608, 0.27058824, 0.51372549);
ENDSEC;
END-ISO-10303-21;
